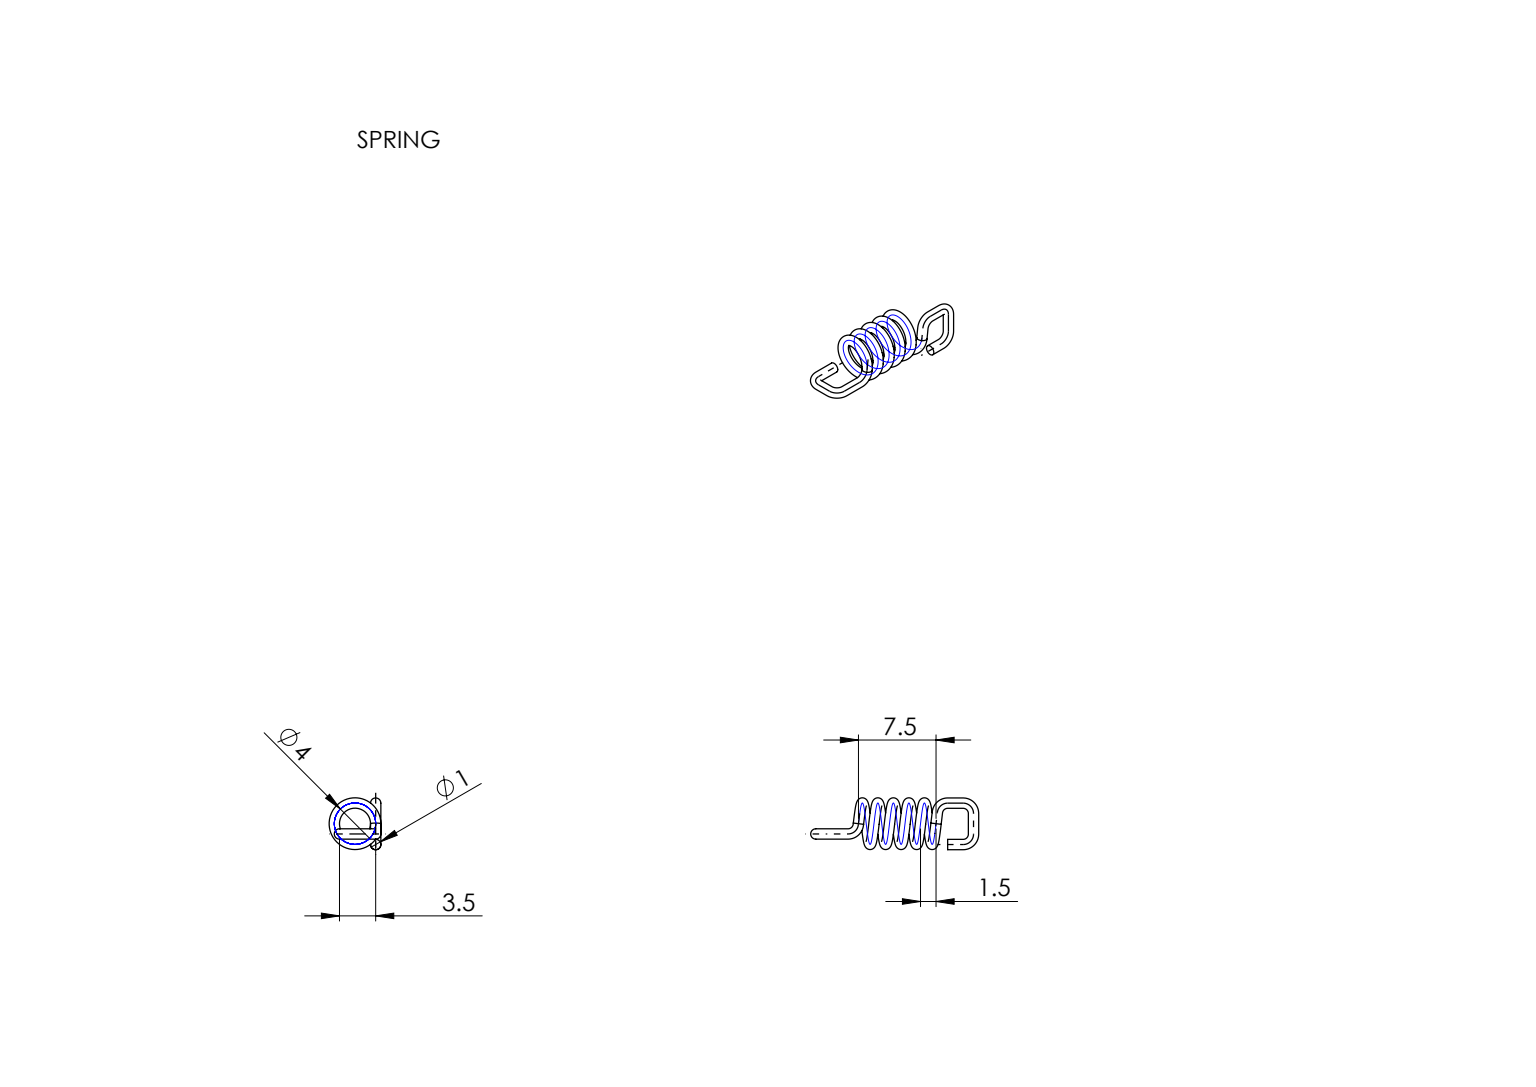
ISO-10303-21;
HEADER;
FILE_DESCRIPTION (('STEP AP214'),
    '1' );
FILE_NAME ('spring.step',
    '2026-09-28T15:49:00',
    ( '' ),
    ( '' ),
    'SwSTEP 2.0',
    'SolidWorks 2026',
    '' );
FILE_SCHEMA (( 'AUTOMOTIVE_DESIGN' ));
ENDSEC;

DATA;
#5=CARTESIAN_POINT ( 'NONE',  ( -34.00000000000000000, -114.0592624029313242, 6.003524454178450043 ) ) ;
#16=CARTESIAN_POINT ( 'NONE',  ( -35.50000000000000000, -112.5389594332240222, 2.818899826424027477 ) ) ;
#20=CARTESIAN_POINT ( 'NONE',  ( -35.50000000000000711, -114.9929510916434339, 11.38636890470581164 ) ) ;
#22=CARTESIAN_POINT ( 'NONE',  ( -34.50000000000000000, -113.9929510916434339, 12.17846912687782712 ) ) ;
#25=CARTESIAN_POINT ( 'NONE',  ( -34.50000000000000000, -113.9929510916434339, 10.68227981832981044 ) ) ;
#26=CARTESIAN_POINT ( 'NONE',  ( -38.99999693208653895, -114.9929510916434339, 12.62875129555797749 ) ) ;
#27=CARTESIAN_POINT ( 'NONE',  ( -35.50000000000000711, -114.9860996047076895, 10.38555023491505835 ) ) ;
#42=CARTESIAN_POINT ( 'NONE',  ( -35.50000000000000000, -113.2441867727860227, 0.9026824934337903672 ) ) ;
#44=CARTESIAN_POINT ( 'NONE',  ( -37.97545270896701908, -113.5265240346955977, 3.847274454178448710 ) ) ;
#51=CARTESIAN_POINT ( 'NONE',  ( -35.50000000000000000, -116.2431927316855109, -2.224114562372550008 ) ) ;
#54=CARTESIAN_POINT ( 'NONE',  ( -39.02454729103295961, -114.7691647218148745, 8.159774454178448266 ) ) ;
#59=CARTESIAN_POINT ( 'NONE',  ( -34.50000000000000000, -113.0140978167136581, -0.6247823525984268489 ) ) ;
#65=CARTESIAN_POINT ( 'NONE',  ( -35.50000000000000000, -113.9929510916434339, 10.61627146648203990 ) ) ;
#70=CARTESIAN_POINT ( 'NONE',  ( -34.50000000000000000, -113.0071371610607684, 2.888584676720006961 ) ) ;
#71=CARTESIAN_POINT ( 'NONE',  ( -39.00000000000000000, -115.9929510916434481, 12.17846912687782179 ) ) ;
#77=CARTESIAN_POINT ( 'NONE',  ( -35.50000000000000711, -114.1414532730574507, 9.517316564499758158 ) ) ;
#95=CARTESIAN_POINT ( 'NONE',  ( -36.64504884055821776, -112.9754527089670688, 6.715225545821551734 ) ) ;
#108=CARTESIAN_POINT ( 'NONE',  ( -35.50000000000000711, -114.0882517521923489, 9.510534276948430232 ) ) ;
#115=CARTESIAN_POINT ( 'NONE',  ( -35.87745010033553683, -115.9929510916434481, 14.11371147303761475 ) ) ;
#124=CARTESIAN_POINT ( 'NONE',  ( -35.62769128460905677, -112.5438815906447729, 6.808975545821550845 ) ) ;
#149=CARTESIAN_POINT ( 'NONE',  ( -34.50000000000000000, -113.4307644833805000, -1.624782352598427959 ) ) ;
#151=CARTESIAN_POINT ( 'NONE',  ( -39.00000000000000711, -114.9929510916434339, 12.60752341388803721 ) ) ;
#152=CARTESIAN_POINT ( 'NONE',  ( -35.50000000000000000, -113.9929510916434339, 10.50625754673586876 ) ) ;
#155=CARTESIAN_POINT ( 'NONE',  ( -36.03125000000004263, -114.9929510916434339, 14.11852480586264846 ) ) ;
#167=CARTESIAN_POINT ( 'NONE',  ( -39.16322519054179452, -116.0794154965774823, 6.566024454178448266 ) ) ;
#174=CARTESIAN_POINT ( 'NONE',  ( -39.07941549657748936, -111.8367748094582055, 6.941024454178450043 ) ) ;
#177=DIRECTION ( 'NONE',  ( -1.000000000000000000, 0.000000000000000000, 0.000000000000000000 ) ) ;
#186=CARTESIAN_POINT ( 'NONE',  ( -35.50000000000000000, -111.8727710936879589, 2.535339294948415922 ) ) ;
#193=CARTESIAN_POINT ( 'NONE',  ( -35.50160444427493189, -114.9929510916434339, 12.65937477241749853 ) ) ;
#194=CARTESIAN_POINT ( 'NONE',  ( -36.03125000000003553, -113.9929510916434339, 14.11852480586265024 ) ) ;
#198=CARTESIAN_POINT ( 'NONE',  ( -34.50000000000000000, -113.9929510916434339, 10.50625754673588474 ) ) ;
#199=CARTESIAN_POINT ( 'NONE',  ( -39.00000000000000711, -114.9929510916434339, 11.21034663311206181 ) ) ;
#200=CARTESIAN_POINT ( 'NONE',  ( -35.50000000000000711, -114.9492820284331742, 10.20776876943783940 ) ) ;
#202=CIRCLE ( 'NONE', #8824, 0.5000000000000004441 ) ;
#213=CARTESIAN_POINT ( 'NONE',  ( -35.50000000000000000, -113.0140978167138712, 0.8127176474015720409 ) ) ;
#215=CARTESIAN_POINT ( 'NONE',  ( -36.11231047232249125, -112.0245472910329880, 5.722274454178448266 ) ) ;
#221=CARTESIAN_POINT ( 'NONE',  ( -35.50000000000000711, -112.8356783780338759, 1.859636627348750348 ) ) ;
#224=CARTESIAN_POINT ( 'NONE',  ( -38.97545270896704039, -113.1123104723225197, 8.347274454178448266 ) ) ;
#228=CARTESIAN_POINT ( 'NONE',  ( -34.50000000000000000, -113.6318576702834804, 1.956056246348823580 ) ) ;
#235=CARTESIAN_POINT ( 'NONE',  ( -35.50000000000000000, -113.9929510916434339, 11.38636890470581164 ) ) ;
#240=CARTESIAN_POINT ( 'NONE',  ( -34.50000000000000000, -111.1014359431343905, 1.472195201997948510 ) ) ;
#242=CARTESIAN_POINT ( 'NONE',  ( -37.51022648969539119, -115.9929510916434481, 14.11852173794918563 ) ) ;
#247=CARTESIAN_POINT ( 'NONE',  ( -37.99999897736217491, -115.9929510916434481, 12.62466071271733092 ) ) ;
#267=CARTESIAN_POINT ( 'NONE',  ( -37.74901162816868805, -113.3347980657955958, 4.933975545821551734 ) ) ;
#276=CARTESIAN_POINT ( 'NONE',  ( -35.50000000000000000, -117.0140978167138854, 0.6252176474015650465 ) ) ;
#287=CARTESIAN_POINT ( 'NONE',  ( -38.81062062679291813, -115.9929510916434481, 13.37409560816442244 ) ) ;
#296=CARTESIAN_POINT ( 'NONE',  ( -37.88768952767750875, -112.0245472910329880, 9.527725545821557063 ) ) ;
#324=CARTESIAN_POINT ( 'NONE',  ( -34.50000000000000000, -115.0795240838853886, -1.623175561345890472 ) ) ;
#325=CARTESIAN_POINT ( 'NONE',  ( -38.99999693208653895, -114.9929510916434339, 12.62875129555797749 ) ) ;
#326=CARTESIAN_POINT ( 'NONE',  ( -35.50000000000000000, -113.9929510916433060, 10.50625754673589540 ) ) ;
#328=CARTESIAN_POINT ( 'NONE',  ( -34.50481333282507279, -114.9929510916434339, 12.74107470552716492 ) ) ;
#337=CARTESIAN_POINT ( 'NONE',  ( -33.97545270896702618, -112.8166217158120475, 5.909774454178450931 ) ) ;
#341=CARTESIAN_POINT ( 'NONE',  ( -35.50000000000000711, -115.6286452741999113, -1.424448457485488095 ) ) ;
#358=CARTESIAN_POINT ( 'NONE',  ( -35.50000000000000000, -112.3070160848889429, 2.749963775944984867 ) ) ;
#361=CARTESIAN_POINT ( 'NONE',  ( -35.83891589277640577, -114.9929510916434339, 13.09299768411358222 ) ) ;
#365=CARTESIAN_POINT ( 'NONE',  ( -34.50000000000000000, -113.9929510916434339, 12.56351784598954424 ) ) ;
#368=CARTESIAN_POINT ( 'NONE',  ( -34.50000000000000000, -113.9929510916434339, 11.21034663311132107 ) ) ;
#371=CARTESIAN_POINT ( 'NONE',  ( -35.50000000000000711, -114.8211182053456838, 9.932864235516914775 ) ) ;
#385=CARTESIAN_POINT ( 'NONE',  ( -35.50000000000000000, -114.5974311500472567, -0.6247823525984269599 ) ) ;
#387=CARTESIAN_POINT ( 'NONE',  ( -39.02454729103295961, -114.7691647218148745, 5.159774454178448266 ) ) ;
#394=CARTESIAN_POINT ( 'NONE',  ( -35.50000000000000711, -112.0140900043112282, 0.8439677466545482121 ) ) ;
#399=CARTESIAN_POINT ( 'NONE',  ( -35.00000000000000000, -114.0592624029313242, 9.003524454178448266 ) ) ;
#401=( NAMED_UNIT ( * ) PLANE_ANGLE_UNIT ( ) SI_UNIT ( $, .RADIAN. ) );
#405=CARTESIAN_POINT ( 'NONE',  ( -34.50000000000000000, -112.7472371723319355, 1.839427296857320648 ) ) ;
#410=CIRCLE ( 'NONE', #8457, 0.5000000000000004441 ) ;
#412=CARTESIAN_POINT ( 'NONE',  ( -35.50000000000000000, -113.9929510916434339, 11.91443571948720148 ) ) ;
#415=CARTESIAN_POINT ( 'NONE',  ( -34.50000000000000000, -115.9821387493194891, -0.8839717462762166633 ) ) ;
#419=CARTESIAN_POINT ( 'NONE',  ( -39.00000206272865455, -115.9929510916434481, 12.61164896875035879 ) ) ;
#446=CARTESIAN_POINT ( 'NONE',  ( -37.05926240293131713, -113.0000000000000000, 3.621475545821551734 ) ) ;
#458=CARTESIAN_POINT ( 'NONE',  ( -35.50000000000000711, -115.6286452741999113, -1.424448457485488095 ) ) ;
#460=CARTESIAN_POINT ( 'NONE',  ( -35.50000000000000711, -114.1264797827112574, 9.515205387299289441 ) ) ;
#464=CARTESIAN_POINT ( 'NONE',  ( -34.50000000000000000, -114.9819937217110635, 10.35556074009299188 ) ) ;
#468=CARTESIAN_POINT ( 'NONE',  ( -36.24999999999983658, -115.9929510916434481, 14.11852480586265024 ) ) ;
#469=CARTESIAN_POINT ( 'NONE',  ( -35.50000000000000711, -112.0140900043366088, -0.5935324770972457697 ) ) ;
#480=CARTESIAN_POINT ( 'NONE',  ( -36.11231047232249125, -115.9754527089670262, 7.277725545821551734 ) ) ;
#507=CARTESIAN_POINT ( 'NONE',  ( -34.50000000000000000, -113.3474311500483935, -0.6247823525984269599 ) ) ;
#510=CARTESIAN_POINT ( 'NONE',  ( -39.00000000000000711, -114.9929510916434339, 11.91443571948719615 ) ) ;
#514=CARTESIAN_POINT ( 'NONE',  ( -34.50000000000000000, -114.9929510916434339, 12.59652202191340642 ) ) ;
#523=CARTESIAN_POINT ( 'NONE',  ( -39.16322519054179452, -116.0794154965774823, 3.566024454178448710 ) ) ;
#526=CARTESIAN_POINT ( 'NONE',  ( -35.50000000000000711, -112.1403507321855528, -1.128496220798856253 ) ) ;
#541=CARTESIAN_POINT ( 'NONE',  ( -35.50000000000000000, -112.9611193698460738, 2.883091707513499635 ) ) ;
#543=CARTESIAN_POINT ( 'NONE',  ( -35.50025087934803736, -114.9929510916434339, 12.63488142334835196 ) ) ;
#547=CARTESIAN_POINT ( 'NONE',  ( -38.98797722933581866, -113.9929510916434339, 12.81430620224974959 ) ) ;
#551=CARTESIAN_POINT ( 'NONE',  ( -34.50300906734826611, -113.9929510916434339, 12.71660600561482468 ) ) ;
#552=CARTESIAN_POINT ( 'NONE',  ( -38.98797722933582577, -114.9929510916434339, 12.81430620224974959 ) ) ;
#553=CARTESIAN_POINT ( 'NONE',  ( -35.50000000000000711, -114.9929510916434339, 10.51175824272318415 ) ) ;
#563=CARTESIAN_POINT ( 'NONE',  ( -35.50000000000000000, -113.0140978167138712, -0.6247823525979733228 ) ) ;
#565=CARTESIAN_POINT ( 'NONE',  ( -35.62769128460905677, -115.4561184093552413, 4.691024454178448266 ) ) ;
#572=CARTESIAN_POINT ( 'NONE',  ( -35.50000000000000711, -112.6605569508015350, 1.812590711673265575 ) ) ;
#575=CARTESIAN_POINT ( 'NONE',  ( -38.37230871539094323, -112.5438815906447729, 5.441024454178449155 ) ) ;
#582=CARTESIAN_POINT ( 'NONE',  ( -34.50000000000000000, -113.0106174888879877, 1.881901162060937827 ) ) ;
#588=CARTESIAN_POINT ( 'NONE',  ( -35.50000000000000000, -113.9929510916434339, 10.50625754673577994 ) ) ;
#592=CARTESIAN_POINT ( 'NONE',  ( -34.50000000000000000, -112.7319952733504635, 2.855726801009121463 ) ) ;
#593=CARTESIAN_POINT ( 'NONE',  ( -37.74437085908086686, -115.9929510916434481, 14.09929883582536903 ) ) ;
#617=CARTESIAN_POINT ( 'NONE',  ( -36.52652403469559061, -114.9754527089670262, 5.777725545821551734 ) ) ;
#629=CARTESIAN_POINT ( 'NONE',  ( -35.50000000000000711, -114.9928438774171582, 10.49113435197128652 ) ) ;
#633=CARTESIAN_POINT ( 'NONE',  ( -34.50000000000000000, -114.9929510916434339, 10.85830208992344303 ) ) ;
#638=CARTESIAN_POINT ( 'NONE',  ( -39.00000000000000000, -115.9929510916434481, 11.73841344789285657 ) ) ;
#639=CARTESIAN_POINT ( 'NONE',  ( -35.50000000000000711, -112.2144317118258527, -1.239329810084414341 ) ) ;
#647=CARTESIAN_POINT ( 'NONE',  ( -36.64504884055821776, -112.9754527089670688, 3.715225545821552178 ) ) ;
#672=CARTESIAN_POINT ( 'NONE',  ( -34.50000000000000000, -115.0140978167138712, -0.6247823525985405357 ) ) ;
#675=CARTESIAN_POINT ( 'NONE',  ( -39.00000000000000711, -114.9929510916434339, 12.39849696637031151 ) ) ;
#679=CARTESIAN_POINT ( 'NONE',  ( -34.50000000000000000, -114.2600084737790809, 8.524153227862690585 ) ) ;
#689=CARTESIAN_POINT ( 'NONE',  ( -38.30190309005061522, -116.9754527089670546, 7.972274454178450043 ) ) ;
#691=CARTESIAN_POINT ( 'NONE',  ( -35.50000000000000711, -112.9486715495423681, -1.623175561345890472 ) ) ;
#704=CARTESIAN_POINT ( 'NONE',  ( -36.23083527818513261, -111.9754527089670404, 5.215225545821551734 ) ) ;
#710=CARTESIAN_POINT ( 'NONE',  ( -35.50000000000000000, -112.4803765279500993, 2.803636946313094569 ) ) ;
#715=CARTESIAN_POINT ( 'NONE',  ( -37.37500000000009237, -114.9929510916434339, 13.11852480586264669 ) ) ;
#717=CARTESIAN_POINT ( 'NONE',  ( -37.54906985245723661, -113.9929510916434339, 14.11777216781844757 ) ) ;
#722=CARTESIAN_POINT ( 'NONE',  ( -36.12500000000014211, -113.9929510916434339, 14.11852480586265024 ) ) ;
#725=CARTESIAN_POINT ( 'NONE',  ( -35.50040135968785648, -114.9929510916434339, 12.63896776382214071 ) ) ;
#730=ORIENTED_EDGE ( 'NONE', *, *, #15666, .T. ) ;
#738=CARTESIAN_POINT ( 'NONE',  ( -35.50000000000000000, -115.0140978167134165, -0.6247823525984399495 ) ) ;
#740=CARTESIAN_POINT ( 'NONE',  ( -38.02454729103296671, -114.3549511594417396, 8.159774454178448266 ) ) ;
#742=CARTESIAN_POINT ( 'NONE',  ( -36.11231047232249125, -112.0245472910329880, 7.222274454178451819 ) ) ;
#748=CARTESIAN_POINT ( 'NONE',  ( -35.50000000000000000, -116.0215255531121983, -2.372276521655488857 ) ) ;
#752=CARTESIAN_POINT ( 'NONE',  ( -36.11231047232249125, -112.0245472910329880, 5.722274454178448266 ) ) ;
#757=CARTESIAN_POINT ( 'NONE',  ( -34.50000000000000000, -112.0414288467712112, 1.115164475686276191 ) ) ;
#766=CARTESIAN_POINT ( 'NONE',  ( -37.18750000000004974, -113.9929510916434339, 13.11852480586264846 ) ) ;
#769=CARTESIAN_POINT ( 'NONE',  ( -34.50000000000000000, -111.0140978167138570, 0.5627176474015715968 ) ) ;
#770=CARTESIAN_POINT ( 'NONE',  ( -39.00000000000000000, -115.9929510916434481, 12.57451923796417681 ) ) ;
#794=CARTESIAN_POINT ( 'NONE',  ( -36.52652403469559061, -114.9754527089670262, 7.277725545821552622 ) ) ;
#801=CARTESIAN_POINT ( 'NONE',  ( -35.50000000000000711, -115.2732872103912030, -1.592823285204062911 ) ) ;
#803=CARTESIAN_POINT ( 'NONE',  ( -35.50000000000000711, -114.9929510916434339, 12.59652202191340642 ) ) ;
#807=CARTESIAN_POINT ( 'NONE',  ( -34.50000000000000000, -114.9929510916434339, 10.55026311463432087 ) ) ;
#811=CARTESIAN_POINT ( 'NONE',  ( -39.00000000000000000, -115.9929510916434481, 12.26648026267477221 ) ) ;
#812=CARTESIAN_POINT ( 'NONE',  ( -35.50000000000000711, -112.0414288467712112, 1.115164475686276191 ) ) ;
#821=CARTESIAN_POINT ( 'NONE',  ( -36.64504884055823908, -115.0245472910329880, 1.784774454178449155 ) ) ;
#832=CARTESIAN_POINT ( 'NONE',  ( -37.05926240293131713, -111.0000000000000284, 5.121475545821551734 ) ) ;
#848=CARTESIAN_POINT ( 'NONE',  ( -34.50000000000000000, -115.0140978167139707, -0.6247823525984387283 ) ) ;
#852=CARTESIAN_POINT ( 'NONE',  ( -39.00000000000000711, -114.9929510916434339, 11.73841344789285657 ) ) ;
#854=CARTESIAN_POINT ( 'NONE',  ( -36.23083527818513261, -116.0245472910329880, 1.784774454178448710 ) ) ;
#855=CARTESIAN_POINT ( 'NONE',  ( -39.00000000000000711, -114.9929510916434339, 11.91443571948719615 ) ) ;
#858=DIRECTION ( 'NONE',  ( 0.000000000000000000, 0.000000000000000000, -1.000000000000000000 ) ) ;
#865=CARTESIAN_POINT ( 'NONE',  ( -35.81662171581203324, -110.9754527089670546, 3.715225545821552178 ) ) ;
#867=CARTESIAN_POINT ( 'NONE',  ( -35.50000000000000711, -112.8511839106603247, -1.611965039240275122 ) ) ;
#885=CARTESIAN_POINT ( 'NONE',  ( -39.02454729103295961, -113.2308352781851397, 6.340225545821550845 ) ) ;
#893=CARTESIAN_POINT ( 'NONE',  ( -35.50000000000000000, -113.2224311500466030, -2.624782352598442614 ) ) ;
#896=CARTESIAN_POINT ( 'NONE',  ( -35.74814306589956914, -114.9929510916434339, 13.05539834812772781 ) ) ;
#897=CARTESIAN_POINT ( 'NONE',  ( -39.00000206272865455, -113.9929510916434339, 12.61164896875035879 ) ) ;
#901=CARTESIAN_POINT ( 'NONE',  ( -35.80421860361284558, -113.9929510916434339, 14.10650203519841916 ) ) ;
#906=CARTESIAN_POINT ( 'NONE',  ( -35.96730626674924025, -114.9929510916434339, 13.11752178341330044 ) ) ;
#913=CARTESIAN_POINT ( 'NONE',  ( -35.74814306589956914, -114.9929510916434339, 13.05539834812772781 ) ) ;
#922=CARTESIAN_POINT ( 'NONE',  ( -35.50000000000000000, -113.0140978167156902, -0.6247823525984268489 ) ) ;
#924=CARTESIAN_POINT ( 'NONE',  ( -35.97545270896702618, -113.6450488405582604, 8.909774454178450043 ) ) ;
#928=CARTESIAN_POINT ( 'NONE',  ( -38.97545270896704039, -113.1123104723225197, 6.847274454178450931 ) ) ;
#931=CARTESIAN_POINT ( 'NONE',  ( -35.50000000000000711, -112.0221129971568104, -0.7553032835231431319 ) ) ;
#942=CARTESIAN_POINT ( 'NONE',  ( -34.50000000000000000, -112.9185811467682754, 1.870920967077121411 ) ) ;
#950=CARTESIAN_POINT ( 'NONE',  ( -35.93473953453761993, -113.9929510916434339, 13.11451721564123396 ) ) ;
#953=CARTESIAN_POINT ( 'NONE',  ( -35.69272627125608466, -113.9929510916434339, 13.01835785830562209 ) ) ;
#955=CARTESIAN_POINT ( 'NONE',  ( -35.50000000000000000, -115.9929510916434481, 10.94631322572069365 ) ) ;
#986=CARTESIAN_POINT ( 'NONE',  ( -37.74901162816868805, -113.3347980657955958, 9.433975545821549957 ) ) ;
#998=CARTESIAN_POINT ( 'NONE',  ( -35.95915003344517658, -114.9929510916434339, 13.11692036158763308 ) ) ;
#1003=CARTESIAN_POINT ( 'NONE',  ( -34.50000000000000000, -114.0998638248492085, 9.511920366020609308 ) ) ;
#1009=CARTESIAN_POINT ( 'NONE',  ( -35.50000000000000000, -115.9929081983957104, 10.49113315946066294 ) ) ;
#1010=CARTESIAN_POINT ( 'NONE',  ( -35.50000000000000711, -113.6318576702834804, 1.956056246348823580 ) ) ;
#1021=CARTESIAN_POINT ( 'NONE',  ( -37.66520193420439711, -114.7490116281687023, 6.058975545821550845 ) ) ;
#1031=CARTESIAN_POINT ( 'NONE',  ( -36.94073759706866156, -111.0000000000000284, 7.128524454178450043 ) ) ;
#1048=CARTESIAN_POINT ( 'NONE',  ( -34.50000000000000000, -115.0140978167138712, -0.4685323525984310122 ) ) ;
#1052=CARTESIAN_POINT ( 'NONE',  ( -34.50000000000000000, -114.3793648455349654, 8.543708532059524074 ) ) ;
#1055=CARTESIAN_POINT ( 'NONE',  ( -38.99879592093640923, -114.9929510916434339, 12.67985367974111455 ) ) ;
#1065=CARTESIAN_POINT ( 'NONE',  ( -39.16322519054178741, -111.9205845034225177, 3.433975545821550845 ) ) ;
#1067=CARTESIAN_POINT ( 'NONE',  ( -35.50000000000000711, -116.0140978167138712, -0.4685323525984310677 ) ) ;
#1079=CARTESIAN_POINT ( 'NONE',  ( -37.76916472181486739, -116.0245472910329880, 5.965225545821551734 ) ) ;
#1083=CARTESIAN_POINT ( 'NONE',  ( -35.50000000000000000, -114.8057644833805853, -2.624782352598442614 ) ) ;
#1088=CARTESIAN_POINT ( 'NONE',  ( -37.59808119975203766, -113.9929510916434339, 14.11551573851449071 ) ) ;
#1093=CARTESIAN_POINT ( 'NONE',  ( -37.46874999999995737, -113.9929510916434339, 14.11852480586265024 ) ) ;
#1095=CARTESIAN_POINT ( 'NONE',  ( -36.03906250000000000, -114.9929510916434339, 13.11852480586264669 ) ) ;
#1102=CARTESIAN_POINT ( 'NONE',  ( -35.50000000000000711, -114.9929510916434339, 11.38636890470581164 ) ) ;
#1105=CARTESIAN_POINT ( 'NONE',  ( -37.88768952767750164, -115.9754527089670262, 1.972274454178448710 ) ) ;
#1110=CARTESIAN_POINT ( 'NONE',  ( -35.50000000000000000, -113.0140978167138996, -0.6247823525984306237 ) ) ;
#1114=CARTESIAN_POINT ( 'NONE',  ( -37.88768952767750164, -115.9754527089670262, 1.972274454178448710 ) ) ;
#1116=CARTESIAN_POINT ( 'NONE',  ( -35.50000000000000711, -115.0795240838853886, -1.623175561345890472 ) ) ;
#1127=CARTESIAN_POINT ( 'NONE',  ( -34.50000000000000000, -116.0140978167138712, -0.4685323525984310677 ) ) ;
#1134=CARTESIAN_POINT ( 'NONE',  ( -37.50613590685470911, -113.9929510916434339, 13.11852378322482515 ) ) ;
#1139=CARTESIAN_POINT ( 'NONE',  ( -35.50000000000000000, -113.9929510916434339, 11.91443571948720148 ) ) ;
#1140=CARTESIAN_POINT ( 'NONE',  ( -35.50000000000000000, -115.9929510916434481, 10.72628538622835670 ) ) ;
#1158=CARTESIAN_POINT ( 'NONE',  ( -34.50000000000000000, -115.2751396785629510, -2.608751991713152307 ) ) ;
#1159=DIRECTION ( 'NONE',  ( -1.000000000000000000, 0.000000000000000000, 0.000000000000000000 ) ) ;
#1162=CARTESIAN_POINT ( 'NONE',  ( -37.99999999999998579, -113.9407375970686758, 3.753524454178448710 ) ) ;
#1168=CARTESIAN_POINT ( 'NONE',  ( -34.50000000000000000, -113.0140978167142833, 0.8752176474019800478 ) ) ;
#1174=CARTESIAN_POINT ( 'NONE',  ( -35.50400759022159036, -114.9929510916434339, 12.68378527132497524 ) ) ;
#1181=CARTESIAN_POINT ( 'NONE',  ( -34.50000000000000000, -114.9929510916434339, 10.94631322572069365 ) ) ;
#1186=CARTESIAN_POINT ( 'NONE',  ( -35.50000000000000000, -115.9874658933321001, 10.35517832894335832 ) ) ;
#1187=CARTESIAN_POINT ( 'NONE',  ( -35.50000000000000711, -112.1222502514821144, 1.343475657184566296 ) ) ;
#1196=CARTESIAN_POINT ( 'NONE',  ( -36.94073759706868287, -115.0000000000000000, 7.371475545821551734 ) ) ;
#1203=CARTESIAN_POINT ( 'NONE',  ( -33.97545270896703329, -115.1833782841879810, 5.590225545821552622 ) ) ;
#1222=CARTESIAN_POINT ( 'NONE',  ( -34.50000000000000000, -113.2224311500466030, -0.6247823525984269599 ) ) ;
#1225=CARTESIAN_POINT ( 'NONE',  ( -34.50000000000000000, -114.1556834383649459, 8.511484393387789282 ) ) ;
#1227=CARTESIAN_POINT ( 'NONE',  ( -38.97545270896704039, -113.1123104723225055, 2.347274454178448710 ) ) ;
#1230=CARTESIAN_POINT ( 'NONE',  ( -34.50000000000000000, -114.1371041221139109, 8.509266650872710613 ) ) ;
#1238=CARTESIAN_POINT ( 'NONE',  ( -34.00000000000000000, -113.9407375970686758, 5.496475545821551734 ) ) ;
#1240=CARTESIAN_POINT ( 'NONE',  ( -35.50000000000000000, -113.3822401464312719, 0.9191614010536472978 ) ) ;
#1248=CARTESIAN_POINT ( 'NONE',  ( -34.97545270896703329, -114.7691647218148745, 2.590225545821551290 ) ) ;
#1253=CARTESIAN_POINT ( 'NONE',  ( -35.50000000000000000, -115.2751396785629510, -2.608751991713152307 ) ) ;
#1257=CARTESIAN_POINT ( 'NONE',  ( -37.99999897736218202, -114.9929510916434339, 12.62466071271732915 ) ) ;
#1259=CARTESIAN_POINT ( 'NONE',  ( -34.50000000000000000, -114.1021862393805577, 9.512197583835053649 ) ) ;
#1262=CARTESIAN_POINT ( 'NONE',  ( -38.99924736195577424, -113.9929510916434339, 12.66759465831984599 ) ) ;
#1264=CARTESIAN_POINT ( 'NONE',  ( -36.24999999999983658, -114.9929510916434339, 13.11852480586264669 ) ) ;
#1270=CARTESIAN_POINT ( 'NONE',  ( -35.50000000000000711, -114.9925223117477202, 10.47601618151863079 ) ) ;
#1278=CARTESIAN_POINT ( 'NONE',  ( -34.50000000000000000, -113.0140978167138712, 0.8752176474016720720 ) ) ;
#1280=CARTESIAN_POINT ( 'NONE',  ( -38.45611840935523418, -115.3723087153909432, 8.066024454178448266 ) ) ;
#1282=CARTESIAN_POINT ( 'NONE',  ( -37.76916472181487450, -111.9754527089670404, 2.534774454178448710 ) ) ;
#1286=CARTESIAN_POINT ( 'NONE',  ( -35.50000000000000711, -113.0557643173828524, -1.624792769101735868 ) ) ;
#1295=CARTESIAN_POINT ( 'NONE',  ( -34.50000000000000000, -112.3995503592287690, -1.424448457485529618 ) ) ;
#1298=ADVANCED_FACE ( 'NONE', ( #6669 ), #9134, .T. ) ;
#1303=CARTESIAN_POINT ( 'NONE',  ( -37.99359134332094357, -113.9929510916434339, 12.69998175888958514 ) ) ;
#1305=CARTESIAN_POINT ( 'NONE',  ( -36.03906250000000000, -113.9929510916434339, 13.11852480586264846 ) ) ;
#1306=CARTESIAN_POINT ( 'NONE',  ( -35.50005019975638021, -115.9929510916434481, 12.62670525340498351 ) ) ;
#1321=CARTESIAN_POINT ( 'NONE',  ( -35.50000000000000711, -113.8159288351371714, 1.978028123174813802 ) ) ;
#1324=CARTESIAN_POINT ( 'NONE',  ( -35.50000000000000711, -114.1152303497977414, 9.513755561829650986 ) ) ;
#1326=ORIENTED_EDGE ( 'NONE', *, *, #32143, .T. ) ;
#1329=CARTESIAN_POINT ( 'NONE',  ( -34.50000000000000000, -113.6807644833805995, -2.624782352598442614 ) ) ;
#1334=CARTESIAN_POINT ( 'NONE',  ( -36.64504884055823908, -115.0245472910329880, 1.784774454178449155 ) ) ;
#1340=CARTESIAN_POINT ( 'NONE',  ( -35.50000000000000000, -113.8474311500459777, -0.6247823525984269599 ) ) ;
#1348=CARTESIAN_POINT ( 'NONE',  ( -35.49999931242378892, -114.9929510916434339, 12.61439929482945566 ) ) ;
#1351=CARTESIAN_POINT ( 'NONE',  ( -34.50120407906360498, -114.9929510916434339, 12.67985367974112343 ) ) ;
#1356=CARTESIAN_POINT ( 'NONE',  ( -35.50000000000000000, -115.9929510916434481, 11.73841344789270202 ) ) ;
#1357=CARTESIAN_POINT ( 'NONE',  ( -35.50000000000000711, -115.1446187476384040, -1.616767172155725740 ) ) ;
#1370=CARTESIAN_POINT ( 'NONE',  ( -36.52652403469559061, -114.9754527089670262, 5.777725545821551734 ) ) ;
#1376=DIRECTION ( 'NONE',  ( 0.000000000000000000, -0.9929510916431035783, 0.1185248058626076212 ) ) ;
#1379=CARTESIAN_POINT ( 'NONE',  ( -38.30190309005061522, -111.0245472910330022, 9.527725545821551734 ) ) ;
#1390=CARTESIAN_POINT ( 'NONE',  ( -35.50000000000000711, -114.0000000000000853, 2.000000000000001776 ) ) ;
#1394=CARTESIAN_POINT ( 'NONE',  ( -34.50000000000000000, -112.4434344552011282, 1.705278471174987986 ) ) ;
#1399=CARTESIAN_POINT ( 'NONE',  ( -37.48437500000004263, -115.9929510916434481, 14.11852480586265024 ) ) ;
#1403=CARTESIAN_POINT ( 'NONE',  ( -39.00000000000000711, -114.9929510916434339, 12.57451923796417503 ) ) ;
#1413=CARTESIAN_POINT ( 'NONE',  ( -40.02454729103296671, -112.8166217158120332, 6.340225545821551734 ) ) ;
#1415=CARTESIAN_POINT ( 'NONE',  ( -35.50000000000000000, -113.0140978167136581, -0.6247823525984268489 ) ) ;
#1427=CARTESIAN_POINT ( 'NONE',  ( -35.54388159064475872, -115.3723087153909432, 7.183975545821551734 ) ) ;
#1432=CARTESIAN_POINT ( 'NONE',  ( -35.50000000000000000, -117.0140978167138854, -0.4685323525984309012 ) ) ;
#1436=CARTESIAN_POINT ( 'NONE',  ( -38.00000000000000711, -114.9929510916434339, 12.57451923796417503 ) ) ;
#1438=CARTESIAN_POINT ( 'NONE',  ( -34.50000000000000000, -114.9929510916434339, 10.94631322572069365 ) ) ;
#1440=CARTESIAN_POINT ( 'NONE',  ( -37.18750000000006395, -114.9929510916434339, 13.11852480586264669 ) ) ;
#1442=CARTESIAN_POINT ( 'NONE',  ( -35.98977351030467986, -113.9929510916434339, 14.11852173794918563 ) ) ;
#1444=CARTESIAN_POINT ( 'NONE',  ( -36.00585935943767169, -114.9929510916434339, 13.11852578240983291 ) ) ;
#1453=CARTESIAN_POINT ( 'NONE',  ( -35.52552712174884419, -114.9929510916434339, 12.77960891308624447 ) ) ;
#1455=CARTESIAN_POINT ( 'NONE',  ( -36.94073759706868287, -112.0000000000000142, 2.628524454178448710 ) ) ;
#1460=CARTESIAN_POINT ( 'NONE',  ( -34.50000000000000000, -113.0140978167138712, -0.4685323525984296800 ) ) ;
#1462=CARTESIAN_POINT ( 'NONE',  ( -38.37230871539094323, -112.5438815906447729, 6.941024454178449155 ) ) ;
#1464=CARTESIAN_POINT ( 'NONE',  ( -38.99999999999999289, -113.9407375970686900, 6.753524454178448266 ) ) ;
#1467=CARTESIAN_POINT ( 'NONE',  ( -35.50000000000000711, -112.9813730236132585, -1.624774171495860786 ) ) ;
#1474=CARTESIAN_POINT ( 'NONE',  ( -34.50000000000000000, -112.0460568841087223, -0.8839717462762063382 ) ) ;
#1484=CARTESIAN_POINT ( 'NONE',  ( -35.69272627125608466, -113.9929510916434339, 13.01835785830562209 ) ) ;
#1486=CARTESIAN_POINT ( 'NONE',  ( -36.01562499999997158, -113.9929510916434339, 13.11852480586264846 ) ) ;
#1487=CARTESIAN_POINT ( 'NONE',  ( -35.50000000000000000, -115.9929510916434481, 10.55026311463432087 ) ) ;
#1499=CARTESIAN_POINT ( 'NONE',  ( -35.50000000000000711, -112.0140978167138712, 0.7502176474015694874 ) ) ;
#1510=CARTESIAN_POINT ( 'NONE',  ( -34.50000000000000000, -115.0631849411758196, -2.624765990393648885 ) ) ;
#1514=CARTESIAN_POINT ( 'NONE',  ( -38.02454729103295961, -113.6450488405582462, 9.340225545821551734 ) ) ;
#1519=CARTESIAN_POINT ( 'NONE',  ( -35.50000000000000000, -114.9932644833805426, -0.6247823525982824089 ) ) ;
#1525=CARTESIAN_POINT ( 'NONE',  ( -35.93473953453761283, -114.9929510916434339, 13.11451721564123574 ) ) ;
#1527=CARTESIAN_POINT ( 'NONE',  ( -34.50000306791346816, -114.9929510916434339, 12.62875129555796150 ) ) ;
#1535=CARTESIAN_POINT ( 'NONE',  ( -35.50000102263781798, -115.9929510916434481, 12.62466071271731494 ) ) ;
#1536=CARTESIAN_POINT ( 'NONE',  ( -35.50000000000000711, -116.0141056290913610, -0.5935324770972248976 ) ) ;
#1548=CARTESIAN_POINT ( 'NONE',  ( -37.97545270896702618, -114.4734759653044023, 7.652725545821552622 ) ) ;
#1559=CARTESIAN_POINT ( 'NONE',  ( -35.54388159064475872, -115.3723087153909432, 2.683975545821551290 ) ) ;
#1580=CARTESIAN_POINT ( 'NONE',  ( -34.50000000000000000, -115.9929510916434481, 12.59102132592610346 ) ) ;
#1585=CARTESIAN_POINT ( 'NONE',  ( -36.94073759706868287, -112.0000000000000142, 2.628524454178448710 ) ) ;
#1587=CARTESIAN_POINT ( 'NONE',  ( -34.50000000000000000, -115.9929510916434481, 12.44250253426871033 ) ) ;
#1597=CARTESIAN_POINT ( 'NONE',  ( -35.81662171581203324, -110.9754527089670546, 6.715225545821551734 ) ) ;
#1600=CARTESIAN_POINT ( 'NONE',  ( -35.50000000000000000, -113.0140978167139991, 0.8752176474014555785 ) ) ;
#1618=CARTESIAN_POINT ( 'NONE',  ( -35.50000000000000000, -114.8474311500471572, -2.624782352598442614 ) ) ;
#1624=CARTESIAN_POINT ( 'NONE',  ( -37.97447287825094975, -114.9929510916434339, 12.77960891308616809 ) ) ;
#1625=CARTESIAN_POINT ( 'NONE',  ( -34.50000000000000000, -114.9929510916434339, 10.61627146648203812 ) ) ;
#1628=CARTESIAN_POINT ( 'NONE',  ( -36.15625000000007816, -114.9929510916434339, 13.11852480586264669 ) ) ;
#1631=CARTESIAN_POINT ( 'NONE',  ( -34.50000000000000000, -114.2598117360253696, 9.542047897280109936 ) ) ;
#1639=CARTESIAN_POINT ( 'NONE',  ( -35.50100302244946704, -114.9929510916434339, 12.65121853911337269 ) ) ;
#1642=CARTESIAN_POINT ( 'NONE',  ( -39.02454729103295961, -114.7691647218148745, 2.159774454178448710 ) ) ;
#1648=CARTESIAN_POINT ( 'NONE',  ( -34.50000000000000000, -113.0140978167138996, -0.6247823525984306237 ) ) ;
#1650=CARTESIAN_POINT ( 'NONE',  ( -36.94073759706868287, -112.0000000000000142, 7.128524454178449155 ) ) ;
#1653=CARTESIAN_POINT ( 'NONE',  ( -34.00000000000000000, -114.0592624029313242, 3.003524454178448710 ) ) ;
#1655=CARTESIAN_POINT ( 'NONE',  ( -35.50000000000000711, -112.2144317118258527, -1.239329810084414341 ) ) ;
#1663=CARTESIAN_POINT ( 'NONE',  ( -34.50000000000000000, -115.8137639216009234, -1.239329810084483841 ) ) ;
#1673=CARTESIAN_POINT ( 'NONE',  ( -34.50000000000000000, -113.9000545103886850, 10.49516883415891577 ) ) ;
#1675=CARTESIAN_POINT ( 'NONE',  ( -35.50000000000000000, -113.9929510916434339, 12.44250253426871033 ) ) ;
#1676=CARTESIAN_POINT ( 'NONE',  ( -37.53269373325071712, -115.9929510916434481, 13.11752178341324360 ) ) ;
#1685=CARTESIAN_POINT ( 'NONE',  ( -35.50000000000000711, -112.6605569508015350, 1.812590711673265575 ) ) ;
#1694=CARTESIAN_POINT ( 'NONE',  ( -34.50000000000000000, -116.0215255531121983, -2.372276521655488857 ) ) ;
#1698=CARTESIAN_POINT ( 'NONE',  ( -37.66520193420439000, -113.2509883718312977, 3.941024454178448710 ) ) ;
#1702=CARTESIAN_POINT ( 'NONE',  ( -35.50000000000000000, -115.0140978167139707, -0.6091573525984161908 ) ) ;
#1706=CARTESIAN_POINT ( 'NONE',  ( -37.93687354226506869, -114.9929510916434339, 12.87038173996323565 ) ) ;
#1709=CARTESIAN_POINT ( 'NONE',  ( -37.54906985245724371, -114.9929510916434339, 14.11777216781844579 ) ) ;
#1716=CARTESIAN_POINT ( 'NONE',  ( -35.98364338251434447, -115.9929510916434481, 13.11827392651456314 ) ) ;
#1717=CARTESIAN_POINT ( 'NONE',  ( -35.50000000000000711, -116.0140978167138712, 0.8752176474015622709 ) ) ;
#1728=CARTESIAN_POINT ( 'NONE',  ( -37.05926240293133134, -115.0000000000000000, 6.378524454178448266 ) ) ;
#1737=CARTESIAN_POINT ( 'NONE',  ( -38.37230871539094323, -115.4561184093552413, 3.058975545821551290 ) ) ;
#1758=CARTESIAN_POINT ( 'NONE',  ( -36.03125000000003553, -115.9929510916434481, 14.11852480586265024 ) ) ;
#1761=CARTESIAN_POINT ( 'NONE',  ( -35.00000000000000000, -114.0592624029313242, 7.503524454178449155 ) ) ;
#1762=CARTESIAN_POINT ( 'NONE',  ( -34.50000000000000000, -115.9929510916434481, 12.17846912687782712 ) ) ;
#1774=CARTESIAN_POINT ( 'NONE',  ( -34.00000000000000000, -113.9407375970686758, 9.996475545821549957 ) ) ;
#1778=CARTESIAN_POINT ( 'NONE',  ( -35.50000000000000000, -113.0140978167138712, -0.4685323525984296800 ) ) ;
#1797=CARTESIAN_POINT ( 'NONE',  ( -35.50000000000000711, -113.0974311500471714, -1.624782352598427959 ) ) ;
#1806=CARTESIAN_POINT ( 'NONE',  ( -34.50000000000000000, -112.1859307030124739, 1.448610958621386224 ) ) ;
#1807=CARTESIAN_POINT ( 'NONE',  ( -34.57658136524562309, -114.9929510916434339, 13.10177712753338497 ) ) ;
#1809=CARTESIAN_POINT ( 'NONE',  ( -37.52044295795950291, -114.9929510916434339, 13.11812344617477244 ) ) ;
#1811=CARTESIAN_POINT ( 'NONE',  ( -34.50000000000000000, -114.4026847875275337, 9.592046023459676718 ) ) ;
#1813=CARTESIAN_POINT ( 'NONE',  ( -38.00000000000000711, -114.9929510916434339, 10.85830208992306822 ) ) ;
#1819=CARTESIAN_POINT ( 'NONE',  ( -37.98402046630260287, -114.9929510916434339, 12.74811950270164118 ) ) ;
#1822=CARTESIAN_POINT ( 'NONE',  ( -39.02454729103295961, -114.7691647218148745, 3.659774454178448710 ) ) ;
#1828=CARTESIAN_POINT ( 'NONE',  ( -34.50000000000000000, -113.0140978167139991, 0.8752176474014555785 ) ) ;
#1836=CARTESIAN_POINT ( 'NONE',  ( -34.00000000000000000, -114.0592624029313242, 1.503524454178448710 ) ) ;
#1848=CARTESIAN_POINT ( 'NONE',  ( -34.50000000000000000, -114.8057644833805853, -2.624782352598442614 ) ) ;
#1854=CARTESIAN_POINT ( 'NONE',  ( -34.50000000000000000, -113.9929510916434339, 10.50625754673588474 ) ) ;
#1859=CARTESIAN_POINT ( 'NONE',  ( -38.00000000000000711, -113.9929510916434339, 12.26648026267477221 ) ) ;
#1860=CARTESIAN_POINT ( 'NONE',  ( -36.01562499999997158, -115.9929510916434481, 13.11852480586264846 ) ) ;
#1872=CARTESIAN_POINT ( 'NONE',  ( -35.50000000000000711, -112.0154707866092707, 0.9357013553229778235 ) ) ;
#1878=CARTESIAN_POINT ( 'NONE',  ( -34.50000000000000000, -111.0173113992184710, -0.7556348869410824953 ) ) ;
#1884=CARTESIAN_POINT ( 'NONE',  ( -35.02454729103298803, -114.8876895276775087, 1.597274454178448710 ) ) ;
#1892=CARTESIAN_POINT ( 'NONE',  ( -35.50000000000000000, -115.0140978167138712, -0.4685323525984309012 ) ) ;
#1896=CARTESIAN_POINT ( 'NONE',  ( -35.50000000000000000, -113.9836614335179377, 10.50514867547815534 ) ) ;
#1898=CARTESIAN_POINT ( 'NONE',  ( -36.31249999999995026, -114.9929510916434339, 14.11852480586264846 ) ) ;
#1904=CARTESIAN_POINT ( 'NONE',  ( -35.50005019975638021, -115.9929510916434481, 12.62670525340498351 ) ) ;
#1905=CARTESIAN_POINT ( 'NONE',  ( -35.50000000000000711, -114.8057644833805568, -1.624782352598427959 ) ) ;
#1916=CARTESIAN_POINT ( 'NONE',  ( -37.99999999999998579, -113.9407375970686758, 5.253524454178449155 ) ) ;
#1925=CARTESIAN_POINT ( 'NONE',  ( -36.94073759706868287, -116.9999999999999858, 7.371475545821551734 ) ) ;
#1943=CARTESIAN_POINT ( 'NONE',  ( -35.95093014754292682, -115.9929510916434481, 14.11777216781842625 ) ) ;
#1945=CARTESIAN_POINT ( 'NONE',  ( -39.02454729103295961, -114.7691647218148745, 8.159774454178448266 ) ) ;
#1946=CARTESIAN_POINT ( 'NONE',  ( -34.50000000000000000, -114.8124184834118324, 8.677834500183694288 ) ) ;
#1955=CARTESIAN_POINT ( 'NONE',  ( -38.37230871539094323, -115.4561184093552413, 4.558975545821550845 ) ) ;
#1957=CARTESIAN_POINT ( 'NONE',  ( -35.50000000000000000, -113.0140978167138712, 0.6252176474015680441 ) ) ;
#1969=CARTESIAN_POINT ( 'NONE',  ( -34.97545270896703329, -114.7691647218148745, 8.590225545821551734 ) ) ;
#1974=CARTESIAN_POINT ( 'NONE',  ( -35.50000000000000711, -112.0577668799241309, 1.173706424699810569 ) ) ;
#1983=CARTESIAN_POINT ( 'NONE',  ( -34.50000000000000000, -114.9929510916434339, 10.52000928670414126 ) ) ;
#1985=CARTESIAN_POINT ( 'NONE',  ( -37.58145695302688694, -114.9929510916434339, 13.11211614918362756 ) ) ;
#1987=CARTESIAN_POINT ( 'NONE',  ( -34.50000000000000000, -114.1302255537607095, 9.515717283514957714 ) ) ;
#1998=CARTESIAN_POINT ( 'NONE',  ( -37.48437500000004263, -114.9929510916434339, 13.11852480586264669 ) ) ;
#2001=CARTESIAN_POINT ( 'NONE',  ( -38.45611840935523418, -115.3723087153909432, 6.566024454178448266 ) ) ;
#2011=CARTESIAN_POINT ( 'NONE',  ( -34.02454729103298092, -115.3019030900506294, 4.597274454178449155 ) ) ;
#2024=CARTESIAN_POINT ( 'NONE',  ( -34.50000000000000000, -111.0140978167138570, 0.5627176474015715968 ) ) ;
#2028=CARTESIAN_POINT ( 'NONE',  ( -35.50000000000000711, -114.0650276068786582, 9.507762098804159123 ) ) ;
#2031=CARTESIAN_POINT ( 'NONE',  ( -34.50000000000000000, -113.9929510916434339, 10.50625754673586876 ) ) ;
#2036=CARTESIAN_POINT ( 'NONE',  ( -34.50000000000000000, -113.9743717753924699, 10.50403980422039396 ) ) ;
#2038=CARTESIAN_POINT ( 'NONE',  ( -37.98402046630260287, -115.9929510916434481, 12.74811950270164296 ) ) ;
#2052=CARTESIAN_POINT ( 'NONE',  ( -35.50000000000000711, -112.0140900043366088, -0.5935324770972457697 ) ) ;
#2054=CARTESIAN_POINT ( 'NONE',  ( -35.50000000000000711, -114.4026847875275337, 9.592046023459676718 ) ) ;
#2059=CARTESIAN_POINT ( 'NONE',  ( -35.50000000000000000, -113.3474311500483935, -2.624782352598442614 ) ) ;
#2063=CARTESIAN_POINT ( 'NONE',  ( -36.25098837183129774, -113.3347980657956242, 5.816024454178450043 ) ) ;
#2070=CARTESIAN_POINT ( 'NONE',  ( -34.50000000000000000, -113.0140978167138712, -0.6247823525988807081 ) ) ;
#2076=CARTESIAN_POINT ( 'NONE',  ( -37.99839555572501837, -114.9929510916434339, 12.65937477241748965 ) ) ;
#2080=CARTESIAN_POINT ( 'NONE',  ( -34.50000000000000000, -112.0269151300720409, -0.7876962586524208776 ) ) ;
#2087=CARTESIAN_POINT ( 'NONE',  ( -35.50000000000000000, -115.9929510916434481, 12.57451923796416260 ) ) ;
#2088=CARTESIAN_POINT ( 'NONE',  ( -35.50000000000000711, -115.9821387493194891, -0.8839717462762166633 ) ) ;
#2100=CARTESIAN_POINT ( 'NONE',  ( -37.66520193420439000, -113.2509883718312977, 6.941024454178450043 ) ) ;
#2112=CARTESIAN_POINT ( 'NONE',  ( -37.05926240293131713, -112.0000000000000142, 5.121475545821551734 ) ) ;
#2136=CARTESIAN_POINT ( 'NONE',  ( -38.45611840935523418, -115.3723087153909432, 5.066024454178449155 ) ) ;
#2137=CARTESIAN_POINT ( 'NONE',  ( -34.50000000000000000, -115.6492853190479337, 9.359470924297957239 ) ) ;
#2148=CARTESIAN_POINT ( 'NONE',  ( -35.62769128460905677, -112.5438815906447729, 5.308975545821551734 ) ) ;
#2164=CARTESIAN_POINT ( 'NONE',  ( -37.05926240293131713, -112.0000000000000142, 9.621475545821551734 ) ) ;
#2170=CARTESIAN_POINT ( 'NONE',  ( -35.50000000000000711, -112.0140978167138712, 0.7502176474015694874 ) ) ;
#2181=CARTESIAN_POINT ( 'NONE',  ( -34.80050084267117683, -114.9929510916434339, 13.54034599209289169 ) ) ;
#2183=CARTESIAN_POINT ( 'NONE',  ( -37.98402046630260287, -114.9929510916434339, 12.74811950270164118 ) ) ;
#2185=EDGE_CURVE ( 'NONE', #12261, #34373, #29027, .T. ) ;
#2186=CARTESIAN_POINT ( 'NONE',  ( -34.50000000000000000, -114.9656200615856818, 10.26631071845107179 ) ) ;
#2195=CARTESIAN_POINT ( 'NONE',  ( -38.00000068757622529, -114.9929510916434339, 12.61439929482944855 ) ) ;
#2197=CARTESIAN_POINT ( 'NONE',  ( -39.99999999999999289, -113.9407375970686758, 2.253524454178448710 ) ) ;
#2205=CARTESIAN_POINT ( 'NONE',  ( -34.92058450342251064, -116.1632251905417945, 4.691024454178447378 ) ) ;
#2217=CARTESIAN_POINT ( 'NONE',  ( -34.50000000000000000, -111.0140978167138570, 0.2502176474015764263 ) ) ;
#2222=CARTESIAN_POINT ( 'NONE',  ( -35.50000000000000711, -114.9925223117477202, 10.47601618151863079 ) ) ;
#2223=CARTESIAN_POINT ( 'NONE',  ( -38.00000000000000711, -113.9929510916434339, 10.85830208992306822 ) ) ;
#2227=CARTESIAN_POINT ( 'NONE',  ( -37.58145695302688694, -113.9929510916434339, 13.11211614918362756 ) ) ;
#2229=CARTESIAN_POINT ( 'NONE',  ( -37.37500000000009237, -115.9929510916434481, 13.11852480586264846 ) ) ;
#2241=CARTESIAN_POINT ( 'NONE',  ( -35.50000000000000711, -112.6043641208289188, 1.789429170677330649 ) ) ;
#2243=CARTESIAN_POINT ( 'NONE',  ( -35.50000000000000711, -114.9929510916434339, 12.44250253426871033 ) ) ;
#2248=CARTESIAN_POINT ( 'NONE',  ( -35.50000000000000000, -114.3474311500471572, -2.624782352598442614 ) ) ;
#2251=CARTESIAN_POINT ( 'NONE',  ( -37.76916472181487450, -111.9754527089670404, 2.534774454178448710 ) ) ;
#2258=CARTESIAN_POINT ( 'NONE',  ( -34.50000000000000000, -112.9977353549762000, -0.6247823525983134951 ) ) ;
#2264=CARTESIAN_POINT ( 'NONE',  ( -38.00000000000000711, -114.9929510916434339, 12.60752341388803721 ) ) ;
#2268=CARTESIAN_POINT ( 'NONE',  ( -34.50000000000000000, -113.4307644833805000, -1.624782352598427959 ) ) ;
#2273=CARTESIAN_POINT ( 'NONE',  ( -35.50000000000000711, -114.0882517521923489, 9.510534276948430232 ) ) ;
#2294=CARTESIAN_POINT ( 'NONE',  ( -35.54388159064475872, -115.3723087153909432, 7.183975545821551734 ) ) ;
#2314=CARTESIAN_POINT ( 'NONE',  ( -37.76916472181487450, -111.9754527089670404, 4.034774454178449155 ) ) ;
#2315=CARTESIAN_POINT ( 'NONE',  ( -34.50000000000000000, -115.9929510916434481, 12.26648026267477398 ) ) ;
#2324=CARTESIAN_POINT ( 'NONE',  ( -34.83677480945821259, -116.0794154965774965, 8.683975545821549957 ) ) ;
#2339=CARTESIAN_POINT ( 'NONE',  ( -36.23083527818513261, -111.9754527089670404, 9.715225545821551734 ) ) ;
#2344=CARTESIAN_POINT ( 'NONE',  ( -35.50000000000000711, -112.0141059978162019, -0.6575071456984691309 ) ) ;
#2350=CARTESIAN_POINT ( 'NONE',  ( -34.50000000000000000, -116.0012805033554883, -0.7876962586524312027 ) ) ;
#2351=CARTESIAN_POINT ( 'NONE',  ( -36.24999999999983658, -114.9929510916434339, 14.11852480586264846 ) ) ;
#2353=CARTESIAN_POINT ( 'NONE',  ( -35.50000000000000000, -113.9929510916434339, 10.53376102667243508 ) ) ;
#2356=CARTESIAN_POINT ( 'NONE',  ( -34.50000000000000000, -114.9929510916434339, 10.52826033068511435 ) ) ;
#2358=CARTESIAN_POINT ( 'NONE',  ( -37.80727372874345349, -114.9929510916434339, 13.01835785830664527 ) ) ;
#2364=CARTESIAN_POINT ( 'NONE',  ( -37.99359134332094357, -114.9929510916434339, 12.69998175888958158 ) ) ;
#2366=CARTESIAN_POINT ( 'NONE',  ( -36.94073759706868287, -112.0000000000000142, 4.128524454178449155 ) ) ;
#2375=CARTESIAN_POINT ( 'NONE',  ( -39.97545270896702618, -112.6980969099493990, 5.347274454178449155 ) ) ;
#2381=EDGE_CURVE ( 'NONE', #19761, #12261, #3715, .T. ) ;
#2388=CARTESIAN_POINT ( 'NONE',  ( -34.50000000000000000, -112.5389594332240222, 2.818899826424027477 ) ) ;
#2392=CARTESIAN_POINT ( 'NONE',  ( -34.50000000000000000, -113.9929510916434339, 10.50625754673587409 ) ) ;
#2396=CARTESIAN_POINT ( 'NONE',  ( -37.46093750000000711, -113.9929510916434339, 13.11852480586264846 ) ) ;
#2397=CARTESIAN_POINT ( 'NONE',  ( -37.99999897736217491, -115.9929510916434481, 12.62466071271733092 ) ) ;
#2409=CARTESIAN_POINT ( 'NONE',  ( -35.50000000000000000, -113.0140978167138712, 0.8752176474015934682 ) ) ;
#2412=CARTESIAN_POINT ( 'NONE',  ( -35.50000000000000711, -114.9929510916434339, 10.52000928670414126 ) ) ;
#2416=CARTESIAN_POINT ( 'NONE',  ( -35.50000000000000000, -111.0140978167138570, -0.3122823525984338988 ) ) ;
#2419=CARTESIAN_POINT ( 'NONE',  ( -38.45611840935523418, -115.3723087153909432, 2.066024454178448710 ) ) ;
#2424=CARTESIAN_POINT ( 'NONE',  ( -34.50000000000000000, -113.0140978167138712, 0.8127176474015720409 ) ) ;
#2430=CARTESIAN_POINT ( 'NONE',  ( -37.53269373325071712, -114.9929510916434339, 13.11752178341324360 ) ) ;
#2433=CARTESIAN_POINT ( 'NONE',  ( -34.50000000000000000, -115.1446187476384040, -1.616767172155725740 ) ) ;
#2439=CARTESIAN_POINT ( 'NONE',  ( -38.00000000000000711, -115.9929510916434481, 11.21034663311206181 ) ) ;
#2461=CARTESIAN_POINT ( 'NONE',  ( -39.02454729103295961, -113.2308352781851539, 4.840225545821551734 ) ) ;
#2481=CARTESIAN_POINT ( 'NONE',  ( -36.23083527818513261, -116.0245472910329880, 3.284774454178449155 ) ) ;
#2483=CARTESIAN_POINT ( 'NONE',  ( -37.37500000000009237, -115.9929510916434481, 14.11852480586265024 ) ) ;
#2494=CARTESIAN_POINT ( 'NONE',  ( -36.11231047232249125, -115.9754527089670262, 4.277725545821551734 ) ) ;
#2515=CARTESIAN_POINT ( 'NONE',  ( -35.50000000000000711, -112.9185811467682754, 1.870920967077121411 ) ) ;
#2521=CARTESIAN_POINT ( 'NONE',  ( -34.50000000000000000, -112.0140978167138712, -0.1247823525984259746 ) ) ;
#2525=CARTESIAN_POINT ( 'NONE',  ( -37.59808119975203766, -114.9929510916434339, 14.11551573851448893 ) ) ;
#2529=CARTESIAN_POINT ( 'NONE',  ( -38.00000000000000711, -114.9929510916434339, 12.56351784598954779 ) ) ;
#2531=CARTESIAN_POINT ( 'NONE',  ( -34.50000000000000000, -114.9929510916434339, 10.85830208992344303 ) ) ;
#2538=CARTESIAN_POINT ( 'NONE',  ( -35.97955704204053262, -114.9929510916434339, 13.11812344617474579 ) ) ;
#2541=CARTESIAN_POINT ( 'NONE',  ( -37.76916472181487450, -111.9754527089670404, 8.534774454178448266 ) ) ;
#2551=CARTESIAN_POINT ( 'NONE',  ( -35.69809690994938478, -111.0245472910330022, 7.222274454178449155 ) ) ;
#2554=CARTESIAN_POINT ( 'NONE',  ( -35.50000000000000711, -116.0140978167138712, -0.3747823525984422255 ) ) ;
#2563=CARTESIAN_POINT ( 'NONE',  ( -34.50000000000000000, -113.1807644833805426, -2.624782352598442614 ) ) ;
#2566=CARTESIAN_POINT ( 'NONE',  ( -35.50000000000000711, -114.9929510916434339, 10.94631322572069365 ) ) ;
#2568=CARTESIAN_POINT ( 'NONE',  ( -35.61121590948313553, -113.9929510916434339, 14.07058620477040733 ) ) ;
#2571=CARTESIAN_POINT ( 'NONE',  ( -37.46874999999995737, -113.9929510916434339, 13.11852480586264846 ) ) ;
#2572=CARTESIAN_POINT ( 'NONE',  ( -35.50000000000000711, -114.9929510916434339, 10.53376102667243508 ) ) ;
#2586=CARTESIAN_POINT ( 'NONE',  ( -35.50000000000000711, -116.0140978167138712, -0.4685323525984310677 ) ) ;
#2588=CARTESIAN_POINT ( 'NONE',  ( -35.50000000000000711, -114.9912366357066986, 10.44580456020104720 ) ) ;
#2592=CARTESIAN_POINT ( 'NONE',  ( -35.50000000000000000, -111.6790780953339066, 2.383953864837686343 ) ) ;
#2595=CARTESIAN_POINT ( 'NONE',  ( -35.62769128460905677, -115.4561184093552413, 3.191024454178449155 ) ) ;
#2599=CARTESIAN_POINT ( 'NONE',  ( -34.50000000000000000, -114.1807644833817648, -0.6247823525984269599 ) ) ;
#2607=CARTESIAN_POINT ( 'NONE',  ( -35.50000000000000000, -113.9929510916430075, 10.50625754673586876 ) ) ;
#2610=CARTESIAN_POINT ( 'NONE',  ( -34.50000000000000000, -112.7549084230351752, -1.592823285203595285 ) ) ;
#2611=CARTESIAN_POINT ( 'NONE',  ( -36.99999999999988631, -115.9929510916434481, 14.11852480586265024 ) ) ;
#2617=CARTESIAN_POINT ( 'NONE',  ( -38.00000000000000711, -115.9929510916434481, 12.53051367006571937 ) ) ;
#2639=CARTESIAN_POINT ( 'NONE',  ( -35.62769128460905677, -112.5438815906447729, 8.308975545821549957 ) ) ;
#2661=CARTESIAN_POINT ( 'NONE',  ( -38.95206139890799335, -115.9929510916434481, 13.00730889637963550 ) ) ;
#2671=CARTESIAN_POINT ( 'NONE',  ( -36.52652403469559061, -114.9754527089670262, 4.277725545821552622 ) ) ;
#2702=CARTESIAN_POINT ( 'NONE',  ( -34.50000000000000000, -115.3362660311619692, -1.573728109101206085 ) ) ;
#2703=CARTESIAN_POINT ( 'NONE',  ( -35.75562914091914024, -114.9929510916434339, 14.09929883582542409 ) ) ;
#2705=CARTESIAN_POINT ( 'NONE',  ( -35.50000000000000000, -113.9929510916438460, 10.50625754673626133 ) ) ;
#2707=CARTESIAN_POINT ( 'NONE',  ( -36.01562499999996447, -114.9929510916434339, 14.11852480586264846 ) ) ;
#2721=CARTESIAN_POINT ( 'NONE',  ( -37.05926240293133134, -116.9999999999999858, 1.878524454178448710 ) ) ;
#2730=CARTESIAN_POINT ( 'NONE',  ( -39.16322519054179452, -116.0794154965774823, 8.066024454178448266 ) ) ;
#2746=CARTESIAN_POINT ( 'NONE',  ( -34.50000000000000000, -116.6134300264884445, -1.853877267570539944 ) ) ;
#2753=CARTESIAN_POINT ( 'NONE',  ( -35.50000000000000711, -114.9929296450195721, 10.49869535309826674 ) ) ;
#2754=CARTESIAN_POINT ( 'NONE',  ( -37.34375000000001421, -113.9929510916434339, 14.11852480586265024 ) ) ;
#2757=CARTESIAN_POINT ( 'NONE',  ( -34.50000000000000000, -113.9929510916430075, 10.50625754673586876 ) ) ;
#2758=CARTESIAN_POINT ( 'NONE',  ( -39.00000000000000711, -114.9929510916434339, 12.59102132592608925 ) ) ;
#2759=CARTESIAN_POINT ( 'NONE',  ( -35.50000000000000711, -114.0882517521923489, 9.510534276948430232 ) ) ;
#2772=CARTESIAN_POINT ( 'NONE',  ( -35.50000000000000000, -113.0140978167136581, 0.8752176474015690433 ) ) ;
#2774=CARTESIAN_POINT ( 'NONE',  ( -38.02454729103296671, -114.3549511594417396, 5.159774454178449155 ) ) ;
#2781=CARTESIAN_POINT ( 'NONE',  ( -35.50000000000000000, -111.2304026862503719, 1.811733666967775713 ) ) ;
#2784=CARTESIAN_POINT ( 'NONE',  ( -35.00000000000000000, -114.0592624029313242, 4.503524454178448266 ) ) ;
#2789=CARTESIAN_POINT ( 'NONE',  ( -34.50000000000000000, -113.4307644833805142, -0.6247823525984269599 ) ) ;
#2796=CARTESIAN_POINT ( 'NONE',  ( -35.50000102263781798, -113.9929510916434339, 12.62466071271731494 ) ) ;
#2800=CARTESIAN_POINT ( 'NONE',  ( -34.50000000000000000, -111.0140978167138570, -0.4997823525984338988 ) ) ;
#2801=CARTESIAN_POINT ( 'NONE',  ( -38.95206139890799335, -115.9929510916434481, 13.00730889637963550 ) ) ;
#2807=CARTESIAN_POINT ( 'NONE',  ( -38.00000000000000711, -115.9929510916434481, 12.17846912687782179 ) ) ;
#2827=CARTESIAN_POINT ( 'NONE',  ( -34.97545270896703329, -114.7691647218148745, 7.090225545821550845 ) ) ;
#2835=CARTESIAN_POINT ( 'NONE',  ( -35.50000000000000711, -114.1068310684433129, 9.512752019463897923 ) ) ;
#2842=CARTESIAN_POINT ( 'NONE',  ( -38.99984940073100148, -115.9929510916434481, 12.64306614848957544 ) ) ;
#2850=CARTESIAN_POINT ( 'NONE',  ( -36.25098837183130485, -114.6652019342044184, 4.183975545821551734 ) ) ;
#2876=CARTESIAN_POINT ( 'NONE',  ( -34.50000000000000000, -112.1403507321855528, -1.128496220798856253 ) ) ;
#2877=CARTESIAN_POINT ( 'NONE',  ( -37.18750000000006395, -114.9929510916434339, 14.11852480586264846 ) ) ;
#2878=CARTESIAN_POINT ( 'NONE',  ( -35.50000000000000000, -113.9186338266397058, 10.49738657667399266 ) ) ;
#2880=CARTESIAN_POINT ( 'NONE',  ( -36.00976557831293690, -114.9929510916434339, 14.11852773550420359 ) ) ;
#2892=CARTESIAN_POINT ( 'NONE',  ( -39.07941549657748936, -111.8367748094582055, 6.941024454178450043 ) ) ;
#2903=CARTESIAN_POINT ( 'NONE',  ( -35.81662171581204746, -117.0245472910329738, 7.784774454178449155 ) ) ;
#2909=EDGE_CURVE ( 'NONE', #14462, #19761, #12277, .T. ) ;
#2915=CARTESIAN_POINT ( 'NONE',  ( -34.50000000000000000, -115.1449503510569059, -2.621568770093253953 ) ) ;
#2920=CARTESIAN_POINT ( 'NONE',  ( -37.50613590685470911, -114.9929510916434339, 13.11852378322482515 ) ) ;
#2921=CARTESIAN_POINT ( 'NONE',  ( -34.49999793727135966, -113.9929510916434339, 12.61164896875036767 ) ) ;
#2924=CARTESIAN_POINT ( 'NONE',  ( -34.50000000000000000, -113.9929510916434339, 10.50625754673577994 ) ) ;
#2925=CARTESIAN_POINT ( 'NONE',  ( -38.99924736195578134, -114.9929510916434339, 12.66759465831984777 ) ) ;
#2927=CARTESIAN_POINT ( 'NONE',  ( -35.50000000000000711, -114.1712995509219724, 9.522174004479579068 ) ) ;
#2940=CARTESIAN_POINT ( 'NONE',  ( -35.50000000000000711, -116.0140978167138712, -0.5622823525984409487 ) ) ;
#2942=CARTESIAN_POINT ( 'NONE',  ( -36.02454729103298092, -114.4734759653044307, 6.097274454178449155 ) ) ;
#2950=CARTESIAN_POINT ( 'NONE',  ( -35.50000000000000000, -115.5324766040685631, -2.560864217809699195 ) ) ;
#2953=CARTESIAN_POINT ( 'NONE',  ( -37.88768952767750164, -115.9754527089670262, 6.472274454178450043 ) ) ;
#2958=CARTESIAN_POINT ( 'NONE',  ( -34.50000000000000000, -115.0140978167140986, -0.6247823525984417259 ) ) ;
#2960=( BOUNDED_SURFACE ( )  B_SPLINE_SURFACE ( 3, 3, ( 
 ( #31743, #31917, #12675, #4396, #15162, #31572, #17700, #14993, #34273, #26718, #12851, #1324, #15344, #26356, #23652, #18414, #9960, #12304, #15521, #26539, #23828, #21106, #2054, #32107, #7436, #4757, #23275, #13028, #24018, #35004, #32284, #16050, #2588, #32455, #7782, #7965, #29772, #5285, #5113, #18768, #16225, #27069, #2412, #13380, #13552, #15876, #10676, #18593, #8138, #24362, #24187, #35180, #35350, #21636, #26901, #10496, #27247, #32642, #18945, #29945, #2243, #24540, #19118, #21461, #35535, #10862, #21821, #5456, #32819, #7603, #30119, #16407, #27426, #29593, #4932, #13209, #34751, #18354, #10072, #12783, #21038, #32399, #20855, #4701, #35119, #23763, #7718, #26110, #7189, #32046, #29179, #31856, #24128, #7381, #15633, #34574, #29354, #4333, #4528, #18701, #1628, #28985, #7011, #26655, #15459, #4158, #15100, #1440, #32223, #9720, #12420, #7550, #23405, #21228, #18168, #34402, #18529, #26474, #9889, #20679, #1809, #31677, #34944, #12607, #1985, #17986, #12962, #23947, #26293, #10266, #15278, #29533, #2183, #23581, #4866, #15809, #26829, #13153, #10443, #21402, #16344, #11144, #11319, #7901, #3049, #16082, #2529, #19226, #5741, #30057, #27008, #19058, #10969, #21570, #22111, #24652, #33107, #35295 ),
 ( #10795, #35464, #2878, #5397, #24476, #13494, #8431, #24304, #21934, #5049, #14008, #21754, #18886, #29881, #27357, #32749, #10613, #5227, #16532, #32929, #30232, #8251, #32567, #2705, #25001, #8075, #13840, #13672, #5570, #326, #24828, #29700, #27186, #16167, #27542, #152, #19415, #27711, #30413, #16699, #22289, #33284, #8600, #15993, #2353, #13323, #9404, #25813, #23083, #26340, #6523, #3846, #29031, #18034, #12289, #31559, #1139, #14975, #31193, #6704, #1675, #17858, #7058, #25982, #31018, #12469, #4380, #31374, #15325, #26152, #20361, #9940, #28498, #20188, #33901, #6884, #17685, #34620, #6350, #23634, #23455, #953, #17316, #34450, #14617, #9767, #28684, #28321, #20728, #12112, #34079, #3667, #4031, #11937, #1486, #14806, #1305, #9230, #23260, #34257, #17498, #9590, #25628, #28855, #12657, #22908, #20558, #4207, #31727, #15147, #13538, #35162, #7590, #2396, #2571, #34797, #29928, #26881, #29400, #10483, #32618, #21270, #18217, #10309, #2227, #12830, #13364, #15858, #24346, #26525, #13195, #20903, #24168, #24524, #21444, #16208, #4745, #18929, #32441, #7765, #7948, #32269, #18577, #18398, #18747, #5269, #27229, #15682, #35513, #29578, #31901, #1859, #21086, #7236, #29223, #10660, #4571, #23813 ),
 ( #15505, #35336, #10119, #32091, #7421, #26700, #2036, #13012, #23997, #34988, #4913, #21617, #29751, #5095, #16036, #27054, #30279, #198, #24873, #5619, #2924, #6135, #21980, #32976, #27755, #13883, #2757, #16389, #5956, #19271, #16580, #24698, #30460, #11182, #8291, #22154, #25408, #8650, #8819, #19102, #33152, #3448, #14228, #3095, #14400, #25045, #8481, #27921, #28105, #25, #19781, #16745, #27588, #368, #22504, #19461, #8120, #5788, #14048, #13719, #3270, #11365, #25228, #27408, #22331, #10842, #33327, #21801, #19617, #17097, #30622, #30794, #16915, #551, #33494, #11538, #32799, #30099, #5437, #11014, #34404, #20145, #15280, #25764, #11703, #6307, #901, #31679, #22672, #26112, #28987, #17274, #1442, #12064, #28638, #33664, #4335, #9722, #4161, #722, #3624, #9001, #7013, #14569, #19966, #12422, #30973, #28279, #17810, #23038, #31151, #15103, #23408, #6482, #1093, #14755, #17455, #28453, #17989, #11883, #22860, #17635, #3798, #25583, #20682, #20322, #33856, #28811, #9183, #34036, #9363, #31516, #31330, #6656, #3984, #14929, #25940, #12248, #1262, #23221, #34214, #9544, #20510, #6838, #5229, #18703, #9891, #7720, #4703, #29884, #29702, #7383, #21040, #26295, #18356, #21230, #4868, #32227 ),
 ( #34576, #10268, #18888, #12609, #29359, #20857, #34753, #24306, #13325, #7553, #26831, #32048, #18531, #26478, #1987, #21572, #13155, #12964, #29181, #29536, #1631, #15811, #1811, #15462, #15635, #26657, #23585, #5051, #2186, #23950, #32569, #34946, #31859, #10445, #4530, #35298, #12785, #10075, #7191, #24130, #35122, #21405, #23765, #2356, #32402, #15996, #27010, #10615, #7903, #18170, #16169, #2531, #32751, #14189, #11321, #27188, #10972, #24830, #8079, #16877, #5399, #13497, #19060, #27360, #16346, #16702, #514, #13844, #5912, #11146, #10797, #13674, #32931, #19418, #328, #5573, #22291, #24654, #14369, #30416, #8253, #3051, #19228, #21937, #25003, #16535, #30234, #27544, #8603, #21756, #22113, #24478, #25191, #2880, #2707, #155, #33109, #8433, #30059, #5743, #14011, #27713, #33287, #19575, #30579, #27881, #11493, #3226, #22463, #33453, #8776, #19743, #30755, #35466, #3579, #30935, #9324, #8956, #12207, #4123, #34356, #20281, #28413, #23181, #23358, #19921, #15063, #12026, #14526, #31291, #17768, #6440, #3410, #31113, #22997, #33623, #34177, #1055, #9501, #11661, #34000, #6090, #6615, #9682, #17586, #1403, #25543, #26073, #28594, #3945, #28770, #17410, #3754, #855, #14890, #12380, #20637, #11837 ),
 ( #25902, #1230, #20459, #31471, #6267, #14709, #17056, #22818, #6797, #9143, #28069, #14358, #25368, #679, #33818, #17232, #22631, #28239, #20105, #25723, #26611, #10222, #1946, #4660, #12921, #2137, #23719, #13284, #4296, #15590, #24263, #17946, #34711, #26247, #4482, #29658, #18661, #23906, #32181, #26432, #34899, #31816, #7337, #26974, #18489, #18313, #34533, #21188, #35249, #7508, #7152, #20813, #20998, #32001, #31636, #35079, #29488, #1762, #2315, #29312, #1587, #15768, #9849, #5000, #18126, #15421, #6973, #10035, #4827, #26787, #29130, #7677, #12744, #13114, #24095, #10403, #21361, #23538, #28947, #15236, #12566, #15956, #32354, #10571, #16301, #30190, #3184, #115, #16837, #30020, #19534, #24791, #33067, #33244, #21897, #32891, #19022, #19367, #8564, #30540, #5356, #468, #10931, #32523, #27143, #21716, #27842, #7855, #11273, #14141, #2483, #22246, #8213, #13803, #18846, #25141, #5870, #24964, #21524, #24433, #29846, #5187, #35420, #16126, #13453, #10750, #32713, #3013, #19191, #27316, #287, #8040, #2661, #5527, #35602, #13624, #24615, #16485, #27503, #2842, #11106, #22074, #8384, #30372, #5701, #16661, #13973, #27672, #11793, #9450, #6565, #811, #26027, #8913, #638, #14313, #22953, #22772 ),
 ( #11451, #3895, #30715, #28547, #25494, #15023, #14851, #28195, #6225, #22417, #3536, #17009, #17541, #19877, #17187, #25319, #31068, #33773, #33579, #9102, #33409, #9278, #20409, #19699, #20062, #4081, #25860, #3709, #8731, #25675, #6396, #1186, #28730, #11615, #31421, #17364, #30890, #1009, #23130, #28366, #6047, #14662, #11985, #3366, #12158, #33951, #34127, #28019, #20233, #22588, #31245, #6751, #17727, #14484, #28901, #1356, #23309, #17905, #35036, #32134, #12332, #31772, #9989, #4251, #2087, #26197, #34309, #15188, #12518, #1535, #1904, #21316, #34668, #26746, #31951, #31597, #34490, #18078, #4614, #21140, #26382, #7464, #9809, #20772, #15548, #29079, #23858, #4428, #7105, #10172, #1716, #15371, #12700, #29441, #6932, #7287, #9638, #10356, #23676, #23495, #20950, #18261, #29266, #26566, #12879, #34847, #18444, #4786, #15729, #13066, #24051, #32310, #7635, #18622, #29620, #4958, #15914, #20599, #26931, #24392, #16083, #30148, #29804, #33027, #24924, #21856, #5485, #32850, #35566, #8169, #8340, #18980, #9010, #35207, #10891, #19974, #13241, #29978, #21487, #35378, #247, #13935, #19150, #27461, #21674, #16440, #27100, #2617, #22201, #13766, #13581, #5143, #2807, #30982, #24751, #2439, #13410, #16256 ),
 ( #6314, #19321, #10527, #30334, #5316, #2273, #5666, #7997, #32676, #24216, #27275, #32479, #22034, #10704, #24575, #77, #16625, #7812, #18804, #27638, #11064, #2976, #11232, #33675, #20691, #34044, #12073, #17283, #9371, #22869, #12433, #25775, #23046, #31160, #1270, #6667, #3808, #31340, #31867, #15111, #15291, #25592, #3996, #9902, #31689, #9553, #20865, #31524, #14938, #34413, #34585, #6489, #26303, #23230, #1102, #6848, #28995, #17644, #14580, #28648, #34223, #9192, #9730, #12256, #7021, #33866, #20520, #28287, #17820, #3631, #28819, #12618, #20330, #1639, #4169, #26120, #4345, #25947, #1453, #14766, #23416, #23593, #913, #17997, #11893, #20153, #17464, #28462, #7393, #2538, #29191, #32580, #35476, #23775, #7914, #18541, #35132, #4538, #10807, #16177, #10624, #21766, #10085, #15470, #13505, #21051, #7198, #18896, #18179, #12795, #24313, #29544, #26666, #21581, #29893, #1998, #32234, #21241, #12973, #34955, #24487, #18365, #29367, #24138, #10276, #34761, #5237, #26842, #26488, #35306, #27199, #7560, #1819, #2364, #4877, #32056, #4712, #15644, #23960, #18713, #15821, #2195, #13163, #10453, #21414, #32410, #7729, #29715, #5059, #16004, #27019, #13335, #30425, #22472, #27723, #27369, #30242, #13854 ) ),
 .UNSPECIFIED., .T., .F., .F. ) 
 B_SPLINE_SURFACE_WITH_KNOTS ( ( 4, 3, 4 ),
 ( 4, 2, 2, 2, 2, 2, 2, 2, 2, 2, 2, 2, 2, 2, 2, 2, 2, 2, 2, 2, 2, 2, 2, 2, 2, 2, 2, 2, 2, 2, 2, 2, 2, 2, 2, 2, 2, 2, 2, 2, 2, 2, 2, 2, 2, 2, 2, 2, 2, 2, 2, 2, 2, 2, 2, 2, 2, 2, 2, 2, 2, 2, 2, 2, 2, 2, 2, 2, 2, 2, 2, 2, 2, 2, 2, 2, 2, 2, 4 ),
 ( 0.000000000000000000, 0.5000000000000000000, 1.000000000000000000 ),
 ( 0.000000000000000000, 0.005381740036788157898, 0.008072610055182236413, 0.009418045064379276105, 0.01009076256897779508, 0.01076348007357631580, 0.01185104180586291078, 0.01293860353814950404, 0.01511372700272269054, 0.01946397393186906355, 0.02816446779016181304, 0.04556545550674730855, 0.08036743093991829956, 0.1151694063730892975, 0.1325703940896748034, 0.1412708879479675494, 0.1456211348771139225, 0.1477962583416871090, 0.1488838200739737161, 0.1499713818062602955, 0.1507624401091536004, 0.1515534984120469053, 0.1531356150178334874, 0.1562998482294066793, 0.1626283146525530909, 0.1752852474988458864, 0.2005991131914315051, 0.2512268445766027147, 0.3018545759617738966, 0.3271684416543594875, 0.3398253745006523108, 0.3461538409237986946, 0.3493180741353718588, 0.3509001907411584686, 0.3524823073469450785, 0.3548354025267266287, 0.3571884977065081790, 0.3618946880660712795, 0.3713070687851974805, 0.3901318302234498825, 0.4277813530999547420, 0.4654308759764596015, 0.4842556374147120035, 0.4936680181338382045, 0.4983742084934013050, 0.5007273036731828553, 0.5030803988529644055, 0.5053274392295320494, 0.5075744796060996933, 0.5120685603592350921, 0.5210567218655057786, 0.5390330448780472627, 0.5749856909031301200, 0.6109383369282129772, 0.6289146599407544613, 0.6379028214470251479, 0.6423969022001605467, 0.6446439425767281906, 0.6468909829532958344, 0.6492440781330773847, 0.6515971733128589349, 0.6563033636724220354, 0.6657157443915482364, 0.6845405058298006384, 0.7221900287063054424, 0.7598395515828102464, 0.7786643130210626484, 0.7880766937401888494, 0.7927828840997519499, 0.7951359792795336112, 0.7974890744593151615, 0.7990711910651018268, 0.8006533076708883812, 0.8038175408824614898, 0.8101460073056079292, 0.8228029401519008079, 0.8481168058444863433, 0.8987445372296576362, 1.000000000000000000 ),
 .UNSPECIFIED. ) 
 GEOMETRIC_REPRESENTATION_ITEM ( )  RATIONAL_B_SPLINE_SURFACE ( (
 ( 1.000000000000000000, 1.000000000000000000, 1.000000000000000000, 1.000000000000000000, 1.000000000000000000, 1.000000000000000000, 1.000000000000000000, 1.000000000000000000, 1.000000000000000000, 1.000000000000000000, 1.000000000000000000, 1.000000000000000000, 1.000000000000000000, 1.000000000000000000, 1.000000000000000000, 1.000000000000000000, 1.000000000000000000, 1.000000000000000000, 1.000000000000000000, 1.000000000000000000, 1.000000000000000000, 1.000000000000000000, 1.000000000000000000, 1.000000000000000000, 1.000000000000000000, 1.000000000000000000, 1.000000000000000000, 1.000000000000000000, 1.000000000000000000, 1.000000000000000000, 1.000000000000000000, 1.000000000000000000, 1.000000000000000000, 1.000000000000000000, 1.000000000000000000, 1.000000000000000000, 1.000000000000000000, 1.000000000000000000, 1.000000000000000000, 1.000000000000000000, 1.000000000000000000, 1.000000000000000000, 1.000000000000000000, 1.000000000000000000, 1.000000000000000000, 1.000000000000000000, 1.000000000000000000, 1.000000000000000000, 1.000000000000000000, 1.000000000000000000, 1.000000000000000000, 1.000000000000000000, 1.000000000000000000, 1.000000000000000000, 1.000000000000000000, 1.000000000000000000, 1.000000000000000000, 1.000000000000000000, 1.000000000000000000, 1.000000000000000000, 1.000000000000000000, 1.000000000000000000, 1.000000000000000000, 1.000000000000000000, 1.000000000000000000, 1.000000000000000000, 1.000000000000000000, 1.000000000000000000, 1.000000000000000000, 1.000000000000000000, 1.000000000000000000, 1.000000000000000000, 1.000000000000000000, 1.000000000000000000, 1.000000000000000000, 1.000000000000000000, 1.000000000000000000, 1.000000000000000000, 1.000000000000000000, 1.000000000000000000, 1.000000000000000000, 1.000000000000000000, 1.000000000000000000, 1.000000000000000000, 1.000000000000000000, 1.000000000000000000, 1.000000000000000000, 1.000000000000000000, 1.000000000000000000, 1.000000000000000000, 1.000000000000000000, 1.000000000000000000, 1.000000000000000000, 1.000000000000000000, 1.000000000000000000, 1.000000000000000000, 1.000000000000000000, 1.000000000000000000, 1.000000000000000000, 1.000000000000000000, 1.000000000000000000, 1.000000000000000000, 1.000000000000000000, 1.000000000000000000, 1.000000000000000000, 1.000000000000000000, 1.000000000000000000, 1.000000000000000000, 1.000000000000000000, 1.000000000000000000, 1.000000000000000000, 1.000000000000000000, 1.000000000000000000, 1.000000000000000000, 1.000000000000000000, 1.000000000000000000, 1.000000000000000000, 1.000000000000000000, 1.000000000000000000, 1.000000000000000000, 1.000000000000000000, 1.000000000000000000, 1.000000000000000000, 1.000000000000000000, 1.000000000000000000, 1.000000000000000000, 1.000000000000000000, 1.000000000000000000, 1.000000000000000000, 1.000000000000000000, 1.000000000000000000, 1.000000000000000000, 1.000000000000000000, 1.000000000000000000, 1.000000000000000000, 1.000000000000000000, 1.000000000000000000, 1.000000000000000000, 1.000000000000000000, 1.000000000000000000, 1.000000000000000000, 1.000000000000000000, 1.000000000000000000, 1.000000000000000000, 1.000000000000000000, 1.000000000000000000, 1.000000000000000000, 1.000000000000000000, 1.000000000000000000, 1.000000000000000000, 1.000000000000000000, 1.000000000000000000, 1.000000000000000000, 1.000000000000000000, 1.000000000000000000, 1.000000000000000000, 1.000000000000000000, 1.000000000000000000),
 ( 0.3333333333333333703, 0.3333333333333333703, 0.3333333333333333703, 0.3333333333333333703, 0.3333333333333333703, 0.3333333333333333703, 0.3333333333333333703, 0.3333333333333333703, 0.3333333333333333703, 0.3333333333333333703, 0.3333333333333333703, 0.3333333333333333703, 0.3333333333333333703, 0.3333333333333333703, 0.3333333333333333703, 0.3333333333333333703, 0.3333333333333333703, 0.3333333333333333703, 0.3333333333333333703, 0.3333333333333333703, 0.3333333333333333703, 0.3333333333333333703, 0.3333333333333333703, 0.3333333333333333703, 0.3333333333333333703, 0.3333333333333333703, 0.3333333333333333703, 0.3333333333333333703, 0.3333333333333333703, 0.3333333333333333703, 0.3333333333333333703, 0.3333333333333333703, 0.3333333333333333703, 0.3333333333333333703, 0.3333333333333333703, 0.3333333333333333703, 0.3333333333333333703, 0.3333333333333333703, 0.3333333333333333703, 0.3333333333333333703, 0.3333333333333333703, 0.3333333333333333703, 0.3333333333333333703, 0.3333333333333333703, 0.3333333333333333703, 0.3333333333333333703, 0.3333333333333333703, 0.3333333333333333703, 0.3333333333333333703, 0.3333333333333333703, 0.3333333333333333703, 0.3333333333333333703, 0.3333333333333333703, 0.3333333333333333703, 0.3333333333333333703, 0.3333333333333333703, 0.3333333333333333703, 0.3333333333333333703, 0.3333333333333333703, 0.3333333333333333703, 0.3333333333333333703, 0.3333333333333333703, 0.3333333333333333703, 0.3333333333333333703, 0.3333333333333333703, 0.3333333333333333703, 0.3333333333333333703, 0.3333333333333333703, 0.3333333333333333703, 0.3333333333333333703, 0.3333333333333333703, 0.3333333333333333703, 0.3333333333333333703, 0.3333333333333333703, 0.3333333333333333703, 0.3333333333333333703, 0.3333333333333333703, 0.3333333333333333703, 0.3333333333333333703, 0.3333333333333333703, 0.3333333333333333703, 0.3333333333333333703, 0.3333333333333333703, 0.3333333333333333703, 0.3333333333333333703, 0.3333333333333333703, 0.3333333333333333703, 0.3333333333333333703, 0.3333333333333333703, 0.3333333333333333703, 0.3333333333333333703, 0.3333333333333333703, 0.3333333333333333703, 0.3333333333333333703, 0.3333333333333333703, 0.3333333333333333703, 0.3333333333333333703, 0.3333333333333333703, 0.3333333333333333703, 0.3333333333333333703, 0.3333333333333333703, 0.3333333333333333703, 0.3333333333333333703, 0.3333333333333333703, 0.3333333333333333703, 0.3333333333333333703, 0.3333333333333333703, 0.3333333333333333703, 0.3333333333333333703, 0.3333333333333333703, 0.3333333333333333703, 0.3333333333333333703, 0.3333333333333333703, 0.3333333333333333703, 0.3333333333333333703, 0.3333333333333333703, 0.3333333333333333703, 0.3333333333333333703, 0.3333333333333333703, 0.3333333333333333703, 0.3333333333333333703, 0.3333333333333333703, 0.3333333333333333703, 0.3333333333333333703, 0.3333333333333333703, 0.3333333333333333703, 0.3333333333333333703, 0.3333333333333333703, 0.3333333333333333703, 0.3333333333333333703, 0.3333333333333333703, 0.3333333333333333703, 0.3333333333333333703, 0.3333333333333333703, 0.3333333333333333703, 0.3333333333333333703, 0.3333333333333333703, 0.3333333333333333703, 0.3333333333333333703, 0.3333333333333333703, 0.3333333333333333703, 0.3333333333333333703, 0.3333333333333333703, 0.3333333333333333703, 0.3333333333333333703, 0.3333333333333333703, 0.3333333333333333703, 0.3333333333333333703, 0.3333333333333333703, 0.3333333333333333703, 0.3333333333333333703, 0.3333333333333333703, 0.3333333333333333703, 0.3333333333333333703, 0.3333333333333333703, 0.3333333333333333703, 0.3333333333333333703, 0.3333333333333333703),
 ( 0.3333333333333333703, 0.3333333333333333703, 0.3333333333333333703, 0.3333333333333333703, 0.3333333333333333703, 0.3333333333333333703, 0.3333333333333333703, 0.3333333333333333703, 0.3333333333333333703, 0.3333333333333333703, 0.3333333333333333703, 0.3333333333333333703, 0.3333333333333333703, 0.3333333333333333703, 0.3333333333333333703, 0.3333333333333333703, 0.3333333333333333703, 0.3333333333333333703, 0.3333333333333333703, 0.3333333333333333703, 0.3333333333333333703, 0.3333333333333333703, 0.3333333333333333703, 0.3333333333333333703, 0.3333333333333333703, 0.3333333333333333703, 0.3333333333333333703, 0.3333333333333333703, 0.3333333333333333703, 0.3333333333333333703, 0.3333333333333333703, 0.3333333333333333703, 0.3333333333333333703, 0.3333333333333333703, 0.3333333333333333703, 0.3333333333333333703, 0.3333333333333333703, 0.3333333333333333703, 0.3333333333333333703, 0.3333333333333333703, 0.3333333333333333703, 0.3333333333333333703, 0.3333333333333333703, 0.3333333333333333703, 0.3333333333333333703, 0.3333333333333333703, 0.3333333333333333703, 0.3333333333333333703, 0.3333333333333333703, 0.3333333333333333703, 0.3333333333333333703, 0.3333333333333333703, 0.3333333333333333703, 0.3333333333333333703, 0.3333333333333333703, 0.3333333333333333703, 0.3333333333333333703, 0.3333333333333333703, 0.3333333333333333703, 0.3333333333333333703, 0.3333333333333333703, 0.3333333333333333703, 0.3333333333333333703, 0.3333333333333333703, 0.3333333333333333703, 0.3333333333333333703, 0.3333333333333333703, 0.3333333333333333703, 0.3333333333333333703, 0.3333333333333333703, 0.3333333333333333703, 0.3333333333333333703, 0.3333333333333333703, 0.3333333333333333703, 0.3333333333333333703, 0.3333333333333333703, 0.3333333333333333703, 0.3333333333333333703, 0.3333333333333333703, 0.3333333333333333703, 0.3333333333333333703, 0.3333333333333333703, 0.3333333333333333703, 0.3333333333333333703, 0.3333333333333333703, 0.3333333333333333703, 0.3333333333333333703, 0.3333333333333333703, 0.3333333333333333703, 0.3333333333333333703, 0.3333333333333333703, 0.3333333333333333703, 0.3333333333333333703, 0.3333333333333333703, 0.3333333333333333703, 0.3333333333333333703, 0.3333333333333333703, 0.3333333333333333703, 0.3333333333333333703, 0.3333333333333333703, 0.3333333333333333703, 0.3333333333333333703, 0.3333333333333333703, 0.3333333333333333703, 0.3333333333333333703, 0.3333333333333333703, 0.3333333333333333703, 0.3333333333333333703, 0.3333333333333333703, 0.3333333333333333703, 0.3333333333333333703, 0.3333333333333333703, 0.3333333333333333703, 0.3333333333333333703, 0.3333333333333333703, 0.3333333333333333703, 0.3333333333333333703, 0.3333333333333333703, 0.3333333333333333703, 0.3333333333333333703, 0.3333333333333333703, 0.3333333333333333703, 0.3333333333333333703, 0.3333333333333333703, 0.3333333333333333703, 0.3333333333333333703, 0.3333333333333333703, 0.3333333333333333703, 0.3333333333333333703, 0.3333333333333333703, 0.3333333333333333703, 0.3333333333333333703, 0.3333333333333333703, 0.3333333333333333703, 0.3333333333333333703, 0.3333333333333333703, 0.3333333333333333703, 0.3333333333333333703, 0.3333333333333333703, 0.3333333333333333703, 0.3333333333333333703, 0.3333333333333333703, 0.3333333333333333703, 0.3333333333333333703, 0.3333333333333333703, 0.3333333333333333703, 0.3333333333333333703, 0.3333333333333333703, 0.3333333333333333703, 0.3333333333333333703, 0.3333333333333333703, 0.3333333333333333703, 0.3333333333333333703, 0.3333333333333333703, 0.3333333333333333703, 0.3333333333333333703, 0.3333333333333333703, 0.3333333333333333703),
 ( 1.000000000000000000, 1.000000000000000000, 1.000000000000000000, 1.000000000000000000, 1.000000000000000000, 1.000000000000000000, 1.000000000000000000, 1.000000000000000000, 1.000000000000000000, 1.000000000000000000, 1.000000000000000000, 1.000000000000000000, 1.000000000000000000, 1.000000000000000000, 1.000000000000000000, 1.000000000000000000, 1.000000000000000000, 1.000000000000000000, 1.000000000000000000, 1.000000000000000000, 1.000000000000000000, 1.000000000000000000, 1.000000000000000000, 1.000000000000000000, 1.000000000000000000, 1.000000000000000000, 1.000000000000000000, 1.000000000000000000, 1.000000000000000000, 1.000000000000000000, 1.000000000000000000, 1.000000000000000000, 1.000000000000000000, 1.000000000000000000, 1.000000000000000000, 1.000000000000000000, 1.000000000000000000, 1.000000000000000000, 1.000000000000000000, 1.000000000000000000, 1.000000000000000000, 1.000000000000000000, 1.000000000000000000, 1.000000000000000000, 1.000000000000000000, 1.000000000000000000, 1.000000000000000000, 1.000000000000000000, 1.000000000000000000, 1.000000000000000000, 1.000000000000000000, 1.000000000000000000, 1.000000000000000000, 1.000000000000000000, 1.000000000000000000, 1.000000000000000000, 1.000000000000000000, 1.000000000000000000, 1.000000000000000000, 1.000000000000000000, 1.000000000000000000, 1.000000000000000000, 1.000000000000000000, 1.000000000000000000, 1.000000000000000000, 1.000000000000000000, 1.000000000000000000, 1.000000000000000000, 1.000000000000000000, 1.000000000000000000, 1.000000000000000000, 1.000000000000000000, 1.000000000000000000, 1.000000000000000000, 1.000000000000000000, 1.000000000000000000, 1.000000000000000000, 1.000000000000000000, 1.000000000000000000, 1.000000000000000000, 1.000000000000000000, 1.000000000000000000, 1.000000000000000000, 1.000000000000000000, 1.000000000000000000, 1.000000000000000000, 1.000000000000000000, 1.000000000000000000, 1.000000000000000000, 1.000000000000000000, 1.000000000000000000, 1.000000000000000000, 1.000000000000000000, 1.000000000000000000, 1.000000000000000000, 1.000000000000000000, 1.000000000000000000, 1.000000000000000000, 1.000000000000000000, 1.000000000000000000, 1.000000000000000000, 1.000000000000000000, 1.000000000000000000, 1.000000000000000000, 1.000000000000000000, 1.000000000000000000, 1.000000000000000000, 1.000000000000000000, 1.000000000000000000, 1.000000000000000000, 1.000000000000000000, 1.000000000000000000, 1.000000000000000000, 1.000000000000000000, 1.000000000000000000, 1.000000000000000000, 1.000000000000000000, 1.000000000000000000, 1.000000000000000000, 1.000000000000000000, 1.000000000000000000, 1.000000000000000000, 1.000000000000000000, 1.000000000000000000, 1.000000000000000000, 1.000000000000000000, 1.000000000000000000, 1.000000000000000000, 1.000000000000000000, 1.000000000000000000, 1.000000000000000000, 1.000000000000000000, 1.000000000000000000, 1.000000000000000000, 1.000000000000000000, 1.000000000000000000, 1.000000000000000000, 1.000000000000000000, 1.000000000000000000, 1.000000000000000000, 1.000000000000000000, 1.000000000000000000, 1.000000000000000000, 1.000000000000000000, 1.000000000000000000, 1.000000000000000000, 1.000000000000000000, 1.000000000000000000, 1.000000000000000000, 1.000000000000000000, 1.000000000000000000, 1.000000000000000000, 1.000000000000000000, 1.000000000000000000, 1.000000000000000000, 1.000000000000000000, 1.000000000000000000, 1.000000000000000000),
 ( 0.3333333333333333703, 0.3333333333333333703, 0.3333333333333333703, 0.3333333333333333703, 0.3333333333333333703, 0.3333333333333333703, 0.3333333333333333703, 0.3333333333333333703, 0.3333333333333333703, 0.3333333333333333703, 0.3333333333333333703, 0.3333333333333333703, 0.3333333333333333703, 0.3333333333333333703, 0.3333333333333333703, 0.3333333333333333703, 0.3333333333333333703, 0.3333333333333333703, 0.3333333333333333703, 0.3333333333333333703, 0.3333333333333333703, 0.3333333333333333703, 0.3333333333333333703, 0.3333333333333333703, 0.3333333333333333703, 0.3333333333333333703, 0.3333333333333333703, 0.3333333333333333703, 0.3333333333333333703, 0.3333333333333333703, 0.3333333333333333703, 0.3333333333333333703, 0.3333333333333333703, 0.3333333333333333703, 0.3333333333333333703, 0.3333333333333333703, 0.3333333333333333703, 0.3333333333333333703, 0.3333333333333333703, 0.3333333333333333703, 0.3333333333333333703, 0.3333333333333333703, 0.3333333333333333703, 0.3333333333333333703, 0.3333333333333333703, 0.3333333333333333703, 0.3333333333333333703, 0.3333333333333333703, 0.3333333333333333703, 0.3333333333333333703, 0.3333333333333333703, 0.3333333333333333703, 0.3333333333333333703, 0.3333333333333333703, 0.3333333333333333703, 0.3333333333333333703, 0.3333333333333333703, 0.3333333333333333703, 0.3333333333333333703, 0.3333333333333333703, 0.3333333333333333703, 0.3333333333333333703, 0.3333333333333333703, 0.3333333333333333703, 0.3333333333333333703, 0.3333333333333333703, 0.3333333333333333703, 0.3333333333333333703, 0.3333333333333333703, 0.3333333333333333703, 0.3333333333333333703, 0.3333333333333333703, 0.3333333333333333703, 0.3333333333333333703, 0.3333333333333333703, 0.3333333333333333703, 0.3333333333333333703, 0.3333333333333333703, 0.3333333333333333703, 0.3333333333333333703, 0.3333333333333333703, 0.3333333333333333703, 0.3333333333333333703, 0.3333333333333333703, 0.3333333333333333703, 0.3333333333333333703, 0.3333333333333333703, 0.3333333333333333703, 0.3333333333333333703, 0.3333333333333333703, 0.3333333333333333703, 0.3333333333333333703, 0.3333333333333333703, 0.3333333333333333703, 0.3333333333333333703, 0.3333333333333333703, 0.3333333333333333703, 0.3333333333333333703, 0.3333333333333333703, 0.3333333333333333703, 0.3333333333333333703, 0.3333333333333333703, 0.3333333333333333703, 0.3333333333333333703, 0.3333333333333333703, 0.3333333333333333703, 0.3333333333333333703, 0.3333333333333333703, 0.3333333333333333703, 0.3333333333333333703, 0.3333333333333333703, 0.3333333333333333703, 0.3333333333333333703, 0.3333333333333333703, 0.3333333333333333703, 0.3333333333333333703, 0.3333333333333333703, 0.3333333333333333703, 0.3333333333333333703, 0.3333333333333333703, 0.3333333333333333703, 0.3333333333333333703, 0.3333333333333333703, 0.3333333333333333703, 0.3333333333333333703, 0.3333333333333333703, 0.3333333333333333703, 0.3333333333333333703, 0.3333333333333333703, 0.3333333333333333703, 0.3333333333333333703, 0.3333333333333333703, 0.3333333333333333703, 0.3333333333333333703, 0.3333333333333333703, 0.3333333333333333703, 0.3333333333333333703, 0.3333333333333333703, 0.3333333333333333703, 0.3333333333333333703, 0.3333333333333333703, 0.3333333333333333703, 0.3333333333333333703, 0.3333333333333333703, 0.3333333333333333703, 0.3333333333333333703, 0.3333333333333333703, 0.3333333333333333703, 0.3333333333333333703, 0.3333333333333333703, 0.3333333333333333703, 0.3333333333333333703, 0.3333333333333333703, 0.3333333333333333703, 0.3333333333333333703, 0.3333333333333333703, 0.3333333333333333703, 0.3333333333333333703),
 ( 0.3333333333333333703, 0.3333333333333333703, 0.3333333333333333703, 0.3333333333333333703, 0.3333333333333333703, 0.3333333333333333703, 0.3333333333333333703, 0.3333333333333333703, 0.3333333333333333703, 0.3333333333333333703, 0.3333333333333333703, 0.3333333333333333703, 0.3333333333333333703, 0.3333333333333333703, 0.3333333333333333703, 0.3333333333333333703, 0.3333333333333333703, 0.3333333333333333703, 0.3333333333333333703, 0.3333333333333333703, 0.3333333333333333703, 0.3333333333333333703, 0.3333333333333333703, 0.3333333333333333703, 0.3333333333333333703, 0.3333333333333333703, 0.3333333333333333703, 0.3333333333333333703, 0.3333333333333333703, 0.3333333333333333703, 0.3333333333333333703, 0.3333333333333333703, 0.3333333333333333703, 0.3333333333333333703, 0.3333333333333333703, 0.3333333333333333703, 0.3333333333333333703, 0.3333333333333333703, 0.3333333333333333703, 0.3333333333333333703, 0.3333333333333333703, 0.3333333333333333703, 0.3333333333333333703, 0.3333333333333333703, 0.3333333333333333703, 0.3333333333333333703, 0.3333333333333333703, 0.3333333333333333703, 0.3333333333333333703, 0.3333333333333333703, 0.3333333333333333703, 0.3333333333333333703, 0.3333333333333333703, 0.3333333333333333703, 0.3333333333333333703, 0.3333333333333333703, 0.3333333333333333703, 0.3333333333333333703, 0.3333333333333333703, 0.3333333333333333703, 0.3333333333333333703, 0.3333333333333333703, 0.3333333333333333703, 0.3333333333333333703, 0.3333333333333333703, 0.3333333333333333703, 0.3333333333333333703, 0.3333333333333333703, 0.3333333333333333703, 0.3333333333333333703, 0.3333333333333333703, 0.3333333333333333703, 0.3333333333333333703, 0.3333333333333333703, 0.3333333333333333703, 0.3333333333333333703, 0.3333333333333333703, 0.3333333333333333703, 0.3333333333333333703, 0.3333333333333333703, 0.3333333333333333703, 0.3333333333333333703, 0.3333333333333333703, 0.3333333333333333703, 0.3333333333333333703, 0.3333333333333333703, 0.3333333333333333703, 0.3333333333333333703, 0.3333333333333333703, 0.3333333333333333703, 0.3333333333333333703, 0.3333333333333333703, 0.3333333333333333703, 0.3333333333333333703, 0.3333333333333333703, 0.3333333333333333703, 0.3333333333333333703, 0.3333333333333333703, 0.3333333333333333703, 0.3333333333333333703, 0.3333333333333333703, 0.3333333333333333703, 0.3333333333333333703, 0.3333333333333333703, 0.3333333333333333703, 0.3333333333333333703, 0.3333333333333333703, 0.3333333333333333703, 0.3333333333333333703, 0.3333333333333333703, 0.3333333333333333703, 0.3333333333333333703, 0.3333333333333333703, 0.3333333333333333703, 0.3333333333333333703, 0.3333333333333333703, 0.3333333333333333703, 0.3333333333333333703, 0.3333333333333333703, 0.3333333333333333703, 0.3333333333333333703, 0.3333333333333333703, 0.3333333333333333703, 0.3333333333333333703, 0.3333333333333333703, 0.3333333333333333703, 0.3333333333333333703, 0.3333333333333333703, 0.3333333333333333703, 0.3333333333333333703, 0.3333333333333333703, 0.3333333333333333703, 0.3333333333333333703, 0.3333333333333333703, 0.3333333333333333703, 0.3333333333333333703, 0.3333333333333333703, 0.3333333333333333703, 0.3333333333333333703, 0.3333333333333333703, 0.3333333333333333703, 0.3333333333333333703, 0.3333333333333333703, 0.3333333333333333703, 0.3333333333333333703, 0.3333333333333333703, 0.3333333333333333703, 0.3333333333333333703, 0.3333333333333333703, 0.3333333333333333703, 0.3333333333333333703, 0.3333333333333333703, 0.3333333333333333703, 0.3333333333333333703, 0.3333333333333333703, 0.3333333333333333703, 0.3333333333333333703, 0.3333333333333333703),
 ( 1.000000000000000000, 1.000000000000000000, 1.000000000000000000, 1.000000000000000000, 1.000000000000000000, 1.000000000000000000, 1.000000000000000000, 1.000000000000000000, 1.000000000000000000, 1.000000000000000000, 1.000000000000000000, 1.000000000000000000, 1.000000000000000000, 1.000000000000000000, 1.000000000000000000, 1.000000000000000000, 1.000000000000000000, 1.000000000000000000, 1.000000000000000000, 1.000000000000000000, 1.000000000000000000, 1.000000000000000000, 1.000000000000000000, 1.000000000000000000, 1.000000000000000000, 1.000000000000000000, 1.000000000000000000, 1.000000000000000000, 1.000000000000000000, 1.000000000000000000, 1.000000000000000000, 1.000000000000000000, 1.000000000000000000, 1.000000000000000000, 1.000000000000000000, 1.000000000000000000, 1.000000000000000000, 1.000000000000000000, 1.000000000000000000, 1.000000000000000000, 1.000000000000000000, 1.000000000000000000, 1.000000000000000000, 1.000000000000000000, 1.000000000000000000, 1.000000000000000000, 1.000000000000000000, 1.000000000000000000, 1.000000000000000000, 1.000000000000000000, 1.000000000000000000, 1.000000000000000000, 1.000000000000000000, 1.000000000000000000, 1.000000000000000000, 1.000000000000000000, 1.000000000000000000, 1.000000000000000000, 1.000000000000000000, 1.000000000000000000, 1.000000000000000000, 1.000000000000000000, 1.000000000000000000, 1.000000000000000000, 1.000000000000000000, 1.000000000000000000, 1.000000000000000000, 1.000000000000000000, 1.000000000000000000, 1.000000000000000000, 1.000000000000000000, 1.000000000000000000, 1.000000000000000000, 1.000000000000000000, 1.000000000000000000, 1.000000000000000000, 1.000000000000000000, 1.000000000000000000, 1.000000000000000000, 1.000000000000000000, 1.000000000000000000, 1.000000000000000000, 1.000000000000000000, 1.000000000000000000, 1.000000000000000000, 1.000000000000000000, 1.000000000000000000, 1.000000000000000000, 1.000000000000000000, 1.000000000000000000, 1.000000000000000000, 1.000000000000000000, 1.000000000000000000, 1.000000000000000000, 1.000000000000000000, 1.000000000000000000, 1.000000000000000000, 1.000000000000000000, 1.000000000000000000, 1.000000000000000000, 1.000000000000000000, 1.000000000000000000, 1.000000000000000000, 1.000000000000000000, 1.000000000000000000, 1.000000000000000000, 1.000000000000000000, 1.000000000000000000, 1.000000000000000000, 1.000000000000000000, 1.000000000000000000, 1.000000000000000000, 1.000000000000000000, 1.000000000000000000, 1.000000000000000000, 1.000000000000000000, 1.000000000000000000, 1.000000000000000000, 1.000000000000000000, 1.000000000000000000, 1.000000000000000000, 1.000000000000000000, 1.000000000000000000, 1.000000000000000000, 1.000000000000000000, 1.000000000000000000, 1.000000000000000000, 1.000000000000000000, 1.000000000000000000, 1.000000000000000000, 1.000000000000000000, 1.000000000000000000, 1.000000000000000000, 1.000000000000000000, 1.000000000000000000, 1.000000000000000000, 1.000000000000000000, 1.000000000000000000, 1.000000000000000000, 1.000000000000000000, 1.000000000000000000, 1.000000000000000000, 1.000000000000000000, 1.000000000000000000, 1.000000000000000000, 1.000000000000000000, 1.000000000000000000, 1.000000000000000000, 1.000000000000000000, 1.000000000000000000, 1.000000000000000000, 1.000000000000000000, 1.000000000000000000, 1.000000000000000000, 1.000000000000000000, 1.000000000000000000, 1.000000000000000000, 1.000000000000000000) ) ) 
 REPRESENTATION_ITEM ( '' )  SURFACE ( )  );
#2962=CARTESIAN_POINT ( 'NONE',  ( -35.50000000000000000, -113.9929510916434339, 10.50625754673586876 ) ) ;
#2968=CARTESIAN_POINT ( 'NONE',  ( -34.50000000000000000, -112.9611193698460738, 2.883091707513499635 ) ) ;
#2970=CARTESIAN_POINT ( 'NONE',  ( -39.00000000000000000, -115.9929510916434481, 12.56351784598954779 ) ) ;
#2976=CARTESIAN_POINT ( 'NONE',  ( -35.50000000000000711, -114.3464919575557843, 9.568884482464163455 ) ) ;
#2994=CARTESIAN_POINT ( 'NONE',  ( -36.94073759706868287, -115.0000000000000000, 7.371475545821551734 ) ) ;
#3004=CARTESIAN_POINT ( 'NONE',  ( -35.50000000000000711, -114.6604609523327838, 9.751889438017201428 ) ) ;
#3013=CARTESIAN_POINT ( 'NONE',  ( -38.25557080230232998, -115.9929510916434481, 13.92914543265419525 ) ) ;
#3022=CARTESIAN_POINT ( 'NONE',  ( -36.94073759706868287, -115.9999999999999858, 7.371475545821551734 ) ) ;
#3044=CARTESIAN_POINT ( 'NONE',  ( -34.50000000000000000, -112.0460568841087223, -0.8839717462762063382 ) ) ;
#3047=CARTESIAN_POINT ( 'NONE',  ( -35.87745010033553683, -114.9929510916434339, 14.11371147303761298 ) ) ;
#3049=CARTESIAN_POINT ( 'NONE',  ( -38.00000000000000711, -114.9929510916434339, 12.59102132592608925 ) ) ;
#3051=CARTESIAN_POINT ( 'NONE',  ( -35.07817881376918479, -114.9929510916434339, 13.81802396319203297 ) ) ;
#3065=CARTESIAN_POINT ( 'NONE',  ( -34.83677480945819838, -111.9205845034225462, 7.316024454178450043 ) ) ;
#3067=CARTESIAN_POINT ( 'NONE',  ( -35.50000000000000711, -112.0140978167138712, -0.3122823525984337878 ) ) ;
#3085=CARTESIAN_POINT ( 'NONE',  ( -35.50000000000000000, -112.8920926830253677, 2.874852253704053062 ) ) ;
#3089=CARTESIAN_POINT ( 'NONE',  ( -35.50000000000000711, -114.9929510916434339, 12.60752341388803544 ) ) ;
#3091=CARTESIAN_POINT ( 'NONE',  ( -34.50120407906360498, -113.9929510916434339, 12.67985367974112343 ) ) ;
#3095=CARTESIAN_POINT ( 'NONE',  ( -34.50000000000000000, -113.9929510916434339, 10.52826033068511435 ) ) ;
#3097=CARTESIAN_POINT ( 'NONE',  ( -35.50000000000000711, -114.9922651054798308, 10.46846006712531008 ) ) ;
#3113=CARTESIAN_POINT ( 'NONE',  ( -35.50000000000000000, -113.0140978167138712, -0.4685323525984296800 ) ) ;
#3115=CARTESIAN_POINT ( 'NONE',  ( -37.76916472181487450, -111.9754527089670404, 4.034774454178449155 ) ) ;
#3118=CARTESIAN_POINT ( 'NONE',  ( -35.50000000000000711, -112.0250551866464548, 1.025914454044489332 ) ) ;
#3121=CARTESIAN_POINT ( 'NONE',  ( -37.76916472181487450, -111.9754527089670404, 7.034774454178450931 ) ) ;
#3127=CARTESIAN_POINT ( 'NONE',  ( -34.50000000000000000, -112.4434344552011282, 1.705278471174987986 ) ) ;
#3132=CARTESIAN_POINT ( 'NONE',  ( -35.50000000000000000, -113.9929510916434339, 10.72628538622835670 ) ) ;
#3138=CARTESIAN_POINT ( 'NONE',  ( -34.50000000000000000, -116.0140978167138712, -0.4685323525984310677 ) ) ;
#3139=CARTESIAN_POINT ( 'NONE',  ( -38.69949915733018742, -115.9929510916434481, 13.54034599209165890 ) ) ;
#3162=CARTESIAN_POINT ( 'NONE',  ( -38.02454729103295961, -113.6450488405582462, 4.840225545821551734 ) ) ;
#3171=CARTESIAN_POINT ( 'NONE',  ( -35.50000000000000711, -115.3362660311619692, -1.573728109101206085 ) ) ;
#3174=CARTESIAN_POINT ( 'NONE',  ( -35.50000000000000711, -114.1302255537607095, 9.515717283514957714 ) ) ;
#3179=CARTESIAN_POINT ( 'NONE',  ( -34.50000000000000000, -114.1861579685891712, 9.524983039397698192 ) ) ;
#3184=CARTESIAN_POINT ( 'NONE',  ( -35.80421860361284558, -115.9929510916434481, 14.10650203519841916 ) ) ;
#3185=CARTESIAN_POINT ( 'NONE',  ( -35.50000000000000711, -112.0140978167138712, -0.5622823525984296245 ) ) ;
#3193=CARTESIAN_POINT ( 'NONE',  ( -35.62769128460905677, -112.5438815906447729, 9.808975545821551734 ) ) ;
#3223=CARTESIAN_POINT ( 'NONE',  ( -34.50000000000000000, -115.9927366631908825, 10.47601115720670073 ) ) ;
#3224=DIRECTION ( 'NONE',  ( 0.000000000000000000, 0.000000000000000000, 1.000000000000000000 ) ) ;
#3226=CARTESIAN_POINT ( 'NONE',  ( -37.18750000000006395, -114.9929510916434339, 14.11852480586264846 ) ) ;
#3236=CARTESIAN_POINT ( 'NONE',  ( -40.02454729103296671, -115.1833782841879525, 5.159774454178449155 ) ) ;
#3239=CARTESIAN_POINT ( 'NONE',  ( -35.50000000000000711, -112.6919296022648638, -1.573728109100751116 ) ) ;
#3258=CARTESIAN_POINT ( 'NONE',  ( -34.50000000000000000, -116.9119893297194324, -1.269118781492768688 ) ) ;
#3262=CARTESIAN_POINT ( 'NONE',  ( -35.91854304697313438, -114.9929510916434339, 13.11211614918345703 ) ) ;
#3266=CARTESIAN_POINT ( 'NONE',  ( -34.50000000000000000, -113.9929510916434339, 12.57451923796416260 ) ) ;
#3270=CARTESIAN_POINT ( 'NONE',  ( -34.50000000000000000, -113.9929510916434339, 12.44250253426871033 ) ) ;
#3273=CARTESIAN_POINT ( 'NONE',  ( -35.50000000000000711, -114.9925223117477202, 10.47601618151863079 ) ) ;
#3286=CARTESIAN_POINT ( 'NONE',  ( -35.50000000000000000, -113.0974311500471714, -0.6247823525984269599 ) ) ;
#3288=CARTESIAN_POINT ( 'NONE',  ( -35.02454729103298803, -114.8876895276775087, 1.597274454178448710 ) ) ;
#3295=CARTESIAN_POINT ( 'NONE',  ( -35.50000000000000000, -117.0140978167138854, 0.8752176474015623819 ) ) ;
#3301=CARTESIAN_POINT ( 'NONE',  ( -38.45611840935523418, -115.3723087153909432, 6.566024454178448266 ) ) ;
#3306=CARTESIAN_POINT ( 'NONE',  ( -34.50000000000000000, -113.1256619669233885, 1.895633585076891947 ) ) ;
#3313=CARTESIAN_POINT ( 'NONE',  ( -35.50000000000000000, -113.9929510916436470, 10.50625754673586876 ) ) ;
#3316=CARTESIAN_POINT ( 'NONE',  ( -34.50000000000000000, -116.0141056290913610, -0.5935324770972248976 ) ) ;
#3319=CARTESIAN_POINT ( 'NONE',  ( -35.50000000000000000, -114.3793648455349654, 8.543708532059524074 ) ) ;
#3346=CARTESIAN_POINT ( 'NONE',  ( -37.05926240293131713, -113.0000000000000000, 5.121475545821551734 ) ) ;
#3357=CARTESIAN_POINT ( 'NONE',  ( -35.50000000000000711, -116.0060826362711595, -0.7553032835231661135 ) ) ;
#3360=CARTESIAN_POINT ( 'NONE',  ( -35.50000000000000711, -114.8847986568751907, 10.03799953695244618 ) ) ;
#3363=CARTESIAN_POINT ( 'NONE',  ( -34.50000000000000000, -114.9929510916434339, 11.91443571948719971 ) ) ;
#3366=CARTESIAN_POINT ( 'NONE',  ( -35.50000000000000000, -115.9929510916434481, 10.52826033068511435 ) ) ;
#3367=CARTESIAN_POINT ( 'NONE',  ( -35.50000000000000711, -112.0651520602111191, -0.9469505670458575608 ) ) ;
#3379=CARTESIAN_POINT ( 'NONE',  ( -37.66520193420439711, -114.7490116281687023, 3.058975545821551734 ) ) ;
#3385=ORIENTED_EDGE ( 'NONE', *, *, #20497, .F. ) ;
#3404=CARTESIAN_POINT ( 'NONE',  ( -34.50000000000000000, -113.0974311500471714, -0.6247823525984269599 ) ) ;
#3407=CARTESIAN_POINT ( 'NONE',  ( -34.50000000000000000, -115.9710363517788068, 10.20486393345008835 ) ) ;
#3410=CARTESIAN_POINT ( 'NONE',  ( -38.95206139890800046, -114.9929510916434339, 13.00730889637963728 ) ) ;
#3421=CARTESIAN_POINT ( 'NONE',  ( -35.81662171581204746, -117.0245472910329738, 4.784774454178448266 ) ) ;
#3423=CARTESIAN_POINT ( 'NONE',  ( -35.50000000000000711, -112.0140978167138712, -0.1247823525984259746 ) ) ;
#3440=CARTESIAN_POINT ( 'NONE',  ( -35.50000000000000000, -111.0140821919084715, 0.8283428459075261596 ) ) ;
#3444=CARTESIAN_POINT ( 'NONE',  ( -36.07812499999994316, -114.9929510916434339, 13.11852480586264669 ) ) ;
#3445=CARTESIAN_POINT ( 'NONE',  ( -39.00000000000000000, -113.9929510916434339, 10.50625754673587053 ) ) ;
#3448=CARTESIAN_POINT ( 'NONE',  ( -34.50000000000000000, -113.9929510916434339, 10.51725893871049067 ) ) ;
#3451=CARTESIAN_POINT ( 'NONE',  ( -37.51635661748575501, -114.9929510916434339, 13.11827392651459157 ) ) ;
#3463=CARTESIAN_POINT ( 'NONE',  ( -35.50000000000000000, -113.0140978167143260, -0.6247823525984285142 ) ) ;
#3465=CARTESIAN_POINT ( 'NONE',  ( -34.97545270896703329, -113.2308352781851539, 5.909774454178449155 ) ) ;
#3471=CARTESIAN_POINT ( 'NONE',  ( -35.50000000000000000, -116.9884631899972476, -0.9506101647064282290 ) ) ;
#3474=CARTESIAN_POINT ( 'NONE',  ( -34.97545270896703329, -113.2308352781851539, 5.909774454178449155 ) ) ;
#3481=CARTESIAN_POINT ( 'NONE',  ( -34.50000000000000000, -112.7765286249690035, 1.847058736912741583 ) ) ;
#3487=CARTESIAN_POINT ( 'NONE',  ( -36.12500000000014211, -113.9929510916434339, 13.11852480586264846 ) ) ;
#3490=CARTESIAN_POINT ( 'NONE',  ( -34.50000000000000000, -116.0140978167138712, -0.5622823525984409487 ) ) ;
#3491=CARTESIAN_POINT ( 'NONE',  ( -39.00000000000000000, -115.9929510916434481, 10.85830208992306822 ) ) ;
#3515=CARTESIAN_POINT ( 'NONE',  ( -36.33479806579560289, -113.2509883718313262, 6.808975545821551734 ) ) ;
#3524=CARTESIAN_POINT ( 'NONE',  ( -35.50000000000000711, -114.1807644833817648, -1.624782352598427959 ) ) ;
#3527=CARTESIAN_POINT ( 'NONE',  ( -35.50000000000000711, -114.9925223117477202, 10.47601618151863079 ) ) ;
#3530=CARTESIAN_POINT ( 'NONE',  ( -34.50000000000000000, -114.9929517792218689, 10.50900788599415314 ) ) ;
#3536=CARTESIAN_POINT ( 'NONE',  ( -35.50000000000000000, -114.2265172349312508, 8.519938377296172760 ) ) ;
#3547=CARTESIAN_POINT ( 'NONE',  ( -35.99999999999999289, -114.0592624029313242, 1.503524454178448710 ) ) ;
#3556=CARTESIAN_POINT ( 'NONE',  ( -34.02454729103298092, -115.3019030900506294, 7.597274454178449155 ) ) ;
#3571=CARTESIAN_POINT ( 'NONE',  ( -34.50000000000000000, -114.8474311500471572, -0.6247823525984269599 ) ) ;
#3574=CARTESIAN_POINT ( 'NONE',  ( -34.50000000000000000, -115.9056129652226872, 9.909279992139808257 ) ) ;
#3579=CARTESIAN_POINT ( 'NONE',  ( -37.46874999999996447, -114.9929510916434339, 14.11852480586264846 ) ) ;
#3589=CARTESIAN_POINT ( 'NONE',  ( -38.18337828418796676, -117.0245472910329738, 7.465225545821552622 ) ) ;
#3591=CARTESIAN_POINT ( 'NONE',  ( -35.50000000000000711, -115.2732872103912030, -1.592823285204062911 ) ) ;
#3604=CARTESIAN_POINT ( 'NONE',  ( -39.02454729103295961, -113.2308352781851397, 3.340225545821551734 ) ) ;
#3611=CARTESIAN_POINT ( 'NONE',  ( -35.50000000000000000, -116.6134300264884445, -1.853877267570539944 ) ) ;
#3616=CARTESIAN_POINT ( 'NONE',  ( -36.06250000000002132, -114.9929510916434339, 13.11852480586264669 ) ) ;
#3618=CARTESIAN_POINT ( 'NONE',  ( -39.00000000000000000, -113.9929510916434339, 12.39849696637031151 ) ) ;
#3624=CARTESIAN_POINT ( 'NONE',  ( -36.15625000000007816, -113.9929510916434339, 14.11852480586265024 ) ) ;
#3626=CARTESIAN_POINT ( 'NONE',  ( -35.50000000000000711, -114.9929510916434339, 12.59102132592610523 ) ) ;
#3631=CARTESIAN_POINT ( 'NONE',  ( -35.50000102263782509, -114.9929510916434339, 12.62466071271731316 ) ) ;
#3640=CARTESIAN_POINT ( 'NONE',  ( -35.50000000000000000, -115.0140978167138712, -0.3122823525984416149 ) ) ;
#3642=CARTESIAN_POINT ( 'NONE',  ( -36.94073759706868287, -112.0000000000000142, 2.628524454178448710 ) ) ;
#3644=CARTESIAN_POINT ( 'NONE',  ( -38.99999999999999289, -113.9407375970686900, 3.753524454178449155 ) ) ;
#3647=CARTESIAN_POINT ( 'NONE',  ( -35.50000000000000000, -114.6807644833805000, -2.624782352598442614 ) ) ;
#3657=CARTESIAN_POINT ( 'NONE',  ( -34.50000000000000000, -112.0140900043366088, -0.5935324770972457697 ) ) ;
#3664=CARTESIAN_POINT ( 'NONE',  ( -37.46874999999995737, -113.9929510916434339, 13.11852480586264846 ) ) ;
#3667=CARTESIAN_POINT ( 'NONE',  ( -35.99181955245763476, -113.9929510916434339, 13.11847460610632510 ) ) ;
#3668=CARTESIAN_POINT ( 'NONE',  ( -35.50000000000000000, -115.9929510916434481, 10.61627146648203990 ) ) ;
#3684=CIRCLE ( 'NONE', #16864, 0.5000000000000004441 ) ;
#3691=CARTESIAN_POINT ( 'NONE',  ( -37.99999999999998579, -114.0592624029313242, 7.746475545821553510 ) ) ;
#3701=CARTESIAN_POINT ( 'NONE',  ( -35.50000000000000711, -114.9929510916434339, 10.72628538622835670 ) ) ;
#3705=CARTESIAN_POINT ( 'NONE',  ( -34.50000000000000000, -114.2305202833893816, 9.534416457224700991 ) ) ;
#3709=CARTESIAN_POINT ( 'NONE',  ( -35.50000000000000000, -115.9056129652226872, 9.909279992139808257 ) ) ;
#3710=CARTESIAN_POINT ( 'NONE',  ( -35.50000000000000711, -112.4434344552011282, 1.705278471174987986 ) ) ;
#3715=CIRCLE ( 'NONE', #5469, 0.5000000000000004441 ) ;
#3720=CARTESIAN_POINT ( 'NONE',  ( -37.05926240293133134, -115.0000000000000000, 1.878524454178448710 ) ) ;
#3729=CARTESIAN_POINT ( 'NONE',  ( -34.00000000000000000, -114.0592624029313242, 9.003524454178446490 ) ) ;
#3747=CARTESIAN_POINT ( 'NONE',  ( -34.50000000000000000, -112.9415908020655195, 1.873661708251232572 ) ) ;
#3751=CARTESIAN_POINT ( 'NONE',  ( -34.50000000000000000, -115.9792481177720731, 10.26484292309424795 ) ) ;
#3754=CARTESIAN_POINT ( 'NONE',  ( -39.00000000000000711, -114.9929510916434339, 12.17846912687782179 ) ) ;
#3763=CARTESIAN_POINT ( 'NONE',  ( -39.99999999999999289, -114.0592624029313242, 4.746475545821549957 ) ) ;
#3766=CARTESIAN_POINT ( 'NONE',  ( -35.50000000000000711, -112.0141059978162019, -0.6575071456984691309 ) ) ;
#3782=CARTESIAN_POINT ( 'NONE',  ( -37.05926240293131713, -112.0000000000000142, 5.121475545821551734 ) ) ;
#3788=CARTESIAN_POINT ( 'NONE',  ( -35.50000000000000000, -116.9980674558286040, -0.8858242144478970514 ) ) ;
#3792=CARTESIAN_POINT ( 'NONE',  ( -37.52044295795950291, -114.9929510916434339, 13.11812344617477244 ) ) ;
#3794=CARTESIAN_POINT ( 'NONE',  ( -37.46093750000000711, -113.9929510916434339, 14.11852480586265024 ) ) ;
#3798=CARTESIAN_POINT ( 'NONE',  ( -37.62254989966453422, -113.9929510916434339, 14.11371147303758278 ) ) ;
#3801=CARTESIAN_POINT ( 'NONE',  ( -35.99386409314529800, -114.9929510916434339, 13.11852378322482515 ) ) ;
#3808=CARTESIAN_POINT ( 'NONE',  ( -35.50000000000000711, -114.9928438774171582, 10.49113435197128652 ) ) ;
#3816=CARTESIAN_POINT ( 'NONE',  ( -35.50000000000000000, -113.8474311500459777, -0.6247823525984269599 ) ) ;
#3819=CARTESIAN_POINT ( 'NONE',  ( -38.37230871539094323, -112.5438815906447729, 5.441024454178449155 ) ) ;
#3821=CARTESIAN_POINT ( 'NONE',  ( -36.23083527818512550, -116.0245472910329880, 1.784774454178448932 ) ) ;
#3824=CARTESIAN_POINT ( 'NONE',  ( -35.50000000000000711, -113.6807644833805995, -1.624782352598427959 ) ) ;
#3836=CARTESIAN_POINT ( 'NONE',  ( -34.50000000000000000, -112.6919296022648638, -1.573728109100751116 ) ) ;
#3843=CARTESIAN_POINT ( 'NONE',  ( -37.50818044754229419, -113.9929510916434339, 13.11847460610629845 ) ) ;
#3844=CARTESIAN_POINT ( 'NONE',  ( -34.50000000000000000, -113.6318576702834804, 1.956056246348823580 ) ) ;
#3846=CARTESIAN_POINT ( 'NONE',  ( -35.50000000000000000, -113.9929510916434339, 10.85830208992344303 ) ) ;
#3847=CARTESIAN_POINT ( 'NONE',  ( -35.50000000000000000, -115.9929524668003182, 10.51038305125561401 ) ) ;
#3871=CARTESIAN_POINT ( 'NONE',  ( -34.50000000000000000, -117.0140978167138854, -0.3747823525984421145 ) ) ;
#3875=CARTESIAN_POINT ( 'NONE',  ( -37.66520193420439000, -113.2509883718312977, 2.441024454178448710 ) ) ;
#3879=CARTESIAN_POINT ( 'NONE',  ( -35.50000000000000000, -115.0140978167138428, -0.6247823525979866455 ) ) ;
#3881=CARTESIAN_POINT ( 'NONE',  ( -35.50000000000000711, -116.0140978167138712, -0.4685323525984310677 ) ) ;
#3885=CARTESIAN_POINT ( 'NONE',  ( -35.51597953369718397, -114.9929510916434339, 12.74811950270164473 ) ) ;
#3891=CARTESIAN_POINT ( 'NONE',  ( -34.50000000000000000, -114.9929510916434339, 11.73841344789270202 ) ) ;
#3895=CARTESIAN_POINT ( 'NONE',  ( -35.50000000000000000, -114.1371041221139109, 8.509266650872710613 ) ) ;
#3896=CARTESIAN_POINT ( 'NONE',  ( -35.50000000000000711, -112.0141053790792114, 0.9054673897245171243 ) ) ;
#3909=CARTESIAN_POINT ( 'NONE',  ( -36.52652403469559061, -114.9754527089670262, 8.777725545821549957 ) ) ;
#3920=CARTESIAN_POINT ( 'NONE',  ( -39.07941549657749647, -116.1632251905417803, 9.058975545821549957 ) ) ;
#3937=CARTESIAN_POINT ( 'NONE',  ( -34.50000000000000000, -114.3474311500471572, -0.6247823525984269599 ) ) ;
#3942=CARTESIAN_POINT ( 'NONE',  ( -34.50000000000000000, -115.1342778146718473, 8.846135899190283425 ) ) ;
#3945=CARTESIAN_POINT ( 'NONE',  ( -39.00000000000000711, -114.9929510916434339, 12.44250253426874941 ) ) ;
#3957=CARTESIAN_POINT ( 'NONE',  ( -36.94073759706868287, -116.9999999999999858, 4.371475545821550845 ) ) ;
#3959=CARTESIAN_POINT ( 'NONE',  ( -35.50000000000000000, -113.0140978167137717, 0.8903425666012282358 ) ) ;
#3972=CARTESIAN_POINT ( 'NONE',  ( -36.94073759706868287, -115.9999999999999858, 5.871475545821550845 ) ) ;
#3976=CARTESIAN_POINT ( 'NONE',  ( -35.50000000000000000, -111.0140978167138570, -0.5622823525984297355 ) ) ;
#3979=CARTESIAN_POINT ( 'NONE',  ( -37.66108410722335265, -114.9929510916434339, 13.09299768411426790 ) ) ;
#3981=CARTESIAN_POINT ( 'NONE',  ( -38.69949915733018742, -113.9929510916434339, 13.54034599209165890 ) ) ;
#3984=CARTESIAN_POINT ( 'NONE',  ( -38.98797722933581866, -113.9929510916434339, 12.81430620224974959 ) ) ;
#3987=CARTESIAN_POINT ( 'NONE',  ( -35.50000000000000711, -114.9929510916434339, 12.44250253426871033 ) ) ;
#3996=CARTESIAN_POINT ( 'NONE',  ( -35.50000000000000711, -114.9929510916434339, 10.52000928670414126 ) ) ;
#3999=CARTESIAN_POINT ( 'NONE',  ( -35.02454729103298803, -114.8876895276775087, 3.097274454178448710 ) ) ;
#4003=CARTESIAN_POINT ( 'NONE',  ( -34.50000000000000000, -113.0601156079281253, 0.8807106166081309917 ) ) ;
#4005=CARTESIAN_POINT ( 'NONE',  ( -38.97545270896704039, -113.1123104723225197, 8.347274454178448266 ) ) ;
#4008=CARTESIAN_POINT ( 'NONE',  ( -35.00000000000000000, -114.0592624029313242, 4.503524454178448266 ) ) ;
#4011=CARTESIAN_POINT ( 'NONE',  ( -35.50000000000000711, -113.8474311500459777, -1.624782352598427959 ) ) ;
#4020=CARTESIAN_POINT ( 'NONE',  ( -34.50000000000000000, -113.2372261171341563, 2.916049522752222511 ) ) ;
#4021=CARTESIAN_POINT ( 'NONE',  ( -35.50000000000000711, -112.8655373925166572, 1.864575885149403423 ) ) ;
#4027=CARTESIAN_POINT ( 'NONE',  ( -36.00585935943765747, -113.9929510916434339, 13.11852578240983291 ) ) ;
#4031=CARTESIAN_POINT ( 'NONE',  ( -35.99386409314529800, -113.9929510916434339, 13.11852378322482515 ) ) ;
#4032=CARTESIAN_POINT ( 'NONE',  ( -35.50000000000000000, -115.9929510916434481, 12.56351784598954424 ) ) ;
#4043=CARTESIAN_POINT ( 'NONE',  ( -35.50000000000000711, -112.9185811467682754, 1.870920967077121411 ) ) ;
#4047=CARTESIAN_POINT ( 'NONE',  ( -35.69809690994938478, -111.0245472910330022, 2.722274454178449155 ) ) ;
#4054=CARTESIAN_POINT ( 'NONE',  ( -34.50000000000000000, -113.1807644833805426, -2.624782352598442614 ) ) ;
#4058=CARTESIAN_POINT ( 'NONE',  ( -38.02454729103296671, -114.3549511594417396, 3.659774454178448710 ) ) ;
#4063=CARTESIAN_POINT ( 'NONE',  ( -34.50000000000000000, -113.0256022645180707, 0.8765908897032291813 ) ) ;
#4067=DIRECTION ( 'NONE',  ( 0.000000000000000000, 0.000000000000000000, 1.000000000000000000 ) ) ;
#4070=CARTESIAN_POINT ( 'NONE',  ( -35.50000000000000711, -114.9929510916434339, 11.73841344789270202 ) ) ;
#4075=CARTESIAN_POINT ( 'NONE',  ( -37.46093750000000711, -114.9929510916434339, 14.11852480586264846 ) ) ;
#4081=CARTESIAN_POINT ( 'NONE',  ( -35.50000000000000000, -115.6492853190479337, 9.359470924297957239 ) ) ;
#4082=CARTESIAN_POINT ( 'NONE',  ( -35.50000000000000711, -112.6919296022648638, -1.573728109100751116 ) ) ;
#4093=CARTESIAN_POINT ( 'NONE',  ( -37.47347596530441649, -113.0245472910329880, 8.027725545821551734 ) ) ;
#4100=CARTESIAN_POINT ( 'NONE',  ( -35.81662171581203324, -110.9754527089670546, 6.715225545821551734 ) ) ;
#4116=CARTESIAN_POINT ( 'NONE',  ( -34.50000000000000000, -115.0140978167137860, -0.6411448143358557950 ) ) ;
#4119=CARTESIAN_POINT ( 'NONE',  ( -37.43749999999998579, -115.9929510916434481, 14.11852480586265024 ) ) ;
#4123=CARTESIAN_POINT ( 'NONE',  ( -37.54906985245724371, -114.9929510916434339, 14.11777216781844579 ) ) ;
#4131=CARTESIAN_POINT ( 'NONE',  ( -39.07941549657749647, -116.1632251905417803, 3.058975545821551734 ) ) ;
#4133=CARTESIAN_POINT ( 'NONE',  ( -35.50000000000000000, -113.0140978167138996, -0.6247823525984302906 ) ) ;
#4142=CARTESIAN_POINT ( 'NONE',  ( -38.45611840935523418, -112.6276912846090568, 4.933975545821551734 ) ) ;
#4149=CARTESIAN_POINT ( 'NONE',  ( -35.50000000000000000, -114.9515981487115823, -2.624803185604625000 ) ) ;
#4156=CARTESIAN_POINT ( 'NONE',  ( -34.50000000000000000, -114.1302255537607095, 9.515717283514957714 ) ) ;
#4158=CARTESIAN_POINT ( 'NONE',  ( -36.87500000000098055, -114.9929510916434339, 13.11852480586264669 ) ) ;
#4161=CARTESIAN_POINT ( 'NONE',  ( -36.07812499999994316, -113.9929510916434339, 14.11852480586265024 ) ) ;
#4163=CARTESIAN_POINT ( 'NONE',  ( -37.46093750000000711, -114.9929510916434339, 13.11852480586264669 ) ) ;
#4169=CARTESIAN_POINT ( 'NONE',  ( -35.50160444427493189, -114.9929510916434339, 12.65937477241749853 ) ) ;
#4177=CARTESIAN_POINT ( 'NONE',  ( -34.50000000000000000, -113.7503824761461004, 0.9631051547057219997 ) ) ;
#4179=CARTESIAN_POINT ( 'NONE',  ( -35.02454729103298803, -114.8876895276775087, 7.597274454178450931 ) ) ;
#4181=CARTESIAN_POINT ( 'NONE',  ( -37.88768952767750164, -115.9754527089670262, 6.472274454178450043 ) ) ;
#4185=CARTESIAN_POINT ( 'NONE',  ( -35.50000000000000711, -113.1807644833805426, -1.624782352598427959 ) ) ;
#4190=SURFACE_STYLE_USAGE ( .BOTH. , #34607 ) ;
#4194=CARTESIAN_POINT ( 'NONE',  ( -34.50000000000000000, -116.0060826362711595, -0.7553032835231661135 ) ) ;
#4195=CARTESIAN_POINT ( 'NONE',  ( -35.50000000000000711, -112.1859307030124739, 1.448610958621386224 ) ) ;
#4204=CARTESIAN_POINT ( 'NONE',  ( -37.46093750000000711, -113.9929510916434339, 13.11852480586264846 ) ) ;
#4206=EDGE_CURVE ( 'NONE', #34373, #35474, #34924, .T. ) ;
#4207=CARTESIAN_POINT ( 'NONE',  ( -37.18750000000004974, -113.9929510916434339, 13.11852480586264846 ) ) ;
#4209=CARTESIAN_POINT ( 'NONE',  ( -35.50100302244945993, -115.9929510916434481, 12.65121853911337446 ) ) ;
#4220=CARTESIAN_POINT ( 'NONE',  ( -35.50000000000000711, -113.6807644833805995, -1.624782352598427959 ) ) ;
#4228=CARTESIAN_POINT ( 'NONE',  ( -34.50000000000000000, -116.9501796819249222, -1.143161139954000260 ) ) ;
#4232=CARTESIAN_POINT ( 'NONE',  ( -37.47347596530441649, -114.9754527089670262, 3.472274454178448710 ) ) ;
#4236=CARTESIAN_POINT ( 'NONE',  ( -35.50000000000000000, -115.0140978167138712, -0.6247823525985405357 ) ) ;
#4243=CARTESIAN_POINT ( 'NONE',  ( -35.50000000000000711, -114.9929510916434339, 12.60752341388803544 ) ) ;
#4247=CARTESIAN_POINT ( 'NONE',  ( -36.62499999999902656, -114.9929510916434339, 14.11852480586264846 ) ) ;
#4251=CARTESIAN_POINT ( 'NONE',  ( -35.50000000000000000, -115.9929510916434481, 12.56351784598954424 ) ) ;
#4252=CARTESIAN_POINT ( 'NONE',  ( -35.50000000000000711, -113.3474311500483935, -1.624782352598427959 ) ) ;
#4262=CARTESIAN_POINT ( 'NONE',  ( -37.05926240293131713, -113.0000000000000000, 8.121475545821549957 ) ) ;
#4274=CARTESIAN_POINT ( 'NONE',  ( -39.07941549657749647, -116.1632251905417803, 7.558975545821551734 ) ) ;
#4292=CARTESIAN_POINT ( 'NONE',  ( -34.50075263804418313, -115.9929510916434481, 12.66759465831979981 ) ) ;
#4296=CARTESIAN_POINT ( 'NONE',  ( -34.50000000000000000, -115.9382890315277308, 10.02636389016632812 ) ) ;
#4304=CARTESIAN_POINT ( 'NONE',  ( -39.97545270896702618, -115.3019030900506152, 6.152725545821551734 ) ) ;
#4306=CARTESIAN_POINT ( 'NONE',  ( -35.50000000000000000, -113.0140978167138712, -0.6247823525988807081 ) ) ;
#4319=CARTESIAN_POINT ( 'NONE',  ( -39.02454729103295961, -113.2308352781851397, 4.840225545821550845 ) ) ;
#4325=CARTESIAN_POINT ( 'NONE',  ( -35.50000000000000000, -115.0631849411758196, -2.624765990393648885 ) ) ;
#4331=CARTESIAN_POINT ( 'NONE',  ( -34.50000000000000000, -114.9929510916434339, 11.91443571948719971 ) ) ;
#4333=CARTESIAN_POINT ( 'NONE',  ( -36.06250000000002132, -114.9929510916434339, 13.11852480586264669 ) ) ;
#4335=CARTESIAN_POINT ( 'NONE',  ( -36.03906250000000000, -113.9929510916434339, 14.11852480586265024 ) ) ;
#4337=CARTESIAN_POINT ( 'NONE',  ( -37.99599240977853754, -114.9929510916434339, 12.68378527132499478 ) ) ;
#4345=CARTESIAN_POINT ( 'NONE',  ( -35.50640865667918433, -114.9929510916434339, 12.69998175888958514 ) ) ;
#4353=CARTESIAN_POINT ( 'NONE',  ( -34.50000000000000000, -113.0140978167137860, -0.6247823525984055326 ) ) ;
#4355=CARTESIAN_POINT ( 'NONE',  ( -37.76916472181487450, -111.9754527089670404, 7.034774454178450931 ) ) ;
#4357=CARTESIAN_POINT ( 'NONE',  ( -37.88768952767750164, -115.9754527089670262, 7.972274454178450043 ) ) ;
#4359=CARTESIAN_POINT ( 'NONE',  ( -35.50000000000000711, -116.0060826362711595, -0.7553032835231661135 ) ) ;
#4368=CARTESIAN_POINT ( 'NONE',  ( -34.50000000000000000, -112.9611193698460738, 2.883091707513499635 ) ) ;
#4369=CARTESIAN_POINT ( 'NONE',  ( -35.50000000000000711, -112.0154707866092707, 0.9357013553229778235 ) ) ;
#4378=CARTESIAN_POINT ( 'NONE',  ( -34.50000000000000000, -113.9929510916433344, 10.50625754673586876 ) ) ;
#4380=CARTESIAN_POINT ( 'NONE',  ( -35.50000000000000000, -113.9929510916434339, 12.59652202191340464 ) ) ;
#4381=CARTESIAN_POINT ( 'NONE',  ( -35.50000000000000000, -115.7766462221073454, 9.569741527169023598 ) ) ;
#4392=CARTESIAN_POINT ( 'NONE',  ( -35.50000000000000711, -114.9724313160460696, -1.624792769101446765 ) ) ;
#4396=CARTESIAN_POINT ( 'NONE',  ( -35.50000000000000711, -114.0650276068786582, 9.507762098804159123 ) ) ;
#4403=CARTESIAN_POINT ( 'NONE',  ( -34.50000000000000000, -116.9119893297194324, -1.269118781492768688 ) ) ;
#4407=CARTESIAN_POINT ( 'NONE',  ( -36.94073759706866156, -113.0000000000000000, 4.128524454178449155 ) ) ;
#4414=CARTESIAN_POINT ( 'NONE',  ( -35.50000000000000000, -115.0140978167138712, -0.1247823525984438492 ) ) ;
#4419=CARTESIAN_POINT ( 'NONE',  ( -35.50000000000000711, -114.9929510916434339, 10.59426868253284226 ) ) ;
#4423=CARTESIAN_POINT ( 'NONE',  ( -36.06250000000002132, -114.9929510916434339, 14.11852480586264846 ) ) ;
#4428=CARTESIAN_POINT ( 'NONE',  ( -35.95915003344518368, -115.9929510916434481, 13.11692036158763308 ) ) ;
#4429=CARTESIAN_POINT ( 'NONE',  ( -35.50000000000000711, -116.0140978167138712, 0.0002176474015577116276 ) ) ;
#4444=CARTESIAN_POINT ( 'NONE',  ( -36.02454729103298092, -114.4734759653044307, 3.097274454178448710 ) ) ;
#4451=CARTESIAN_POINT ( 'NONE',  ( -35.00000000000000000, -114.0000000000000853, 2.000000000000001776 ) ) ;
#4453=CARTESIAN_POINT ( 'NONE',  ( -40.02454729103296671, -112.8166217158120332, 6.340225545821551734 ) ) ;
#4476=CARTESIAN_POINT ( 'NONE',  ( -35.24442919769867899, -115.9929510916434481, 13.92914543265605509 ) ) ;
#4480=CARTESIAN_POINT ( 'NONE',  ( -35.54388159064475872, -112.6276912846090568, 7.316024454178449155 ) ) ;
#4482=CARTESIAN_POINT ( 'NONE',  ( -34.50000000000000000, -115.9920935318519923, 10.44577481630138749 ) ) ;
#4494=CARTESIAN_POINT ( 'NONE',  ( -37.88768952767750875, -112.0245472910329880, 5.027725545821550845 ) ) ;
#4498=CARTESIAN_POINT ( 'NONE',  ( -35.50000000000000000, -113.0140978167138712, -0.6247823525983134951 ) ) ;
#4517=CARTESIAN_POINT ( 'NONE',  ( -35.50000000000000711, -112.0140978167138712, 0.0002176474015661141945 ) ) ;
#4522=CARTESIAN_POINT ( 'NONE',  ( -38.00000000000000711, -114.9929510916434339, 11.91443571948719615 ) ) ;
#4526=CARTESIAN_POINT ( 'NONE',  ( -34.50075263804418313, -114.9929510916434339, 12.66759465831979981 ) ) ;
#4528=CARTESIAN_POINT ( 'NONE',  ( -36.07812499999994316, -114.9929510916434339, 13.11852480586264669 ) ) ;
#4530=CARTESIAN_POINT ( 'NONE',  ( -34.50000000000000000, -114.9925223117477202, 10.47601618151863079 ) ) ;
#4532=CARTESIAN_POINT ( 'NONE',  ( -37.97447287825094975, -114.9929510916434339, 12.77960891308616809 ) ) ;
#4538=CARTESIAN_POINT ( 'NONE',  ( -36.06250000000002132, -114.9929510916434339, 13.11852480586264669 ) ) ;
#4541=CARTESIAN_POINT ( 'NONE',  ( -37.88768952767750164, -115.9754527089670262, 3.472274454178448266 ) ) ;
#4548=CARTESIAN_POINT ( 'NONE',  ( -34.50000000000000000, -113.0140978167138712, -0.4997823525984338988 ) ) ;
#4552=CARTESIAN_POINT ( 'NONE',  ( -35.02454729103298803, -114.8876895276775087, 7.597274454178450931 ) ) ;
#4562=CARTESIAN_POINT ( 'NONE',  ( -34.50000000000000000, -115.5178116849130276, -1.498529437126731034 ) ) ;
#4569=CARTESIAN_POINT ( 'NONE',  ( -34.50000000000000000, -113.9929510916434623, 10.50625754673586876 ) ) ;
#4571=CARTESIAN_POINT ( 'NONE',  ( -38.00000000000000711, -113.9929510916434339, 10.85830208992306822 ) ) ;
#4572=CARTESIAN_POINT ( 'NONE',  ( -36.03125000000003553, -115.9929510916434481, 13.11852480586264846 ) ) ;
#4581=CARTESIAN_POINT ( 'NONE',  ( -35.50000000000000711, -112.0140978167138712, -0.3747823525984256832 ) ) ;
#4589=CARTESIAN_POINT ( 'NONE',  ( -34.50000000000000000, -111.4147656069378058, -1.853877267569947529 ) ) ;
#4593=CARTESIAN_POINT ( 'NONE',  ( -37.05926240293133134, -115.0000000000000000, 3.378524454178448710 ) ) ;
#4599=CARTESIAN_POINT ( 'NONE',  ( -35.50000000000000000, -115.0140978167138712, -0.3122823525984416149 ) ) ;
#4603=CARTESIAN_POINT ( 'NONE',  ( -35.50000000000000000, -113.9465028010160381, 10.50071319044726081 ) ) ;
#4606=CARTESIAN_POINT ( 'NONE',  ( -35.61121590948313553, -114.9929510916434339, 14.07058620477040733 ) ) ;
#4614=CARTESIAN_POINT ( 'NONE',  ( -35.52552712174883709, -115.9929510916434481, 12.77960891308624625 ) ) ;
#4615=CARTESIAN_POINT ( 'NONE',  ( -35.50000000000000711, -112.8511839106603247, -1.611965039240275122 ) ) ;
#4625=CARTESIAN_POINT ( 'NONE',  ( -36.33479806579561000, -114.7490116281687165, 6.191024454178448266 ) ) ;
#4633=CARTESIAN_POINT ( 'NONE',  ( -34.83677480945821259, -116.0794154965774965, 8.683975545821549957 ) ) ;
#4656=CARTESIAN_POINT ( 'NONE',  ( -36.00976557831293690, -115.9929510916434481, 14.11852773550420359 ) ) ;
#4658=CARTESIAN_POINT ( 'NONE',  ( -36.23083527818513261, -116.0245472910329880, 7.784774454178449155 ) ) ;
#4660=CARTESIAN_POINT ( 'NONE',  ( -34.50000000000000000, -115.1342778146718473, 8.846135899190283425 ) ) ;
#4670=CARTESIAN_POINT ( 'NONE',  ( -35.00000000000000000, -113.9407375970686900, 2.496475545821551290 ) ) ;
#4673=CARTESIAN_POINT ( 'NONE',  ( -35.50000000000000000, -113.9344536409997630, 0.9850770315317123327 ) ) ;
#4688=CARTESIAN_POINT ( 'NONE',  ( -35.50000000000000711, -112.0157046079661995, -0.6902086197697556713 ) ) ;
#4698=CARTESIAN_POINT ( 'NONE',  ( -34.50000000000000000, -113.0106174888879877, 1.881901162060937827 ) ) ;
#4699=CARTESIAN_POINT ( 'NONE',  ( -34.50000000000000000, -114.1861579685891712, 9.524983039397698192 ) ) ;
#4701=CARTESIAN_POINT ( 'NONE',  ( -35.83891589277640577, -114.9929510916434339, 13.09299768411358222 ) ) ;
#4703=CARTESIAN_POINT ( 'NONE',  ( -39.00000000000000000, -113.9929510916434339, 12.50851088611646311 ) ) ;
#4706=CARTESIAN_POINT ( 'NONE',  ( -37.54084996655477369, -114.9929510916434339, 13.11692036158760466 ) ) ;
#4712=CARTESIAN_POINT ( 'NONE',  ( -37.99899697755054717, -114.9929510916434339, 12.65121853911336736 ) ) ;
#4714=CARTESIAN_POINT ( 'NONE',  ( -36.94073759706868287, -112.0000000000000142, 7.128524454178449155 ) ) ;
#4722=CARTESIAN_POINT ( 'NONE',  ( -36.11231047232249125, -112.0245472910329880, 8.722274454178448266 ) ) ;
#4735=CARTESIAN_POINT ( 'NONE',  ( -34.50000000000000000, -111.0397324434303101, -0.9506101647064429949 ) ) ;
#4741=CARTESIAN_POINT ( 'NONE',  ( -35.50000000000000711, -114.3464919575557843, 9.568884482464163455 ) ) ;
#4742=CARTESIAN_POINT ( 'NONE',  ( -38.00000000000000711, -113.9929510916434339, 12.60752341388803721 ) ) ;
#4745=CARTESIAN_POINT ( 'NONE',  ( -37.99899697755054717, -113.9929510916434339, 12.65121853911336913 ) ) ;
#4746=CARTESIAN_POINT ( 'NONE',  ( -37.58145695302688694, -115.9929510916434481, 13.11211614918362756 ) ) ;
#4755=CARTESIAN_POINT ( 'NONE',  ( -35.50000000000000711, -112.0140900043112282, 0.8439677466545482121 ) ) ;
#4757=CARTESIAN_POINT ( 'NONE',  ( -35.50000000000000711, -114.8211182053456838, 9.932864235516914775 ) ) ;
#4763=CARTESIAN_POINT ( 'NONE',  ( -35.50000000000000000, -111.0140978167138570, -0.4685323525984296800 ) ) ;
#4767=CARTESIAN_POINT ( 'NONE',  ( -36.64504884055823908, -115.0245472910329880, 7.784774454178449155 ) ) ;
#4773=CARTESIAN_POINT ( 'NONE',  ( -34.50000000000000000, -113.0349311500474982, -0.6247823525985715110 ) ) ;
#4776=CARTESIAN_POINT ( 'NONE',  ( -37.62959469683911351, -114.9929510916434339, 13.10254527216511633 ) ) ;
#4779=CARTESIAN_POINT ( 'NONE',  ( -34.50000000000000000, -112.0141053790792114, 0.9054673897245171243 ) ) ;
#4780=CARTESIAN_POINT ( 'NONE',  ( -35.87745010033553683, -114.9929510916434339, 14.11371147303761298 ) ) ;
#4786=CARTESIAN_POINT ( 'NONE',  ( -37.18750000000004974, -115.9929510916434481, 13.11852480586264846 ) ) ;
#4787=CARTESIAN_POINT ( 'NONE',  ( -35.50000000000000711, -113.6807644833805995, -1.624782352598427959 ) ) ;
#4796=CARTESIAN_POINT ( 'NONE',  ( -37.47347596530441649, -114.9754527089670262, 3.472274454178448710 ) ) ;
#4807=CARTESIAN_POINT ( 'NONE',  ( -36.23083527818512550, -111.9754527089670404, 3.715225545821550845 ) ) ;
#4826=CARTESIAN_POINT ( 'NONE',  ( -35.54388159064475872, -112.6276912846090568, 8.816024454178448266 ) ) ;
#4827=CARTESIAN_POINT ( 'NONE',  ( -34.49999793727135966, -115.9929510916434481, 12.61164896875036767 ) ) ;
#4836=CARTESIAN_POINT ( 'NONE',  ( -37.76916472181486739, -116.0245472910329880, 5.965225545821550845 ) ) ;
#4846=ORIENTED_EDGE ( 'NONE', *, *, #22366, .F. ) ;
#4849=CARTESIAN_POINT ( 'NONE',  ( -38.97545270896704039, -114.8876895276775087, 9.152725545821553510 ) ) ;
#4856=CARTESIAN_POINT ( 'NONE',  ( -35.50000000000000711, -112.0140900043112282, 0.8439677466545482121 ) ) ;
#4863=CARTESIAN_POINT ( 'NONE',  ( -34.50000000000000000, -112.0250551866464548, 1.025914454044489332 ) ) ;
#4864=CARTESIAN_POINT ( 'NONE',  ( -34.50481333282507279, -114.9929510916434339, 12.74107470552716492 ) ) ;
#4866=CARTESIAN_POINT ( 'NONE',  ( -37.99599240977853754, -114.9929510916434339, 12.68378527132499478 ) ) ;
#4868=CARTESIAN_POINT ( 'NONE',  ( -39.00000000000000000, -113.9929510916434339, 10.85830208992306822 ) ) ;
#4869=DIRECTION ( 'NONE',  ( 0.000000000000000000, 0.9929510916431029122, -0.1185248058626136303 ) ) ;
#4871=CARTESIAN_POINT ( 'NONE',  ( -38.00000000000000711, -114.9929510916434339, 11.21034663311206181 ) ) ;
#4877=CARTESIAN_POINT ( 'NONE',  ( -37.99599240977853754, -114.9929510916434339, 12.68378527132499478 ) ) ;
#4879=CARTESIAN_POINT ( 'NONE',  ( -35.00000000000000000, -114.0592624029313242, 9.003524454178448266 ) ) ;
#4890=CARTESIAN_POINT ( 'NONE',  ( -36.94073759706866156, -111.0000000000000284, 2.628524454178448710 ) ) ;
#4904=CARTESIAN_POINT ( 'NONE',  ( -34.50000000000000000, -111.0140978167138570, 0.0002176474015659786963 ) ) ;
#4907=CARTESIAN_POINT ( 'NONE',  ( -35.50000000000000711, -114.2305202833893816, 9.534416457224700991 ) ) ;
#4909=CARTESIAN_POINT ( 'NONE',  ( -34.50000000000000000, -113.9929510916434339, 10.52000928670414126 ) ) ;
#4913=CARTESIAN_POINT ( 'NONE',  ( -34.50000000000000000, -113.9917898843777522, 10.50611893782865813 ) ) ;
#4916=CARTESIAN_POINT ( 'NONE',  ( -37.42187499999996447, -115.9929510916434481, 13.11852480586264846 ) ) ;
#4928=CARTESIAN_POINT ( 'NONE',  ( -35.50000000000000711, -112.0140978167138712, 0.8127176474015721519 ) ) ;
#4932=CARTESIAN_POINT ( 'NONE',  ( -35.50160444427493189, -114.9929510916434339, 12.65937477241749853 ) ) ;
#4937=CARTESIAN_POINT ( 'NONE',  ( -35.50000000000000000, -113.8474311500459777, -2.624782352598442614 ) ) ;
#4940=CARTESIAN_POINT ( 'NONE',  ( -35.99999999999999289, -114.0592624029313242, 7.503524454178450043 ) ) ;
#4945=CARTESIAN_POINT ( 'NONE',  ( -34.50000000000000000, -114.6807644833805000, -0.6247823525984269599 ) ) ;
#4948=CARTESIAN_POINT ( 'NONE',  ( -38.00000000000000711, -114.9929510916434339, 12.39849696637031151 ) ) ;
#4951=CARTESIAN_POINT ( 'NONE',  ( -34.50000000000000000, -112.0140978167138712, -0.5622823525984296245 ) ) ;
#4958=CARTESIAN_POINT ( 'NONE',  ( -37.48437500000004263, -115.9929510916434481, 13.11852480586264846 ) ) ;
#4979=CARTESIAN_POINT ( 'NONE',  ( -37.76916472181486739, -116.0245472910329880, 4.465225545821550845 ) ) ;
#4999=CARTESIAN_POINT ( 'NONE',  ( -38.97545270896704039, -113.1123104723225055, 6.847274454178450043 ) ) ;
#5000=CARTESIAN_POINT ( 'NONE',  ( -34.50000000000000000, -115.9929510916434481, 12.56351784598954424 ) ) ;
#5012=CARTESIAN_POINT ( 'NONE',  ( -36.94073759706868287, -116.9999999999999858, 8.871475545821548181 ) ) ;
#5033=CARTESIAN_POINT ( 'NONE',  ( -35.50000000000000711, -112.0154707866092707, 0.9357013553229778235 ) ) ;
#5041=CARTESIAN_POINT ( 'NONE',  ( -34.50000000000000000, -115.8878449012421754, -1.128496220799388494 ) ) ;
#5043=APPLICATION_CONTEXT ( 'automotive_design' ) ;
#5045=CARTESIAN_POINT ( 'NONE',  ( -34.50000000000000000, -114.3464919575557843, 9.568884482464163455 ) ) ;
#5049=CARTESIAN_POINT ( 'NONE',  ( -35.50000000000000000, -113.9883062625807071, 10.50570311110699961 ) ) ;
#5051=CARTESIAN_POINT ( 'NONE',  ( -34.50000000000000000, -114.9492820284331742, 10.20776876943783940 ) ) ;
#5053=CARTESIAN_POINT ( 'NONE',  ( -37.99839555572501837, -114.9929510916434339, 12.65937477241748965 ) ) ;
#5059=CARTESIAN_POINT ( 'NONE',  ( -38.00000000000000711, -114.9929510916434339, 12.50851088611646311 ) ) ;
#5062=CARTESIAN_POINT ( 'NONE',  ( -35.02454729103298803, -114.8876895276775087, 6.097274454178449155 ) ) ;
#5071=CARTESIAN_POINT ( 'NONE',  ( -40.02454729103296671, -115.1833782841879525, 5.159774454178449155 ) ) ;
#5084=CARTESIAN_POINT ( 'NONE',  ( -34.50000000000000000, -111.0278007905855588, 1.116632271043183078 ) ) ;
#5089=CARTESIAN_POINT ( 'NONE',  ( -34.50000000000000000, -113.9929510916434339, 10.50625754673588474 ) ) ;
#5095=CARTESIAN_POINT ( 'NONE',  ( -34.50000000000000000, -113.9929510916434623, 10.50625754673586876 ) ) ;
#5097=CARTESIAN_POINT ( 'NONE',  ( -37.18750000000004974, -115.9929510916434481, 13.11852480586264846 ) ) ;
#5111=CARTESIAN_POINT ( 'NONE',  ( -35.50000000000000000, -113.0140978167138712, 0.3752176474015639918 ) ) ;
#5113=CARTESIAN_POINT ( 'NONE',  ( -35.50000000000000711, -114.9929501463477663, 10.50247632894551231 ) ) ;
#5117=CARTESIAN_POINT ( 'NONE',  ( -35.50000000000000000, -111.0140821919084715, 0.8283428459075261596 ) ) ;
#5120=CARTESIAN_POINT ( 'NONE',  ( -37.47347596530441649, -114.9754527089670262, 6.472274454178449155 ) ) ;
#5127=CARTESIAN_POINT ( 'NONE',  ( -34.50000000000000000, -113.0140978167138712, 0.7502176474015694874 ) ) ;
#5133=CARTESIAN_POINT ( 'NONE',  ( -37.97447287825094975, -114.9929510916434339, 12.77960891308616809 ) ) ;
#5138=CARTESIAN_POINT ( 'NONE',  ( -34.50000000000000000, -115.0468226098135744, -1.624774171496087716 ) ) ;
#5143=CARTESIAN_POINT ( 'NONE',  ( -38.00000000000000711, -115.9929510916434481, 12.26648026267477221 ) ) ;
#5163=CARTESIAN_POINT ( 'NONE',  ( -35.62769128460905677, -112.5438815906447729, 3.808975545821551290 ) ) ;
#5186=CARTESIAN_POINT ( 'NONE',  ( -38.97545270896704039, -113.1123104723225055, 5.347274454178449155 ) ) ;
#5187=CARTESIAN_POINT ( 'NONE',  ( -37.59808119975203766, -115.9929510916434481, 14.11551573851449071 ) ) ;
#5196=CARTESIAN_POINT ( 'NONE',  ( -34.02454729103297382, -112.6980969099494132, 9.902725545821553510 ) ) ;
#5202=CARTESIAN_POINT ( 'NONE',  ( -34.50000000000000000, -113.9344536409997630, 0.9850770315317123327 ) ) ;
#5218=CARTESIAN_POINT ( 'NONE',  ( -35.50000000000000711, -114.0000000000000853, 2.000000000000001776 ) ) ;
#5224=CARTESIAN_POINT ( 'NONE',  ( -34.50000000000000000, -116.0140978167138712, -0.4997823525984418369 ) ) ;
#5225=CARTESIAN_POINT ( 'NONE',  ( -35.95093014754292682, -114.9929510916434339, 14.11777216781842448 ) ) ;
#5227=CARTESIAN_POINT ( 'NONE',  ( -35.50000000000000000, -113.9929510916434339, 10.50625754673588474 ) ) ;
#5229=CARTESIAN_POINT ( 'NONE',  ( -39.00000000000000000, -113.9929510916434339, 12.59102132592609102 ) ) ;
#5237=CARTESIAN_POINT ( 'NONE',  ( -37.66108410722335265, -114.9929510916434339, 13.09299768411426790 ) ) ;
#5239=CARTESIAN_POINT ( 'NONE',  ( -35.62769128460905677, -115.4561184093552413, 7.691024454178449155 ) ) ;
#5247=CARTESIAN_POINT ( 'NONE',  ( -34.00000000000000000, -113.9407375970686758, 2.496475545821551290 ) ) ;
#5250=CARTESIAN_POINT ( 'NONE',  ( -35.50000000000000711, -116.0140978167138712, 0.8752176474015622709 ) ) ;
#5261=CARTESIAN_POINT ( 'NONE',  ( -34.50000000000000000, -111.4147656069378058, -1.853877267569947529 ) ) ;
#5265=CARTESIAN_POINT ( 'NONE',  ( -35.50000000000000711, -114.9929510916434339, 10.59426868253284226 ) ) ;
#5266=CARTESIAN_POINT ( 'NONE',  ( -36.00976557831293690, -113.9929510916434339, 14.11852773550420359 ) ) ;
#5269=CARTESIAN_POINT ( 'NONE',  ( -38.00000000000000711, -113.9929510916434339, 12.57451923796417681 ) ) ;
#5270=CARTESIAN_POINT ( 'NONE',  ( -37.66108410722335265, -115.9929510916434481, 13.09299768411426612 ) ) ;
#5283=CARTESIAN_POINT ( 'NONE',  ( -35.50000000000000711, -116.0140978167138712, -0.1247823525984439463 ) ) ;
#5285=CARTESIAN_POINT ( 'NONE',  ( -35.50000000000000711, -114.9929296450195721, 10.49869535309826674 ) ) ;
#5290=CARTESIAN_POINT ( 'NONE',  ( -35.50000000000000000, -112.0066700803175763, -2.372276521656937920 ) ) ;
#5294=CARTESIAN_POINT ( 'NONE',  ( -35.97545270896702618, -113.6450488405582604, 8.909774454178450043 ) ) ;
#5299=CARTESIAN_POINT ( 'NONE',  ( -34.50000000000000000, -113.0140978167143260, -0.6247823525984285142 ) ) ;
#5307=CARTESIAN_POINT ( 'NONE',  ( -35.50000000000000000, -113.9929510916434339, 10.55026311463432087 ) ) ;
#5310=CARTESIAN_POINT ( 'NONE',  ( -34.50000000000000000, -112.0140978167138712, 0.2502176474015765373 ) ) ;
#5311=CARTESIAN_POINT ( 'NONE',  ( -34.50120407906360498, -115.9929510916434481, 12.67985367974112343 ) ) ;
#5316=CARTESIAN_POINT ( 'NONE',  ( -35.50000000000000711, -114.0743172650041686, 9.508870970061893857 ) ) ;
#5337=CARTESIAN_POINT ( 'NONE',  ( -36.94073759706868287, -115.9999999999999858, 5.871475545821550845 ) ) ;
#5356=CARTESIAN_POINT ( 'NONE',  ( -36.15625000000007816, -115.9929510916434481, 14.11852480586265024 ) ) ;
#5367=CARTESIAN_POINT ( 'NONE',  ( -36.02454729103297382, -113.5265240346956261, 3.902725545821552178 ) ) ;
#5392=CARTESIAN_POINT ( 'NONE',  ( -34.50000000000000000, -114.5974311500472425, -1.624782352598427959 ) ) ;
#5394=CARTESIAN_POINT ( 'NONE',  ( -36.03125000000004263, -114.9929510916434339, 14.11852480586264846 ) ) ;
#5397=CARTESIAN_POINT ( 'NONE',  ( -35.50000000000000000, -113.9465028010160381, 10.50071319044726081 ) ) ;
#5399=CARTESIAN_POINT ( 'NONE',  ( -34.50000000000000000, -114.9929510916434339, 12.44250253426871033 ) ) ;
#5411=CARTESIAN_POINT ( 'NONE',  ( -34.97545270896703329, -113.2308352781851539, 8.909774454178450043 ) ) ;
#5419=CARTESIAN_POINT ( 'NONE',  ( -39.97545270896702618, -115.3019030900506152, 3.152725545821551734 ) ) ;
#5430=CARTESIAN_POINT ( 'NONE',  ( -34.50000000000000000, -111.1162063037085801, -1.269118781493287607 ) ) ;
#5433=CARTESIAN_POINT ( 'NONE',  ( -35.50000000000000711, -114.9929510916434339, 10.56126450660895699 ) ) ;
#5434=CARTESIAN_POINT ( 'NONE',  ( -34.68937937320795584, -113.9929510916434339, 13.37409560816408671 ) ) ;
#5437=CARTESIAN_POINT ( 'NONE',  ( -34.57658136524561598, -113.9929510916434339, 13.10177712753338675 ) ) ;
#5439=CARTESIAN_POINT ( 'NONE',  ( -35.50000000000000711, -114.2305202833893816, 9.534416457224700991 ) ) ;
#5452=CARTESIAN_POINT ( 'NONE',  ( -35.50000000000000000, -113.0140978167142833, 0.8752176474015604946 ) ) ;
#5454=CARTESIAN_POINT ( 'NONE',  ( -36.02454729103298092, -114.4734759653044307, 4.597274454178449155 ) ) ;
#5456=CARTESIAN_POINT ( 'NONE',  ( -35.50000000000000711, -114.9929510916434339, 12.60752341388803544 ) ) ;
#5460=CARTESIAN_POINT ( 'NONE',  ( -35.50000000000000000, -112.6882700046066645, -2.599147725882136939 ) ) ;
#5463=CARTESIAN_POINT ( 'NONE',  ( -35.62769128460905677, -115.4561184093552413, 7.691024454178449155 ) ) ;
#5467=CARTESIAN_POINT ( 'NONE',  ( -34.50000000000000000, -114.5974311500472567, -0.6247823525984269599 ) ) ;
#5469=AXIS2_PLACEMENT_3D ( 'NONE', #4451, #1376, #17383 ) ;
#5475=CARTESIAN_POINT ( 'NONE',  ( -35.50000000000000000, -113.9929510916433912, 10.50625754673588474 ) ) ;
#5478=CARTESIAN_POINT ( 'NONE',  ( -34.50000000000000000, -111.0140978167138570, -0.3122823525984338988 ) ) ;
#5479=CARTESIAN_POINT ( 'NONE',  ( -35.50000000000000000, -114.2265172349312508, 8.519938377296172760 ) ) ;
#5485=CARTESIAN_POINT ( 'NONE',  ( -37.66108410722335265, -115.9929510916434481, 13.09299768411426612 ) ) ;
#5507=CARTESIAN_POINT ( 'NONE',  ( -36.94073759706868287, -115.9999999999999858, 7.371475545821551734 ) ) ;
#5517=CARTESIAN_POINT ( 'NONE',  ( -35.50000000000000711, -114.9929510916434339, 10.52826033068511435 ) ) ;
#5527=CARTESIAN_POINT ( 'NONE',  ( -38.98077402996267438, -115.9929510916434481, 12.86289566494346204 ) ) ;
#5537=CARTESIAN_POINT ( 'NONE',  ( -39.02454729103295961, -113.2308352781851539, 9.340225545821549957 ) ) ;
#5566=CARTESIAN_POINT ( 'NONE',  ( -34.50000000000000000, -112.0140978167138712, -0.5622823525984296245 ) ) ;
#5567=CARTESIAN_POINT ( 'NONE',  ( -38.99984940073101569, -114.9929510916434339, 12.64306614848957189 ) ) ;
#5570=CARTESIAN_POINT ( 'NONE',  ( -35.50000000000000000, -113.9929510916436470, 10.50625754673581724 ) ) ;
#5573=CARTESIAN_POINT ( 'NONE',  ( -34.51202277066418844, -114.9929510916434339, 12.81430620224972294 ) ) ;
#5584=CARTESIAN_POINT ( 'NONE',  ( -37.05926240293133134, -116.9999999999999858, 7.878524454178450043 ) ) ;
#5594=CARTESIAN_POINT ( 'NONE',  ( -34.83677480945819838, -111.9205845034225462, 7.316024454178450043 ) ) ;
#5607=CARTESIAN_POINT ( 'NONE',  ( -35.50000000000000000, -111.2304026862503719, 1.811733666967775713 ) ) ;
#5613=CARTESIAN_POINT ( 'NONE',  ( -36.12500000000014211, -114.9929510916434339, 13.11852480586264669 ) ) ;
#5614=CARTESIAN_POINT ( 'NONE',  ( -35.87745010033553683, -113.9929510916434339, 14.11371147303761475 ) ) ;
#5619=CARTESIAN_POINT ( 'NONE',  ( -34.50000000000000000, -113.9929510916435618, 10.50625754673588474 ) ) ;
#5621=CARTESIAN_POINT ( 'NONE',  ( -35.50000000000000711, -114.9929510916434339, 10.72628538622835670 ) ) ;
#5634=CARTESIAN_POINT ( 'NONE',  ( -35.50000000000000000, -113.0140978167138712, 0.8752176474016720720 ) ) ;
#5636=CARTESIAN_POINT ( 'NONE',  ( -37.66520193420439000, -113.2509883718312977, 5.441024454178449155 ) ) ;
#5641=CARTESIAN_POINT ( 'NONE',  ( -35.50000000000000000, -117.0140978167138854, -0.3122823525984416149 ) ) ;
#5644=CARTESIAN_POINT ( 'NONE',  ( -35.54388159064475872, -112.6276912846090568, 7.316024454178449155 ) ) ;
#5650=CARTESIAN_POINT ( 'NONE',  ( -34.50000000000000000, -112.8356783780338759, 1.859636627348750348 ) ) ;
#5657=CARTESIAN_POINT ( 'NONE',  ( -35.49999931242378182, -113.9929510916434339, 12.61439929482945743 ) ) ;
#5660=CARTESIAN_POINT ( 'NONE',  ( -34.50000000000000000, -111.0140978167138570, 0.7189676474015717078 ) ) ;
#5661=CARTESIAN_POINT ( 'NONE',  ( -37.54906985245723661, -115.9929510916434481, 14.11777216781844757 ) ) ;
#5666=CARTESIAN_POINT ( 'NONE',  ( -35.50000000000000711, -114.0928965812550757, 9.511088712577292270 ) ) ;
#5686=CARTESIAN_POINT ( 'NONE',  ( -37.35495115944176803, -115.0245472910329880, 4.465225545821550845 ) ) ;
#5693=CARTESIAN_POINT ( 'NONE',  ( -35.50000000000000711, -114.1021862393805577, 9.512197583835053649 ) ) ;
#5701=CARTESIAN_POINT ( 'NONE',  ( -39.00000000000000000, -115.9929510916434481, 12.59102132592609102 ) ) ;
#5709=CARTESIAN_POINT ( 'NONE',  ( -38.45611840935523418, -112.6276912846090568, 7.933975545821552622 ) ) ;
#5739=CARTESIAN_POINT ( 'NONE',  ( -34.50000000000000000, -112.0140978167138712, 0.2502176474015765373 ) ) ;
#5740=CARTESIAN_POINT ( 'NONE',  ( -37.74437085908087397, -114.9929510916434339, 14.09929883582536903 ) ) ;
#5741=CARTESIAN_POINT ( 'NONE',  ( -38.00000000000000711, -114.9929510916434339, 12.50851088611646311 ) ) ;
#5743=CARTESIAN_POINT ( 'NONE',  ( -36.12500000000014211, -114.9929510916434339, 14.11852480586264846 ) ) ;
#5755=CARTESIAN_POINT ( 'NONE',  ( -35.69809690994938478, -111.0245472910330022, 4.222274454178449155 ) ) ;
#5759=CARTESIAN_POINT ( 'NONE',  ( -35.50000000000000711, -112.9813730236132585, -1.624774171495860786 ) ) ;
#5779=CARTESIAN_POINT ( 'NONE',  ( -34.50000000000000000, -115.0631849411758196, -2.624765990393648885 ) ) ;
#5783=CARTESIAN_POINT ( 'NONE',  ( -36.03906250000000000, -114.9929510916434339, 13.11852480586264669 ) ) ;
#5785=CARTESIAN_POINT ( 'NONE',  ( -37.18750000000004974, -113.9929510916434339, 14.11852480586265024 ) ) ;
#5788=CARTESIAN_POINT ( 'NONE',  ( -34.50000000000000000, -113.9929510916434339, 12.17846912687782712 ) ) ;
#5789=CARTESIAN_POINT ( 'NONE',  ( -38.99518666717493431, -114.9929510916434339, 12.74107470552714716 ) ) ;
#5791=CARTESIAN_POINT ( 'NONE',  ( -35.50000000000000711, -114.9656200615856818, 10.26631071845107179 ) ) ;
#5803=CARTESIAN_POINT ( 'NONE',  ( -35.50000000000000711, -115.2732872103912030, -1.592823285204062911 ) ) ;
#5806=CARTESIAN_POINT ( 'NONE',  ( -37.05926240293131713, -115.9999999999999858, 6.378524454178448266 ) ) ;
#5812=CARTESIAN_POINT ( 'NONE',  ( -35.50000000000000711, -113.8159288351371714, 1.978028123174813802 ) ) ;
#5816=CARTESIAN_POINT ( 'NONE',  ( -36.23083527818512550, -116.0245472910329880, 6.284774454178450043 ) ) ;
#5821=CARTESIAN_POINT ( 'NONE',  ( -34.50000000000000000, -112.0250551866464548, 1.025914454044489332 ) ) ;
#5824=CARTESIAN_POINT ( 'NONE',  ( -35.50000000000000000, -113.9929510916434339, 10.50625754673587409 ) ) ;
#5830=CARTESIAN_POINT ( 'NONE',  ( -34.50000000000000000, -112.8115600290184801, 2.865251044451027074 ) ) ;
#5831=CARTESIAN_POINT ( 'NONE',  ( -35.50000000000000000, -114.1928420708668028, 8.515919878418792166 ) ) ;
#5853=CARTESIAN_POINT ( 'NONE',  ( -36.02454729103297382, -113.5265240346956261, 3.902725545821552178 ) ) ;
#5861=CARTESIAN_POINT ( 'NONE',  ( -35.50000000000000711, -116.0140978167138712, -0.5622823525984409487 ) ) ;
#5864=CARTESIAN_POINT ( 'NONE',  ( -35.50000000000000711, -114.9902084924877954, 10.43071793783961176 ) ) ;
#5867=CARTESIAN_POINT ( 'NONE',  ( -34.50000000000000000, -114.5636144531578680, 9.676196722963288366 ) ) ;
#5870=CARTESIAN_POINT ( 'NONE',  ( -37.49023442168701337, -115.9929510916434481, 14.11852773550420359 ) ) ;
#5880=CARTESIAN_POINT ( 'NONE',  ( -36.11231047232249125, -115.9754527089670262, 8.777725545821555286 ) ) ;
#5906=CARTESIAN_POINT ( 'NONE',  ( -34.50000000000000000, -116.0140978167138712, 0.0002176474015577116276 ) ) ;
#5909=CARTESIAN_POINT ( 'NONE',  ( -34.50000000000000000, -115.9929524668003182, 10.51038305125561401 ) ) ;
#5910=CARTESIAN_POINT ( 'NONE',  ( -38.50000000000000711, -114.9929510916434339, 10.50625754673587231 ) ) ;
#5912=CARTESIAN_POINT ( 'NONE',  ( -34.49999793727135255, -114.9929510916434339, 12.61164896875036590 ) ) ;
#5925=CARTESIAN_POINT ( 'NONE',  ( -35.81662171581204746, -117.0245472910329738, 3.284774454178449155 ) ) ;
#5927=CARTESIAN_POINT ( 'NONE',  ( -35.50000000000000711, -112.0140978167138712, -0.3747823525984256832 ) ) ;
#5946=CARTESIAN_POINT ( 'NONE',  ( -35.50000000000000000, -111.3577635893106361, 2.022004269840791402 ) ) ;
#5951=CARTESIAN_POINT ( 'NONE',  ( -35.50400759022159036, -114.9929510916434339, 12.68378527132497524 ) ) ;
#5953=CARTESIAN_POINT ( 'NONE',  ( -34.50000000000000000, -113.9929510916434339, 12.50851088611648265 ) ) ;
#5956=CARTESIAN_POINT ( 'NONE',  ( -34.50000000000000000, -113.9929510916436470, 10.50625754673581724 ) ) ;
#5958=CARTESIAN_POINT ( 'NONE',  ( -35.50000000000000711, -114.0743172650041686, 9.508870970061893857 ) ) ;
#5974=CARTESIAN_POINT ( 'NONE',  ( -35.50000000000000000, -114.9932644833805426, -0.6247823525982824089 ) ) ;
#5976=CARTESIAN_POINT ( 'NONE',  ( -34.97545270896703329, -113.2308352781851539, 2.909774454178448710 ) ) ;
#5983=CARTESIAN_POINT ( 'NONE',  ( -35.50000000000000000, -114.8057644833805853, -2.624782352598442614 ) ) ;
#5991=CARTESIAN_POINT ( 'NONE',  ( -34.50000000000000000, -112.0141053790792114, 0.9054673897245171243 ) ) ;
#5997=CARTESIAN_POINT ( 'NONE',  ( -35.50640865667917723, -113.9929510916434339, 12.69998175888958691 ) ) ;
#6003=CARTESIAN_POINT ( 'NONE',  ( -34.50000000000000000, -113.8814751941374652, 2.992951091643117678 ) ) ;
#6004=CARTESIAN_POINT ( 'NONE',  ( -35.50000000000000000, -114.2675000158779710, 8.525177020294046670 ) ) ;
#6028=CARTESIAN_POINT ( 'NONE',  ( -35.97545270896705460, -114.3549511594417680, 4.090225545821551734 ) ) ;
#6034=CARTESIAN_POINT ( 'NONE',  ( -35.50000000000000711, -116.0140978167138712, 0.8752176474015622709 ) ) ;
#6039=CARTESIAN_POINT ( 'NONE',  ( -35.50000000000000711, -114.9860996047076895, 10.38555023491505835 ) ) ;
#6042=CARTESIAN_POINT ( 'NONE',  ( -34.50000000000000000, -114.9929510916434339, 10.53376102667243508 ) ) ;
#6047=CARTESIAN_POINT ( 'NONE',  ( -35.50000000000000000, -115.9929510916434481, 10.51175824272318415 ) ) ;
#6048=CARTESIAN_POINT ( 'NONE',  ( -35.50000000000000711, -112.0140978167138712, 0.2502176474015765373 ) ) ;
#6051=PLANE ( 'NONE',  #33149 ) ;
#6058=CARTESIAN_POINT ( 'NONE',  ( -38.02454729103295961, -113.6450488405582462, 3.340225545821551290 ) ) ;
#6084=CARTESIAN_POINT ( 'NONE',  ( -34.50000000000000000, -115.0140978167138712, 0.6252176474015650465 ) ) ;
#6087=CARTESIAN_POINT ( 'NONE',  ( -34.50000000000000000, -114.1371041221139109, 8.509266650872710613 ) ) ;
#6090=CARTESIAN_POINT ( 'NONE',  ( -39.00000206272865455, -114.9929510916434339, 12.61164896875035701 ) ) ;
#6099=CARTESIAN_POINT ( 'NONE',  ( -34.83677480945819838, -111.9205845034225462, 4.316024454178448266 ) ) ;
#6102=CARTESIAN_POINT ( 'NONE',  ( -35.50000000000000711, -112.0140978167138712, 0.2502176474015765373 ) ) ;
#6119=CARTESIAN_POINT ( 'NONE',  ( -35.50000000000000000, -111.0141129414446652, 0.9205922128478062350 ) ) ;
#6126=CARTESIAN_POINT ( 'NONE',  ( -35.97955704204053262, -114.9929510916434339, 13.11812344617474579 ) ) ;
#6127=MECHANICAL_DESIGN_GEOMETRIC_PRESENTATION_REPRESENTATION('',(#20502),#12480);
#6130=CARTESIAN_POINT ( 'NONE',  ( -38.99924736195577424, -113.9929510916434339, 12.66759465831984599 ) ) ;
#6135=CARTESIAN_POINT ( 'NONE',  ( -34.50000000000000000, -113.9929510916434339, 10.50625754673609258 ) ) ;
#6136=CARTESIAN_POINT ( 'NONE',  ( -39.00000000000000711, -114.9929510916434339, 11.73841344789285657 ) ) ;
#6138=CARTESIAN_POINT ( 'NONE',  ( -35.50000000000000711, -114.9819937217110635, 10.35556074009299188 ) ) ;
#6149=CARTESIAN_POINT ( 'NONE',  ( -35.50000000000000000, -115.0140978167139707, -0.6091573525984161908 ) ) ;
#6151=CARTESIAN_POINT ( 'NONE',  ( -38.97545270896704039, -113.1123104723225197, 5.347274454178449155 ) ) ;
#6157=CARTESIAN_POINT ( 'NONE',  ( -35.50000000000000000, -116.7615919857705080, -1.632210089000343700 ) ) ;
#6161=CARTESIAN_POINT ( 'NONE',  ( -35.02454729103298803, -114.8876895276775087, 7.597274454178450931 ) ) ;
#6166=CARTESIAN_POINT ( 'NONE',  ( -34.50000000000000000, -112.0140978167138712, -0.3747823525984256832 ) ) ;
#6176=CARTESIAN_POINT ( 'NONE',  ( -37.99959864031216483, -113.9929510916434339, 12.63896776382213538 ) ) ;
#6180=CARTESIAN_POINT ( 'NONE',  ( -34.50000000000000000, -111.0168437565048691, 0.9961850632443862708 ) ) ;
#6184=CARTESIAN_POINT ( 'NONE',  ( -38.81062062679291813, -115.9929510916434481, 13.37409560816442244 ) ) ;
#6205=CARTESIAN_POINT ( 'NONE',  ( -37.74901162816868805, -113.3347980657955958, 6.433975545821551734 ) ) ;
#6216=CARTESIAN_POINT ( 'NONE',  ( -35.50000000000000711, -115.9630435732166518, -0.9469505670456015434 ) ) ;
#6218=CARTESIAN_POINT ( 'NONE',  ( -35.50000000000000711, -114.1712995509219724, 9.522174004479579068 ) ) ;
#6222=CARTESIAN_POINT ( 'NONE',  ( -34.50000000000000000, -114.0882517521923489, 9.510534276948430232 ) ) ;
#6225=CARTESIAN_POINT ( 'NONE',  ( -35.50000000000000000, -114.2207110452431635, 8.519246492191951958 ) ) ;
#6226=CARTESIAN_POINT ( 'NONE',  ( -35.50000000000000711, -113.2637153405686519, 1.912112492696748989 ) ) ;
#6236=CARTESIAN_POINT ( 'NONE',  ( -37.05926240293131713, -113.0000000000000000, 5.121475545821551734 ) ) ;
#6247=CARTESIAN_POINT ( 'NONE',  ( -39.97545270896702618, -112.6980969099493990, 8.347274454178448266 ) ) ;
#6261=CARTESIAN_POINT ( 'NONE',  ( -34.50000000000000000, -113.6318576702834804, 1.956056246348823580 ) ) ;
#6264=CARTESIAN_POINT ( 'NONE',  ( -39.00000000000000711, -114.9929510916434339, 12.44250253426874941 ) ) ;
#6267=CARTESIAN_POINT ( 'NONE',  ( -34.50000000000000000, -114.1928420708668028, 8.515919878418792166 ) ) ;
#6276=CARTESIAN_POINT ( 'NONE',  ( -39.99999999999999289, -113.9407375970686758, 8.253524454178448266 ) ) ;
#6278=CARTESIAN_POINT ( 'NONE',  ( -35.50000000000000711, -115.1770117227680998, -1.611965039240062181 ) ) ;
#6292=CARTESIAN_POINT ( 'NONE',  ( -38.97545270896704039, -114.8876895276775087, 3.152725545821551290 ) ) ;
#6297=CARTESIAN_POINT ( 'NONE',  ( -35.50000000000000000, -111.0140978167138570, 0.3752176474015639918 ) ) ;
#6300=CARTESIAN_POINT ( 'NONE',  ( -35.50000000000000711, -114.9929510916434339, 11.73841344789270202 ) ) ;
#6302=CARTESIAN_POINT ( 'NONE',  ( -37.51022648969539119, -113.9929510916434339, 14.11852173794918563 ) ) ;
#6307=CARTESIAN_POINT ( 'NONE',  ( -35.75562914091914024, -113.9929510916434339, 14.09929883582542409 ) ) ;
#6310=CARTESIAN_POINT ( 'NONE',  ( -35.50000000000000711, -114.9929510916434339, 12.50851088611648088 ) ) ;
#6314=CARTESIAN_POINT ( 'NONE',  ( -35.50000000000000711, -114.0000000000003411, 9.500000000000035527 ) ) ;
#6322=CARTESIAN_POINT ( 'NONE',  ( -35.50000000000000000, -113.0140978167137860, -0.6247823525984055326 ) ) ;
#6324=CARTESIAN_POINT ( 'NONE',  ( -37.66520193420439000, -113.2509883718312977, 8.441024454178448266 ) ) ;
#6327=CARTESIAN_POINT ( 'NONE',  ( -35.62769128460905677, -115.4561184093552413, 4.691024454178448266 ) ) ;
#6330=CARTESIAN_POINT ( 'NONE',  ( -35.50000000000000000, -117.0140978167138854, 0.6252176474015650465 ) ) ;
#6340=CARTESIAN_POINT ( 'NONE',  ( -34.50000000000000000, -115.0140978167138712, 0.6252176474015650465 ) ) ;
#6346=CARTESIAN_POINT ( 'NONE',  ( -35.91854304697312728, -113.9929510916434339, 13.11211614918345703 ) ) ;
#6350=CARTESIAN_POINT ( 'NONE',  ( -35.52552712174883709, -113.9929510916434339, 12.77960891308624625 ) ) ;
#6351=CARTESIAN_POINT ( 'NONE',  ( -35.50000000000000000, -115.9929510916434481, 10.68227981832981044 ) ) ;
#6364=CARTESIAN_POINT ( 'NONE',  ( -35.50000000000000711, -114.0000000000000853, 2.000000000000001776 ) ) ;
#6377=CARTESIAN_POINT ( 'NONE',  ( -37.66520193420439711, -114.7490116281687023, 6.058975545821550845 ) ) ;
#6388=CARTESIAN_POINT ( 'NONE',  ( -35.50000000000000711, -114.9929510916434339, 12.56351784598954424 ) ) ;
#6392=CARTESIAN_POINT ( 'NONE',  ( -34.50000000000000000, -114.1068310684433129, 9.512752019463897923 ) ) ;
#6396=CARTESIAN_POINT ( 'NONE',  ( -35.50000000000000000, -115.9792481177720731, 10.26484292309424795 ) ) ;
#6408=CARTESIAN_POINT ( 'NONE',  ( -37.99999999999998579, -114.0592624029313242, 9.246475545821549957 ) ) ;
#6417=CARTESIAN_POINT ( 'NONE',  ( -39.07941549657748936, -111.8367748094582055, 8.441024454178448266 ) ) ;
#6433=CARTESIAN_POINT ( 'NONE',  ( -34.50000000000000000, -115.0140978167138712, -0.6247823525984408377 ) ) ;
#6436=CARTESIAN_POINT ( 'NONE',  ( -34.50000000000000000, -115.9929510916434481, 10.56126450660895699 ) ) ;
#6440=CARTESIAN_POINT ( 'NONE',  ( -38.92341863475394348, -114.9929510916434339, 13.10177712753322155 ) ) ;
#6442=CARTESIAN_POINT ( 'NONE',  ( -35.00000000000000000, -116.0140978167138712, 0.8752176474015622709 ) ) ;
#6450=CARTESIAN_POINT ( 'NONE',  ( -37.05926240293131713, -111.0000000000000284, 3.621475545821551734 ) ) ;
#6453=CARTESIAN_POINT ( 'NONE',  ( -35.50000000000000711, -114.3474311500471430, -1.624782352598427959 ) ) ;
#6466=CARTESIAN_POINT ( 'NONE',  ( -35.02454729103298092, -113.1123104723225055, 3.902725545821551290 ) ) ;
#6471=CARTESIAN_POINT ( 'NONE',  ( -35.50000000000000000, -111.0140978167138570, -0.3122823525984338988 ) ) ;
#6478=CARTESIAN_POINT ( 'NONE',  ( -39.00000000000000000, -113.9929510916434339, 12.50851088611646311 ) ) ;
#6482=CARTESIAN_POINT ( 'NONE',  ( -37.46093750000000711, -113.9929510916434339, 14.11852480586265024 ) ) ;
#6484=CARTESIAN_POINT ( 'NONE',  ( -35.74814306589956914, -114.9929510916434339, 13.05539834812772781 ) ) ;
#6489=CARTESIAN_POINT ( 'NONE',  ( -35.50000000000000711, -114.9929510916434339, 10.85830208992344303 ) ) ;
#6497=CARTESIAN_POINT ( 'NONE',  ( -35.50000000000000000, -114.8474311500471572, -0.6247823525984269599 ) ) ;
#6499=CARTESIAN_POINT ( 'NONE',  ( -38.99999999999999289, -113.9407375970686900, 3.753524454178449155 ) ) ;
#6501=CARTESIAN_POINT ( 'NONE',  ( -36.94073759706868287, -112.0000000000000142, 2.628524454178448710 ) ) ;
#6503=CARTESIAN_POINT ( 'NONE',  ( -35.50000000000000711, -116.0141056290913610, -0.5935324770972248976 ) ) ;
#6512=CARTESIAN_POINT ( 'NONE',  ( -34.50000000000000000, -116.0141056290913610, -0.5935324770972248976 ) ) ;
#6513=CARTESIAN_POINT ( 'NONE',  ( -35.50000000000000711, -112.0414288467712112, 1.115164475686276191 ) ) ;
#6521=CARTESIAN_POINT ( 'NONE',  ( -37.89983305244309264, -113.9929510916434339, 12.92579853460519423 ) ) ;
#6523=CARTESIAN_POINT ( 'NONE',  ( -35.50000000000000000, -113.9929510916434339, 10.72628538622835670 ) ) ;
#6524=CARTESIAN_POINT ( 'NONE',  ( -35.50025087934803736, -115.9929510916434481, 12.63488142334835196 ) ) ;
#6543=CARTESIAN_POINT ( 'NONE',  ( -34.50000000000000000, -111.2666036476567655, -1.632210088999287212 ) ) ;
#6547=CARTESIAN_POINT ( 'NONE',  ( -35.99999999999999289, -113.9407375970686758, 8.496475545821549957 ) ) ;
#6551=CARTESIAN_POINT ( 'NONE',  ( -34.50000000000000000, -113.0140978167136581, 0.8752176474015604946 ) ) ;
#6556=CARTESIAN_POINT ( 'NONE',  ( -36.03906250000000000, -114.9929510916434339, 13.11852480586264669 ) ) ;
#6560=CARTESIAN_POINT ( 'NONE',  ( -34.50000000000000000, -114.9929510916434339, 11.38636890470581164 ) ) ;
#6565=CARTESIAN_POINT ( 'NONE',  ( -39.00000000000000000, -115.9929510916434481, 12.39849696637031151 ) ) ;
#6566=CARTESIAN_POINT ( 'NONE',  ( -35.50000000000000711, -112.7472371723319355, 1.839427296857320648 ) ) ;
#6578=CARTESIAN_POINT ( 'NONE',  ( -36.94073759706868287, -115.0000000000000000, 8.871475545821548181 ) ) ;
#6587=CARTESIAN_POINT ( 'NONE',  ( -37.05926240293131713, -112.0000000000000142, 3.621475545821551290 ) ) ;
#6607=CARTESIAN_POINT ( 'NONE',  ( -34.50000000000000000, -113.6807644833805995, -0.6247823525984269599 ) ) ;
#6611=CARTESIAN_POINT ( 'NONE',  ( -34.50000000000000000, -114.2183886307118428, 8.518969274377507617 ) ) ;
#6615=CARTESIAN_POINT ( 'NONE',  ( -39.00000000000000711, -114.9929510916434339, 12.60752341388803721 ) ) ;
#6624=CARTESIAN_POINT ( 'NONE',  ( -39.99999999999999289, -114.0592624029313242, 3.246475545821551734 ) ) ;
#6626=CARTESIAN_POINT ( 'NONE',  ( -35.50000000000000000, -113.7503824761461004, 0.9631051547057219997 ) ) ;
#6640=CARTESIAN_POINT ( 'NONE',  ( -38.37230871539094323, -115.4561184093552413, 3.058975545821551290 ) ) ;
#6647=CARTESIAN_POINT ( 'NONE',  ( -35.50000000000000000, -112.9650106922503170, -2.624765990393421955 ) ) ;
#6652=CARTESIAN_POINT ( 'NONE',  ( -38.00000000000000711, -114.9929510916434339, 12.44250253426874941 ) ) ;
#6653=CARTESIAN_POINT ( 'NONE',  ( -34.50000000000000000, -114.0928965812550757, 9.511088712577292270 ) ) ;
#6656=CARTESIAN_POINT ( 'NONE',  ( -38.98077402996267438, -113.9929510916434339, 12.86289566494346204 ) ) ;
#6660=CARTESIAN_POINT ( 'NONE',  ( -36.99999999999989342, -114.9929510916434339, 13.11852480586264669 ) ) ;
#6667=CARTESIAN_POINT ( 'NONE',  ( -35.50000000000000711, -114.9927795562974069, 10.48735431211914815 ) ) ;
#6669=FACE_OUTER_BOUND ( 'NONE', #9469, .T. ) ;
#6674=CARTESIAN_POINT ( 'NONE',  ( -35.50000000000000000, -114.6807644833805000, -0.6247823525984269599 ) ) ;
#6678=CARTESIAN_POINT ( 'NONE',  ( -34.97545270896703329, -113.2308352781851539, 4.409774454178448266 ) ) ;
#6683=CARTESIAN_POINT ( 'NONE',  ( -35.50000000000000711, -112.0140978167138712, -0.4997823525984337878 ) ) ;
#6692=CARTESIAN_POINT ( 'NONE',  ( -34.50000000000000000, -116.0140978167138712, -0.1247823525984439463 ) ) ;
#6694=CARTESIAN_POINT ( 'NONE',  ( -35.50000000000000711, -113.2637153405686519, 1.912112492696748989 ) ) ;
#6702=CARTESIAN_POINT ( 'NONE',  ( -35.56312645773537895, -113.9929510916434339, 12.87038173996308998 ) ) ;
#6704=CARTESIAN_POINT ( 'NONE',  ( -35.50000000000000000, -113.9929510916434339, 12.39849696637031684 ) ) ;
#6705=CARTESIAN_POINT ( 'NONE',  ( -35.50000000000000000, -115.9929510916434481, 11.38636890470581164 ) ) ;
#6728=CARTESIAN_POINT ( 'NONE',  ( -34.50000000000000000, -114.9515981487115823, -2.624803185604625000 ) ) ;
#6732=CARTESIAN_POINT ( 'NONE',  ( -37.47347596530441649, -114.9754527089670262, 1.972274454178448932 ) ) ;
#6737=CARTESIAN_POINT ( 'NONE',  ( -35.50000000000000000, -113.0349311500474982, -0.6247823525985715110 ) ) ;
#6743=CARTESIAN_POINT ( 'NONE',  ( -35.50000000000000711, -114.9929510916434339, 11.21034663311131929 ) ) ;
#6747=CARTESIAN_POINT ( 'NONE',  ( -37.46874999999996447, -114.9929510916434339, 14.11852480586264846 ) ) ;
#6751=CARTESIAN_POINT ( 'NONE',  ( -35.50000000000000000, -115.9929510916434481, 10.85830208992344303 ) ) ;
#6752=CARTESIAN_POINT ( 'NONE',  ( -35.50000000000000711, -112.0140978167138712, -0.4685323525984295134 ) ) ;
#6763=CARTESIAN_POINT ( 'NONE',  ( -36.02454729103297382, -113.5265240346956261, 6.902725545821551734 ) ) ;
#6775=CARTESIAN_POINT ( 'NONE',  ( -34.92058450342249643, -111.8367748094582197, 5.308975545821551734 ) ) ;
#6790=CARTESIAN_POINT ( 'NONE',  ( -34.50000000000000000, -112.6043641208289188, 1.789429170677330649 ) ) ;
#6794=CARTESIAN_POINT ( 'NONE',  ( -36.03906250000000000, -115.9929510916434481, 14.11852480586265024 ) ) ;
#6797=CARTESIAN_POINT ( 'NONE',  ( -34.50000000000000000, -114.2207110452431635, 8.519246492191951958 ) ) ;
#6806=CARTESIAN_POINT ( 'NONE',  ( -34.83677480945821259, -116.0794154965774965, 4.183975545821551734 ) ) ;
#6808=CARTESIAN_POINT ( 'NONE',  ( -35.50000000000000000, -112.9990795116828650, 0.8734249692896993711 ) ) ;
#6822=CARTESIAN_POINT ( 'NONE',  ( -39.02454729103295961, -113.2308352781851397, 7.840225545821551734 ) ) ;
#6829=CARTESIAN_POINT ( 'NONE',  ( -35.50000000000000000, -112.4957190293567066, -2.560864217808777266 ) ) ;
#6834=CARTESIAN_POINT ( 'NONE',  ( -37.43749999999998579, -113.9929510916434339, 14.11852480586265024 ) ) ;
#6838=CARTESIAN_POINT ( 'NONE',  ( -39.00000000000000000, -113.9929510916434339, 12.59652202191340820 ) ) ;
#6841=CARTESIAN_POINT ( 'NONE',  ( -35.51597953369718397, -114.9929510916434339, 12.74811950270164473 ) ) ;
#6844=CARTESIAN_POINT ( 'NONE',  ( -35.00000000000000000, -113.9407375970690310, 9.996475545821589037 ) ) ;
#6848=CARTESIAN_POINT ( 'NONE',  ( -35.50000000000000711, -114.9929510916434339, 11.73841344789270202 ) ) ;
#6850=CARTESIAN_POINT ( 'NONE',  ( -38.37230871539094323, -112.5438815906447729, 2.441024454178448710 ) ) ;
#6855=CARTESIAN_POINT ( 'NONE',  ( -34.50000000000000000, -113.0140978167138712, 0.8752176474015934682 ) ) ;
#6857=CARTESIAN_POINT ( 'NONE',  ( -38.97545270896704039, -113.1123104723225197, 6.847274454178450931 ) ) ;
#6861=CARTESIAN_POINT ( 'NONE',  ( -35.62769128460905677, -115.4561184093552413, 3.191024454178449155 ) ) ;
#6864=CARTESIAN_POINT ( 'NONE',  ( -35.50000000000000711, -112.3995503592287690, -1.424448457485529618 ) ) ;
#6874=CARTESIAN_POINT ( 'NONE',  ( -34.50000000000000000, -116.0012805033554883, -0.7876962586524312027 ) ) ;
#6882=CARTESIAN_POINT ( 'NONE',  ( -35.95915003344518368, -113.9929510916434339, 13.11692036158763308 ) ) ;
#6884=CARTESIAN_POINT ( 'NONE',  ( -35.50400759022158326, -113.9929510916434339, 12.68378527132497524 ) ) ;
#6886=CARTESIAN_POINT ( 'NONE',  ( -35.50000000000000000, -115.3279708130221479, 8.997521329298534098 ) ) ;
#6896=CARTESIAN_POINT ( 'NONE',  ( -35.50000000000000711, -113.2224311500466030, -1.624782352598427959 ) ) ;
#6908=CARTESIAN_POINT ( 'NONE',  ( -34.50000000000000000, -115.1449503510569059, -2.621568770093253953 ) ) ;
#6912=CARTESIAN_POINT ( 'NONE',  ( -35.97545270896705460, -114.3549511594417680, 8.590225545821549957 ) ) ;
#6916=CARTESIAN_POINT ( 'NONE',  ( -35.50000000000000000, -115.0140978167138428, -0.6247823525986679893 ) ) ;
#6922=CARTESIAN_POINT ( 'NONE',  ( -35.50000000000000711, -114.9929510916434339, 12.50851088611648088 ) ) ;
#6926=CARTESIAN_POINT ( 'NONE',  ( -37.51022648969539119, -114.9929510916434339, 14.11852173794918386 ) ) ;
#6932=CARTESIAN_POINT ( 'NONE',  ( -36.01562499999997158, -115.9929510916434481, 13.11852480586264846 ) ) ;
#6933=CARTESIAN_POINT ( 'NONE',  ( -35.50000000000000711, -116.0012805033554883, -0.7876962586524312027 ) ) ;
#6943=CARTESIAN_POINT ( 'NONE',  ( -37.74901162816868805, -113.3347980657955958, 4.933975545821551734 ) ) ;
#6951=CARTESIAN_POINT ( 'NONE',  ( -34.92058450342249643, -111.8367748094582197, 9.808975545821553510 ) ) ;
#6969=CARTESIAN_POINT ( 'NONE',  ( -34.80050084267116972, -115.9929510916434481, 13.54034599209289347 ) ) ;
#6971=CARTESIAN_POINT ( 'NONE',  ( -35.02454729103298092, -114.8876895276775087, 1.597274454178448932 ) ) ;
#6973=CARTESIAN_POINT ( 'NONE',  ( -34.50000000000000000, -115.9929510916434481, 12.59652202191340464 ) ) ;
#6983=CARTESIAN_POINT ( 'NONE',  ( -39.97545270896702618, -115.3019030900506152, 4.652725545821551734 ) ) ;
#6985=CARTESIAN_POINT ( 'NONE',  ( -35.50000000000000000, -113.1061333991432321, 0.8862035858144284850 ) ) ;
#6993=CARTESIAN_POINT ( 'NONE',  ( -37.05926240293131713, -112.0000000000000142, 8.121475545821549957 ) ) ;
#7001=CARTESIAN_POINT ( 'NONE',  ( -35.50000000000000000, -117.0140814545088688, -0.6738694770610542673 ) ) ;
#7005=CARTESIAN_POINT ( 'NONE',  ( -37.75185693410092824, -114.9929510916434339, 13.05539834812634581 ) ) ;
#7008=CARTESIAN_POINT ( 'NONE',  ( -34.50000000000000000, -114.8211182053456838, 9.932864235516914775 ) ) ;
#7011=CARTESIAN_POINT ( 'NONE',  ( -36.31249999999995026, -114.9929510916434339, 13.11852480586264669 ) ) ;
#7013=CARTESIAN_POINT ( 'NONE',  ( -36.31249999999994316, -113.9929510916434339, 14.11852480586265024 ) ) ;
#7015=CARTESIAN_POINT ( 'NONE',  ( -37.93687354226506869, -114.9929510916434339, 12.87038173996323565 ) ) ;
#7021=CARTESIAN_POINT ( 'NONE',  ( -35.50000000000000711, -114.9929510916434339, 12.57451923796416082 ) ) ;
#7030=CARTESIAN_POINT ( 'NONE',  ( -34.50000000000000000, -113.0140978167138712, 0.8752176474015154195 ) ) ;
#7032=CARTESIAN_POINT ( 'NONE',  ( -39.02454729103295961, -114.7691647218148745, 8.159774454178448266 ) ) ;
#7034=CARTESIAN_POINT ( 'NONE',  ( -39.02454729103295961, -114.7691647218148745, 5.159774454178448266 ) ) ;
#7037=CARTESIAN_POINT ( 'NONE',  ( -35.50000000000000711, -115.9821387493194891, -0.8839717462762166633 ) ) ;
#7045=CARTESIAN_POINT ( 'NONE',  ( -34.50000000000000000, -113.0974311500471714, -1.624782352598427959 ) ) ;
#7046=CARTESIAN_POINT ( 'NONE',  ( -35.50000000000000711, -112.9185811467682754, 1.870920967077121411 ) ) ;
#7054=CARTESIAN_POINT ( 'NONE',  ( -34.50000000000000000, -113.9929510916434339, 10.50625754673586876 ) ) ;
#7058=CARTESIAN_POINT ( 'NONE',  ( -35.50000000000000000, -113.9929510916434339, 12.53051367006571581 ) ) ;
#7059=CARTESIAN_POINT ( 'NONE',  ( -35.50000000000000000, -115.1342778146718473, 8.846135899190283425 ) ) ;
#7073=CARTESIAN_POINT ( 'NONE',  ( -35.50000000000000711, -112.2144317118258527, -1.239329810084414341 ) ) ;
#7080=CARTESIAN_POINT ( 'NONE',  ( -35.50000000000000000, -113.6974040292745656, 2.970979214817929481 ) ) ;
#7084=CARTESIAN_POINT ( 'NONE',  ( -38.02454729103296671, -114.3549511594417396, 5.159774454178449155 ) ) ;
#7089=CARTESIAN_POINT ( 'NONE',  ( -35.50000000000000000, -113.6807644833805995, -0.6247823525984269599 ) ) ;
#7095=CARTESIAN_POINT ( 'NONE',  ( -36.99999999999989342, -114.9929510916434339, 13.11852480586264669 ) ) ;
#7101=CARTESIAN_POINT ( 'NONE',  ( -34.68937937320795584, -114.9929510916434339, 13.37409560816408671 ) ) ;
#7105=CARTESIAN_POINT ( 'NONE',  ( -35.96730626674924025, -115.9929510916434481, 13.11752178341330222 ) ) ;
#7106=CARTESIAN_POINT ( 'NONE',  ( -35.50000000000000711, -113.2224311500466030, -1.624782352598427959 ) ) ;
#7118=CARTESIAN_POINT ( 'NONE',  ( -35.97545270896702618, -113.6450488405582604, 5.909774454178450931 ) ) ;
#7129=CARTESIAN_POINT ( 'NONE',  ( -35.69809690994941320, -116.9754527089670546, 7.277725545821552622 ) ) ;
#7148=CARTESIAN_POINT ( 'NONE',  ( -36.50000000000010658, -115.9929510916434481, 14.11852480586265024 ) ) ;
#7151=CARTESIAN_POINT ( 'NONE',  ( -36.11231047232249836, -112.0245472910329880, 7.222274454178450043 ) ) ;
#7152=CARTESIAN_POINT ( 'NONE',  ( -34.50000000000000000, -115.9929510916434481, 10.72628538622835670 ) ) ;
#7161=CARTESIAN_POINT ( 'NONE',  ( -34.92058450342249643, -111.8367748094582197, 5.308975545821551734 ) ) ;
#7163=CARTESIAN_POINT ( 'NONE',  ( -35.50000000000000000, -113.1981689815712997, 0.8971895242272823756 ) ) ;
#7180=CARTESIAN_POINT ( 'NONE',  ( -35.50000000000000711, -112.9813730236132585, -1.624774171495860786 ) ) ;
#7184=CARTESIAN_POINT ( 'NONE',  ( -37.99839555572501837, -114.9929510916434339, 12.65937477241748965 ) ) ;
#7187=CARTESIAN_POINT ( 'NONE',  ( -34.50000000000000000, -114.9902084924877954, 10.43071793783961176 ) ) ;
#7189=CARTESIAN_POINT ( 'NONE',  ( -35.96730626674924025, -114.9929510916434339, 13.11752178341330044 ) ) ;
#7191=CARTESIAN_POINT ( 'NONE',  ( -34.50000000000000000, -114.9929501463477663, 10.50247632894551231 ) ) ;
#7193=CARTESIAN_POINT ( 'NONE',  ( -37.66108410722335265, -114.9929510916434339, 13.09299768411426790 ) ) ;
#7198=CARTESIAN_POINT ( 'NONE',  ( -36.99999999999989342, -114.9929510916434339, 13.11852480586264669 ) ) ;
#7200=CARTESIAN_POINT ( 'NONE',  ( -37.76916472181487450, -111.9754527089670404, 2.534774454178448710 ) ) ;
#7207=CARTESIAN_POINT ( 'NONE',  ( -34.50000000000000000, -113.0140978167136581, 0.8752176474015690433 ) ) ;
#7209=CARTESIAN_POINT ( 'NONE',  ( -38.45611840935523418, -115.3723087153909432, 6.566024454178448266 ) ) ;
#7211=CARTESIAN_POINT ( 'NONE',  ( -34.83677480945819838, -111.9205845034225462, 5.816024454178450043 ) ) ;
#7215=CARTESIAN_POINT ( 'NONE',  ( -35.50000000000000711, -112.0157046079661995, -0.6902086197697556713 ) ) ;
#7224=CARTESIAN_POINT ( 'NONE',  ( -34.50000000000000000, -113.3474311500483935, -1.624782352598427959 ) ) ;
#7234=CARTESIAN_POINT ( 'NONE',  ( -34.50000000000000000, -113.9836614335179377, 10.50514867547815534 ) ) ;
#7236=CARTESIAN_POINT ( 'NONE',  ( -38.00000000000000711, -113.9929510916434339, 11.91443571948719615 ) ) ;
#7237=CARTESIAN_POINT ( 'NONE',  ( -38.00000000000000711, -115.9929510916434481, 12.44250253426875119 ) ) ;
#7249=CARTESIAN_POINT ( 'NONE',  ( -35.50000000000000711, -112.8835768857893527, -1.616767172155725740 ) ) ;
#7259=CARTESIAN_POINT ( 'NONE',  ( -34.50000000000000000, -116.2431927316855109, -2.224114562372550008 ) ) ;
#7264=CARTESIAN_POINT ( 'NONE',  ( -37.74901162816869515, -114.6652019342044042, 2.066024454178448710 ) ) ;
#7271=CARTESIAN_POINT ( 'NONE',  ( -34.50000000000000000, -113.0601156079281253, 0.8807106166081309917 ) ) ;
#7278=CARTESIAN_POINT ( 'NONE',  ( -35.50000000000000000, -113.9813390189866027, 10.50487145766371100 ) ) ;
#7281=CARTESIAN_POINT ( 'NONE',  ( -35.95093014754292682, -114.9929510916434339, 14.11777216781842448 ) ) ;
#7287=CARTESIAN_POINT ( 'NONE',  ( -36.03125000000003553, -115.9929510916434481, 13.11852480586264846 ) ) ;
#7300=CARTESIAN_POINT ( 'NONE',  ( -36.94073759706866156, -113.0000000000000000, 2.628524454178448710 ) ) ;
#7311=CARTESIAN_POINT ( 'NONE',  ( -39.02454729103295961, -113.2308352781851539, 3.340225545821550845 ) ) ;
#7334=CARTESIAN_POINT ( 'NONE',  ( -34.50000000000000000, -115.9929510916434481, 12.39849696637031684 ) ) ;
#7336=CARTESIAN_POINT ( 'NONE',  ( -35.00000000000000000, -114.0592624029313242, 4.503524454178448266 ) ) ;
#7337=CARTESIAN_POINT ( 'NONE',  ( -34.50000000000000000, -115.9929510916434481, 10.52000928670414126 ) ) ;
#7351=CARTESIAN_POINT ( 'NONE',  ( -35.81662171581203324, -110.9754527089670546, 9.715225545821551734 ) ) ;
#7354=CARTESIAN_POINT ( 'NONE',  ( -35.50000000000000000, -113.0140978167138712, 0.8752176474016720720 ) ) ;
#7371=CARTESIAN_POINT ( 'NONE',  ( -35.50000000000000711, -112.7472371723319355, 1.839427296857320648 ) ) ;
#7379=CARTESIAN_POINT ( 'NONE',  ( -34.50000000000000000, -114.9819937217110635, 10.35556074009299188 ) ) ;
#7381=CARTESIAN_POINT ( 'NONE',  ( -36.00585935943767169, -114.9929510916434339, 13.11852578240983291 ) ) ;
#7383=CARTESIAN_POINT ( 'NONE',  ( -39.00000000000000000, -113.9929510916434339, 12.26648026267477221 ) ) ;
#7393=CARTESIAN_POINT ( 'NONE',  ( -35.96730626674924025, -114.9929510916434339, 13.11752178341330044 ) ) ;
#7396=CARTESIAN_POINT ( 'NONE',  ( -34.97545270896703329, -113.2308352781851539, 4.409774454178448266 ) ) ;
#7401=CARTESIAN_POINT ( 'NONE',  ( -38.37230871539094323, -112.5438815906447729, 8.441024454178448266 ) ) ;
#7403=CARTESIAN_POINT ( 'NONE',  ( -40.02454729103296671, -115.1833782841879525, 3.659774454178448710 ) ) ;
#7412=CARTESIAN_POINT ( 'NONE',  ( -34.50000000000000000, -111.0173113992184710, -0.7556348869410824953 ) ) ;
#7418=CARTESIAN_POINT ( 'NONE',  ( -38.00000000000000711, -113.9929510916434339, 12.59102132592609102 ) ) ;
#7421=CARTESIAN_POINT ( 'NONE',  ( -34.50000000000000000, -113.9557924591415627, 10.50182206170499555 ) ) ;
#7422=CARTESIAN_POINT ( 'NONE',  ( -37.24999999999992184, -115.9929510916434481, 13.11852480586264846 ) ) ;
#7432=CARTESIAN_POINT ( 'NONE',  ( -35.50000000000000711, -112.9813730236132585, -1.624774171495860786 ) ) ;
#7436=CARTESIAN_POINT ( 'NONE',  ( -35.50000000000000711, -114.6604609523327838, 9.751889438017201428 ) ) ;
#7441=CARTESIAN_POINT ( 'NONE',  ( -35.50000000000000000, -112.3070160848889429, 2.749963775944984867 ) ) ;
#7445=CARTESIAN_POINT ( 'NONE',  ( -38.99999999999999289, -113.9407375970686900, 3.753524454178449155 ) ) ;
#7450=CARTESIAN_POINT ( 'NONE',  ( -34.50000000000000000, -113.0140978167136581, -0.6247823525984261828 ) ) ;
#7453=CARTESIAN_POINT ( 'NONE',  ( -35.50000000000000000, -113.9186338266397058, 10.49738657667399266 ) ) ;
#7455=CARTESIAN_POINT ( 'NONE',  ( -34.50000000000000000, -112.0209493036498287, 0.9959249592223760050 ) ) ;
#7456=CARTESIAN_POINT ( 'NONE',  ( -34.50481333282507279, -114.9929510916434339, 12.74107470552716492 ) ) ;
#7464=CARTESIAN_POINT ( 'NONE',  ( -35.69272627125608466, -115.9929510916434481, 13.01835785830562209 ) ) ;
#7465=CARTESIAN_POINT ( 'NONE',  ( -35.50000000000000711, -114.1807644833817648, -1.624782352598427959 ) ) ;
#7476=CARTESIAN_POINT ( 'NONE',  ( -36.52652403469556930, -113.0245472910329880, 7.222274454178449155 ) ) ;
#7485=CARTESIAN_POINT ( 'NONE',  ( -39.02454729103295961, -113.2308352781851539, 6.340225545821550845 ) ) ;
#7505=CARTESIAN_POINT ( 'NONE',  ( -35.00000000000000000, -114.0000000000003411, 9.500000000000035527 ) ) ;
#7506=CARTESIAN_POINT ( 'NONE',  ( -36.11231047232249836, -112.0245472910329880, 8.722274454178448266 ) ) ;
#7508=CARTESIAN_POINT ( 'NONE',  ( -34.50000000000000000, -115.9929510916434481, 10.68227981832981044 ) ) ;
#7518=CARTESIAN_POINT ( 'NONE',  ( -37.05926240293131713, -112.0000000000000142, 3.621475545821551290 ) ) ;
#7539=CARTESIAN_POINT ( 'NONE',  ( -35.50000000000000711, -112.0140978167138712, -0.5622823525984296245 ) ) ;
#7547=CARTESIAN_POINT ( 'NONE',  ( -34.50000000000000000, -114.9929510916434339, 12.59102132592610523 ) ) ;
#7550=CARTESIAN_POINT ( 'NONE',  ( -37.42187499999997158, -114.9929510916434339, 13.11852480586264669 ) ) ;
#7553=CARTESIAN_POINT ( 'NONE',  ( -34.50000000000000000, -114.1068310684433129, 9.512752019463897923 ) ) ;
#7555=CARTESIAN_POINT ( 'NONE',  ( -38.00000000000000711, -114.9929510916434339, 12.59102132592608925 ) ) ;
#7560=CARTESIAN_POINT ( 'NONE',  ( -37.97447287825094975, -114.9929510916434339, 12.77960891308616809 ) ) ;
#7562=CARTESIAN_POINT ( 'NONE',  ( -38.37230871539094323, -112.5438815906447729, 8.441024454178448266 ) ) ;
#7568=( GEOMETRIC_REPRESENTATION_CONTEXT ( 3 ) GLOBAL_UNCERTAINTY_ASSIGNED_CONTEXT ( ( #28039 ) ) GLOBAL_UNIT_ASSIGNED_CONTEXT ( ( #17842, #34065, #31886 ) ) REPRESENTATION_CONTEXT ( 'NONE', 'WORKASPACE' ) );
#7571=CARTESIAN_POINT ( 'NONE',  ( -33.97545270896702618, -112.8166217158120475, 2.909774454178449155 ) ) ;
#7581=CARTESIAN_POINT ( 'NONE',  ( -34.50000000000000000, -111.0140978167138570, -0.4685323525984296800 ) ) ;
#7585=CARTESIAN_POINT ( 'NONE',  ( -35.50000000000000711, -114.1489256397697289, 9.518467544735724317 ) ) ;
#7586=CARTESIAN_POINT ( 'NONE',  ( -34.50000000000000000, -113.9929510916434339, 10.50625754673587409 ) ) ;
#7590=CARTESIAN_POINT ( 'NONE',  ( -37.43749999999998579, -113.9929510916434339, 13.11852480586264846 ) ) ;
#7591=CARTESIAN_POINT ( 'NONE',  ( -37.99959864031216483, -115.9929510916434481, 12.63896776382213538 ) ) ;
#7601=CARTESIAN_POINT ( 'NONE',  ( -35.50000000000000711, -112.3995503592287690, -1.424448457485529618 ) ) ;
#7603=CARTESIAN_POINT ( 'NONE',  ( -35.50000102263782509, -114.9929510916434339, 12.62466071271731316 ) ) ;
#7607=CARTESIAN_POINT ( 'NONE',  ( -35.50000000000000000, -111.0140978167138570, 0.8127176474015720409 ) ) ;
#7611=CARTESIAN_POINT ( 'NONE',  ( -35.00000000000000000, -114.0592624029313242, 1.503524454178448710 ) ) ;
#7617=CARTESIAN_POINT ( 'NONE',  ( -34.50000000000000000, -113.0974311500471714, -0.6247823525984269599 ) ) ;
#7623=CARTESIAN_POINT ( 'NONE',  ( -37.99899697755054717, -114.9929510916434339, 12.65121853911336736 ) ) ;
#7628=CARTESIAN_POINT ( 'NONE',  ( -34.50000000000000000, -113.1807644833805426, -1.624782352598427959 ) ) ;
#7635=CARTESIAN_POINT ( 'NONE',  ( -37.43749999999998579, -115.9929510916434481, 13.11852480586264846 ) ) ;
#7655=CARTESIAN_POINT ( 'NONE',  ( -38.37230871539094323, -115.4561184093552413, 6.058975545821551734 ) ) ;
#7676=CARTESIAN_POINT ( 'NONE',  ( -36.23083527818513261, -116.0245472910329880, 4.784774454178448266 ) ) ;
#7677=CARTESIAN_POINT ( 'NONE',  ( -34.50075263804418313, -115.9929510916434481, 12.66759465831979981 ) ) ;
#7686=CARTESIAN_POINT ( 'NONE',  ( -37.76916472181486739, -116.0245472910329880, 2.965225545821551290 ) ) ;
#7706=CARTESIAN_POINT ( 'NONE',  ( -35.50000000000000711, -112.9415908020655195, 1.873661708251232572 ) ) ;
#7716=CARTESIAN_POINT ( 'NONE',  ( -34.50000000000000000, -114.9927795562974069, 10.48735431211914815 ) ) ;
#7718=CARTESIAN_POINT ( 'NONE',  ( -35.93473953453761283, -114.9929510916434339, 13.11451721564123574 ) ) ;
#7720=CARTESIAN_POINT ( 'NONE',  ( -39.00000000000000000, -113.9929510916434339, 12.53051367006571937 ) ) ;
#7729=CARTESIAN_POINT ( 'NONE',  ( -38.00000000000000711, -114.9929510916434339, 12.56351784598954779 ) ) ;
#7731=CARTESIAN_POINT ( 'NONE',  ( -39.97545270896702618, -112.6980969099493990, 2.347274454178448710 ) ) ;
#7743=CARTESIAN_POINT ( 'NONE',  ( -35.81662171581204746, -117.0245472910329738, 3.284774454178449155 ) ) ;
#7755=CARTESIAN_POINT ( 'NONE',  ( -34.50000000000000000, -111.6790780953339066, 2.383953864837686343 ) ) ;
#7758=CARTESIAN_POINT ( 'NONE',  ( -35.50000000000000711, -114.1861579685891712, 9.524983039397698192 ) ) ;
#7761=CARTESIAN_POINT ( 'NONE',  ( -38.00000000000000711, -113.9929510916434339, 12.56351784598954779 ) ) ;
#7765=CARTESIAN_POINT ( 'NONE',  ( -37.99994980024369085, -113.9929510916434339, 12.62670525340494621 ) ) ;
#7767=CARTESIAN_POINT ( 'NONE',  ( -37.99359134332094357, -115.9929510916434481, 12.69998175888958514 ) ) ;
#7779=CARTESIAN_POINT ( 'NONE',  ( -35.50000000000000000, -113.0140978167138712, 0.2502176474015764263 ) ) ;
#7782=CARTESIAN_POINT ( 'NONE',  ( -35.50000000000000711, -114.9925223117477202, 10.47601618151863079 ) ) ;
#7787=CARTESIAN_POINT ( 'NONE',  ( -35.50000000000000000, -111.7850029017436810, -2.224114562373086912 ) ) ;
#7790=ADVANCED_FACE ( 'NONE', ( #34705 ), #29125, .F. ) ;
#7791=CARTESIAN_POINT ( 'NONE',  ( -35.99999999999999289, -114.0592624029313242, 6.003524454178450043 ) ) ;
#7798=CARTESIAN_POINT ( 'NONE',  ( -34.50000000000000000, -113.1807644833805426, -0.6247823525984269599 ) ) ;
#7804=CARTESIAN_POINT ( 'NONE',  ( -37.99999897736218202, -114.9929510916434339, 12.62466071271732915 ) ) ;
#7807=CARTESIAN_POINT ( 'NONE',  ( -34.50000000000000000, -114.9724313160460696, -1.624792769101446765 ) ) ;
#7812=CARTESIAN_POINT ( 'NONE',  ( -35.50000000000000711, -114.1712995509219724, 9.522174004479579068 ) ) ;
#7836=CARTESIAN_POINT ( 'NONE',  ( -36.23083527818512550, -111.9754527089670404, 5.215225545821551734 ) ) ;
#7854=CARTESIAN_POINT ( 'NONE',  ( -35.02454729103298092, -114.8876895276775087, 4.597274454178448266 ) ) ;
#7855=CARTESIAN_POINT ( 'NONE',  ( -37.18750000000004974, -115.9929510916434481, 14.11852480586265024 ) ) ;
#7867=CARTESIAN_POINT ( 'NONE',  ( -35.00000000000000000, -113.9407375970686900, 3.996475545821551290 ) ) ;
#7872=CARTESIAN_POINT ( 'NONE',  ( -34.50000000000000000, -113.0140978167156902, -0.6247823525984268489 ) ) ;
#7883=CARTESIAN_POINT ( 'NONE',  ( -36.11231047232249836, -115.9754527089670262, 8.777725545821553510 ) ) ;
#7889=CARTESIAN_POINT ( 'NONE',  ( -35.50000000000000711, -112.8835768857893527, -1.616767172155725740 ) ) ;
#7897=CARTESIAN_POINT ( 'NONE',  ( -34.50000000000000000, -112.8835768857893527, -1.616767172155725740 ) ) ;
#7899=CARTESIAN_POINT ( 'NONE',  ( -38.25557080230232998, -114.9929510916434339, 13.92914543265419525 ) ) ;
#7901=CARTESIAN_POINT ( 'NONE',  ( -38.00000000000000711, -114.9929510916434339, 12.59652202191340820 ) ) ;
#7903=CARTESIAN_POINT ( 'NONE',  ( -34.50000000000000000, -114.9929510916434339, 10.61627146648203812 ) ) ;
#7914=CARTESIAN_POINT ( 'NONE',  ( -36.01562499999996447, -114.9929510916434339, 13.11852480586264669 ) ) ;
#7916=CARTESIAN_POINT ( 'NONE',  ( -38.37230871539094323, -112.5438815906447729, 5.441024454178449155 ) ) ;
#7926=CARTESIAN_POINT ( 'NONE',  ( -38.37230871539094323, -112.5438815906447729, 8.441024454178448266 ) ) ;
#7939=CARTESIAN_POINT ( 'NONE',  ( -34.50000000000000000, -111.0141141789186605, -0.6738694770610589302 ) ) ;
#7942=CARTESIAN_POINT ( 'NONE',  ( -35.50000000000000711, -114.9929510916434339, 10.52826033068511435 ) ) ;
#7944=CARTESIAN_POINT ( 'NONE',  ( -34.50000306791346816, -113.9929510916434339, 12.62875129555796150 ) ) ;
#7948=CARTESIAN_POINT ( 'NONE',  ( -37.99999897736217491, -113.9929510916434339, 12.62466071271733092 ) ) ;
#7949=CARTESIAN_POINT ( 'NONE',  ( -36.12500000000014211, -115.9929510916434481, 13.11852480586264846 ) ) ;
#7963=CARTESIAN_POINT ( 'NONE',  ( -35.50000000000000711, -116.0140978167138712, -0.4997823525984418369 ) ) ;
#7965=CARTESIAN_POINT ( 'NONE',  ( -35.50000000000000711, -114.9927795562974069, 10.48735431211914815 ) ) ;
#7970=CARTESIAN_POINT ( 'NONE',  ( -35.50000000000000000, -111.0173113992184710, -0.7556348869410824953 ) ) ;
#7973=CARTESIAN_POINT ( 'NONE',  ( -36.52652403469556930, -113.0245472910329880, 8.722274454178450043 ) ) ;
#7981=CARTESIAN_POINT ( 'NONE',  ( -34.50000000000000000, -113.0140978167137717, -0.6411448143358797758 ) ) ;
#7987=CARTESIAN_POINT ( 'NONE',  ( -37.98402046630260287, -114.9929510916434339, 12.74811950270164118 ) ) ;
#7991=CARTESIAN_POINT ( 'NONE',  ( -34.50000000000000000, -112.9486715495423681, -1.623175561345890472 ) ) ;
#7992=CARTESIAN_POINT ( 'NONE',  ( -34.51922597003733273, -115.9929510916434481, 12.86289566494349224 ) ) ;
#7997=CARTESIAN_POINT ( 'NONE',  ( -35.50000000000000711, -114.0998638248492085, 9.511920366020609308 ) ) ;
#8017=CARTESIAN_POINT ( 'NONE',  ( -36.11231047232249125, -115.9754527089670262, 7.277725545821551734 ) ) ;
#8040=CARTESIAN_POINT ( 'NONE',  ( -38.92341863475394348, -115.9929510916434481, 13.10177712753322155 ) ) ;
#8048=CARTESIAN_POINT ( 'NONE',  ( -34.97545270896703329, -114.7691647218148745, 2.590225545821551734 ) ) ;
#8072=CARTESIAN_POINT ( 'NONE',  ( -34.50000000000000000, -112.0140978167138712, -0.3747823525984256832 ) ) ;
#8073=CARTESIAN_POINT ( 'NONE',  ( -37.52454134262690388, -114.9929510916434339, 14.11837420659362152 ) ) ;
#8075=CARTESIAN_POINT ( 'NONE',  ( -35.50000000000000000, -113.9929510916434339, 10.50625754673588474 ) ) ;
#8079=CARTESIAN_POINT ( 'NONE',  ( -34.50000000000000000, -114.9929510916434339, 12.26648026267477221 ) ) ;
#8089=CARTESIAN_POINT ( 'NONE',  ( -34.02454729103298092, -115.3019030900506294, 1.597274454178448932 ) ) ;
#8097=CARTESIAN_POINT ( 'NONE',  ( -33.97545270896702618, -112.8166217158120475, 7.409774454178449155 ) ) ;
#8109=CARTESIAN_POINT ( 'NONE',  ( -34.50000000000000000, -111.0140978167138570, -0.1247823525984260717 ) ) ;
#8111=EDGE_CURVE ( 'NONE', #12890, #18651, #9959, .T. ) ;
#8114=CARTESIAN_POINT ( 'NONE',  ( -35.50000000000000711, -114.9929517792218689, 10.50900788599415314 ) ) ;
#8115=CARTESIAN_POINT ( 'NONE',  ( -34.50000000000000000, -113.9929510916434339, 10.85830208992344303 ) ) ;
#8120=CARTESIAN_POINT ( 'NONE',  ( -34.50000000000000000, -113.9929510916434339, 11.91443571948720148 ) ) ;
#8122=CARTESIAN_POINT ( 'NONE',  ( -38.00000000000000711, -115.9929510916434481, 12.39849696637031151 ) ) ;
#8134=ORIENTED_EDGE ( 'NONE', *, *, #32143, .F. ) ;
#8135=CARTESIAN_POINT ( 'NONE',  ( -35.50000000000000000, -113.3822401464312719, 0.9191614010536472978 ) ) ;
#8137=CARTESIAN_POINT ( 'NONE',  ( -35.97545270896702618, -113.6450488405582604, 4.409774454178449155 ) ) ;
#8138=CARTESIAN_POINT ( 'NONE',  ( -35.50000000000000711, -114.9929510916434339, 10.61627146648203812 ) ) ;
#8139=FACE_OUTER_BOUND ( 'NONE', #13605, .T. ) ;
#8142=CARTESIAN_POINT ( 'NONE',  ( -35.50000000000000000, -111.0141129414446652, 0.9205922128478062350 ) ) ;
#8145=CARTESIAN_POINT ( 'NONE',  ( -38.45611840935523418, -115.3723087153909432, 3.566024454178448710 ) ) ;
#8149=CARTESIAN_POINT ( 'NONE',  ( -34.50000000000000000, -115.0140978167138712, -0.6247823525983134951 ) ) ;
#8158=CARTESIAN_POINT ( 'NONE',  ( -35.50000000000000000, -113.9929510916435618, 10.50625754673588474 ) ) ;
#8162=CARTESIAN_POINT ( 'NONE',  ( -34.50000000000000000, -114.1807644833817648, -1.624782352598427959 ) ) ;
#8164=CARTESIAN_POINT ( 'NONE',  ( -37.52454134262689678, -115.9929510916434481, 14.11837420659362152 ) ) ;
#8169=CARTESIAN_POINT ( 'NONE',  ( -37.89983305244309264, -115.9929510916434481, 12.92579853460519423 ) ) ;
#8192=CARTESIAN_POINT ( 'NONE',  ( -38.45611840935523418, -112.6276912846090568, 6.433975545821550845 ) ) ;
#8205=CARTESIAN_POINT ( 'NONE',  ( -35.50000000000000711, -114.9929510916434339, 10.51725893871048889 ) ) ;
#8213=CARTESIAN_POINT ( 'NONE',  ( -37.43749999999998579, -115.9929510916434481, 14.11852480586265024 ) ) ;
#8222=CARTESIAN_POINT ( 'NONE',  ( -37.88768952767750875, -112.0245472910329880, 8.027725545821549957 ) ) ;
#8241=ORIENTED_EDGE ( 'NONE', *, *, #29513, .F. ) ;
#8248=CARTESIAN_POINT ( 'NONE',  ( -34.50000000000000000, -112.0141059978162019, -0.6575071456984691309 ) ) ;
#8249=CARTESIAN_POINT ( 'NONE',  ( -38.98077402996267438, -114.9929510916434339, 12.86289566494346204 ) ) ;
#8251=CARTESIAN_POINT ( 'NONE',  ( -35.50000000000000000, -113.9929510916434339, 10.50625754673609258 ) ) ;
#8253=CARTESIAN_POINT ( 'NONE',  ( -34.80050084267117683, -114.9929510916434339, 13.54034599209289169 ) ) ;
#8264=CARTESIAN_POINT ( 'NONE',  ( -36.94073759706866156, -111.0000000000000284, 4.128524454178449155 ) ) ;
#8273=CARTESIAN_POINT ( 'NONE',  ( -35.69809690994941320, -116.9754527089670546, 4.277725545821552622 ) ) ;
#8284=CARTESIAN_POINT ( 'NONE',  ( -34.50000000000000000, -115.6584342456100671, -2.522673865603758614 ) ) ;
#8287=CARTESIAN_POINT ( 'NONE',  ( -36.01562499999996447, -114.9929510916434339, 13.11852480586264669 ) ) ;
#8288=CARTESIAN_POINT ( 'NONE',  ( -34.50075263804418313, -113.9929510916434339, 12.66759465831979981 ) ) ;
#8291=CARTESIAN_POINT ( 'NONE',  ( -34.50000000000000000, -113.9929510916434339, 10.50625754673587409 ) ) ;
#8293=CARTESIAN_POINT ( 'NONE',  ( -35.50000000000000711, -114.9929510916434339, 10.51725893871048889 ) ) ;
#8306=CARTESIAN_POINT ( 'NONE',  ( -35.50000000000000000, -113.0140978167138712, 0.0002176474015660057743 ) ) ;
#8308=CARTESIAN_POINT ( 'NONE',  ( -37.97545270896701908, -113.5265240346955977, 2.347274454178448710 ) ) ;
#8312=CARTESIAN_POINT ( 'NONE',  ( -35.50000000000000711, -112.0577668799241309, 1.173706424699810569 ) ) ;
#8315=CARTESIAN_POINT ( 'NONE',  ( -36.23083527818512550, -116.0245472910329880, 4.784774454178448266 ) ) ;
#8317=( LENGTH_UNIT ( ) NAMED_UNIT ( * ) SI_UNIT ( .MILLI., .METRE. ) );
#8322=CARTESIAN_POINT ( 'NONE',  ( -34.50000000000000000, -115.0140978167138712, -0.6247823525984403936 ) ) ;
#8330=CARTESIAN_POINT ( 'NONE',  ( -35.50000000000000000, -113.9929510916434339, 12.59652202191340464 ) ) ;
#8333=CARTESIAN_POINT ( 'NONE',  ( -34.50000000000000000, -111.0140978167138570, -0.4685323525984296800 ) ) ;
#8335=CARTESIAN_POINT ( 'NONE',  ( -38.99984940073100148, -115.9929510916434481, 12.64306614848957544 ) ) ;
#8340=CARTESIAN_POINT ( 'NONE',  ( -37.93687354226506869, -115.9929510916434481, 12.87038173996323565 ) ) ;
#8361=CARTESIAN_POINT ( 'NONE',  ( -35.99999999999999289, -113.9407375970686758, 2.496475545821551290 ) ) ;
#8362=EDGE_CURVE ( 'NONE', #35474, #31629, #12526, .T. ) ;
#8372=CARTESIAN_POINT ( 'NONE',  ( -35.50000000000000711, -114.1091535596544873, 9.513028657562415447 ) ) ;
#8384=CARTESIAN_POINT ( 'NONE',  ( -39.00000000000000000, -115.9929510916434481, 12.60752341388803721 ) ) ;
#8397=CARTESIAN_POINT ( 'NONE',  ( -39.02454729103295961, -113.2308352781851539, 6.340225545821550845 ) ) ;
#8406=DIRECTION ( 'NONE',  ( -1.000000000000000000, 0.000000000000000000, 0.000000000000000000 ) ) ;
#8426=CARTESIAN_POINT ( 'NONE',  ( -34.50000000000000000, -115.1446187476384040, -1.616767172155725740 ) ) ;
#8428=CARTESIAN_POINT ( 'NONE',  ( -36.07812499999994316, -114.9929510916434339, 14.11852480586264846 ) ) ;
#8431=CARTESIAN_POINT ( 'NONE',  ( -35.50000000000000000, -113.9743717753924699, 10.50403980422039396 ) ) ;
#8433=CARTESIAN_POINT ( 'NONE',  ( -36.06250000000002132, -114.9929510916434339, 14.11852480586264846 ) ) ;
#8446=CARTESIAN_POINT ( 'NONE',  ( -33.97545270896702618, -112.8166217158120475, 2.909774454178449155 ) ) ;
#8450=CARTESIAN_POINT ( 'NONE',  ( -35.50000000000000711, -115.8137639216009234, -1.239329810084483841 ) ) ;
#8457=AXIS2_PLACEMENT_3D ( 'NONE', #13974, #13804, #16302 ) ;
#8469=CARTESIAN_POINT ( 'NONE',  ( -34.50000000000000000, -117.0140978167138854, 0.6252176474015650465 ) ) ;
#8475=CARTESIAN_POINT ( 'NONE',  ( -35.50000000000000711, -114.9929510916434339, 12.59102132592610523 ) ) ;
#8478=CARTESIAN_POINT ( 'NONE',  ( -34.50000000000000000, -113.9929510916434339, 10.94631322572069365 ) ) ;
#8481=CARTESIAN_POINT ( 'NONE',  ( -34.50000000000000000, -113.9929510916434339, 10.56126450660895699 ) ) ;
#8483=CARTESIAN_POINT ( 'NONE',  ( -35.50000000000000711, -114.1068310684433129, 9.512752019463897923 ) ) ;
#8499=CARTESIAN_POINT ( 'NONE',  ( -35.50000000000000711, -115.6286452741999113, -1.424448457485488095 ) ) ;
#8501=CARTESIAN_POINT ( 'NONE',  ( -37.05926240293131713, -115.9999999999999858, 1.878524454178448710 ) ) ;
#8506=CARTESIAN_POINT ( 'NONE',  ( -35.50000000000000000, -116.9501796819249222, -1.143161139954000260 ) ) ;
#8509=CARTESIAN_POINT ( 'NONE',  ( -35.54388159064475872, -112.6276912846090568, 8.816024454178448266 ) ) ;
#8511=ORIENTED_EDGE ( 'NONE', *, *, #12960, .F. ) ;
#8513=CARTESIAN_POINT ( 'NONE',  ( -34.50000000000000000, -112.0154707866092707, 0.9357013553229778235 ) ) ;
#8518=CARTESIAN_POINT ( 'NONE',  ( -35.50000000000000000, -113.9929510916434339, 10.52000928670414126 ) ) ;
#8522=CARTESIAN_POINT ( 'NONE',  ( -34.50000000000000000, -112.3070160848889429, 2.749963775944984867 ) ) ;
#8523=CARTESIAN_POINT ( 'NONE',  ( -35.50000000000000000, -114.1556834383649459, 8.511484393387789282 ) ) ;
#8546=CARTESIAN_POINT ( 'NONE',  ( -37.97545270896702618, -114.4734759653044023, 6.152725545821551734 ) ) ;
#8551=CARTESIAN_POINT ( 'NONE',  ( -35.50000000000000711, -115.1770117227680998, -1.611965039240062181 ) ) ;
#8554=CARTESIAN_POINT ( 'NONE',  ( -35.50000000000000711, -114.5636144531578680, 9.676196722963288366 ) ) ;
#8564=CARTESIAN_POINT ( 'NONE',  ( -36.07812499999994316, -115.9929510916434481, 14.11852480586265024 ) ) ;
#8573=CARTESIAN_POINT ( 'NONE',  ( -38.37230871539094323, -115.4561184093552413, 9.058975545821551734 ) ) ;
#8599=CARTESIAN_POINT ( 'NONE',  ( -35.61121590948313553, -114.9929510916434339, 14.07058620477040733 ) ) ;
#8600=CARTESIAN_POINT ( 'NONE',  ( -35.50000000000000000, -113.9929510916434339, 10.52000928670414126 ) ) ;
#8603=CARTESIAN_POINT ( 'NONE',  ( -35.90191880024783444, -114.9929510916434339, 14.11551573851448893 ) ) ;
#8616=CARTESIAN_POINT ( 'NONE',  ( -34.00000000000000000, -114.0592624029313242, 7.503524454178450043 ) ) ;
#8619=CARTESIAN_POINT ( 'NONE',  ( -35.50000000000000711, -114.5974311500472425, -1.624782352598427959 ) ) ;
#8639=CARTESIAN_POINT ( 'NONE',  ( -35.50000000000000000, -113.8814751941374652, 2.992951091643117678 ) ) ;
#8646=CARTESIAN_POINT ( 'NONE',  ( -35.50000000000000711, -114.9929510916434339, 12.39849696637031506 ) ) ;
#8647=CARTESIAN_POINT ( 'NONE',  ( -34.50000000000000000, -113.9929510916434339, 11.38636890470581164 ) ) ;
#8648=CARTESIAN_POINT ( 'NONE',  ( -39.00000000000000711, -114.9929510916434339, 10.50625754673587231 ) ) ;
#8650=CARTESIAN_POINT ( 'NONE',  ( -34.50000000000000000, -113.9929510916434339, 10.50625754673586876 ) ) ;
#8652=CARTESIAN_POINT ( 'NONE',  ( -35.50000000000000711, -114.9929510916434339, 11.38636890470581164 ) ) ;
#8663=CARTESIAN_POINT ( 'NONE',  ( -35.50000000000000000, -113.0349311500474982, -0.6247823525985715110 ) ) ;
#8665=CARTESIAN_POINT ( 'NONE',  ( -36.94073759706868287, -112.0000000000000142, 5.628524454178449155 ) ) ;
#8674=CARTESIAN_POINT ( 'NONE',  ( -35.50000000000000711, -112.0140978167138712, 0.7189676474015718188 ) ) ;
#8677=CARTESIAN_POINT ( 'NONE',  ( -35.00000000000000000, -114.0592624029313242, 6.003524454178450043 ) ) ;
#8681=CARTESIAN_POINT ( 'NONE',  ( -34.50000000000000000, -112.0140978167138712, 0.2502176474015765373 ) ) ;
#8684=B_SPLINE_CURVE_WITH_KNOTS ( 'NONE', 3,
 ( #9227, #29529, #3844, #11934, #31191, #14804, #25811, #4698, #24125, #26471, #18526, #23758, #22904, #12108, #31853, #32041, #12957, #15454, #34938, #1806, #18349, #10263, #12780, #4863, #35116, #15806, #10439, #21398, #32395, #28319, #14615, #20183, #16164, #16529, #5739, #16697, #2521, #33281, #8072, #29696, #24299, #5566, #10965, #8248, #17215, #10610, #16339, #3044, #27182, #2876, #21751, #32927, #24999, #13838, #18698, #13490, #7897, #21932, #24650, #19224, #30228, #27540, #24825, #27354, #149, #11316, #35460, #11140, #14005, #5392, #35289, #22109, #18881, #33105, #19055, #10791, #324, #8426, #19411, #24473, #2702, #30411, #27709, #22285, #5041, #15990, #27004, #2350, #13670, #13320, #21567, #32563, #29878, #5224, #32744, #30054, #20276, #8950, #5906, #33619, #14520, #11833 ),
 .UNSPECIFIED., .F., .F.,
 ( 4, 2, 2, 2, 2, 2, 2, 2, 2, 2, 2, 2, 2, 2, 2, 2, 2, 2, 2, 2, 2, 2, 2, 2, 2, 2, 2, 2, 2, 2, 2, 2, 2, 2, 2, 2, 2, 2, 2, 2, 2, 2, 2, 2, 2, 2, 2, 2, 2, 2, 4 ),
 ( 0.000000000000000000, 0.05194669433742771930, 0.07792004150614158242, 0.09090671509049851051, 0.09740005188267697456, 0.1038933886748554386, 0.1123700156520060500, 0.1208466426291566476, 0.1377998965834578704, 0.1717064044920602883, 0.2056129124006627062, 0.2225661663549639291, 0.2310427933321145266, 0.2395194203092651519, 0.2482763131408625423, 0.2570332059724599327, 0.2745469916356546580, 0.3095745629620442196, 0.3446021342884337813, 0.3621159199516285621, 0.3708728127832259247, 0.3796297056148233429, 0.3887999023441631730, 0.3979700990735030031, 0.4163104925321826633, 0.4529912794495420392, 0.4896720663669014151, 0.5080124598255810753, 0.5171826565549209054, 0.5263528532842607355, 0.5380287103930572190, 0.5497045675018538136, 0.5730562817194468916, 0.6197597101546329368, 0.6664631385898189819, 0.6898148528074120600, 0.7014907099162086546, 0.7131665670250051381, 0.7223367637543449682, 0.7315069604836847983, 0.7498473539423643475, 0.7865281408597235568, 0.8232089277770826552, 0.8415493212357623154, 0.8507195179651021455, 0.8598897146944418646, 0.8686466075260392827, 0.8774035003576365899, 0.8949172860208314262, 0.9299448573472208768, 1.000000000000000000 ),
 .UNSPECIFIED. ) ;
#8687=CARTESIAN_POINT ( 'NONE',  ( -35.50025087934803736, -113.9929510916434339, 12.63488142334835196 ) ) ;
#8692=CARTESIAN_POINT ( 'NONE',  ( -34.50000000000000000, -112.8690837874180062, 2.872105769100646189 ) ) ;
#8693=CARTESIAN_POINT ( 'NONE',  ( -35.50000000000000000, -114.1185248058629611, 8.507048908356933836 ) ) ;
#8714=CARTESIAN_POINT ( 'NONE',  ( -38.02454729103295961, -113.6450488405582462, 3.340225545821551290 ) ) ;
#8722=CARTESIAN_POINT ( 'NONE',  ( -35.50000000000000711, -116.0140978167138712, 0.0002176474015577116276 ) ) ;
#8724=CARTESIAN_POINT ( 'NONE',  ( -35.50000000000000711, -114.3464919575557843, 9.568884482464163455 ) ) ;
#8726=CARTESIAN_POINT ( 'NONE',  ( -35.50000000000000711, -116.0140978167138712, 0.8752176474015622709 ) ) ;
#8727=CARTESIAN_POINT ( 'NONE',  ( -34.50000000000000000, -114.9929296450195721, 10.49869535309826674 ) ) ;
#8731=CARTESIAN_POINT ( 'NONE',  ( -35.50000000000000000, -115.9382890315277308, 10.02636389016632812 ) ) ;
#8733=CARTESIAN_POINT ( 'NONE',  ( -35.50000000000000711, -112.0140978167138712, 0.5627176474015717078 ) ) ;
#8740=CARTESIAN_POINT ( 'NONE',  ( -36.25098837183130485, -114.6652019342044184, 2.683975545821551734 ) ) ;
#8768=CARTESIAN_POINT ( 'NONE',  ( -34.50000000000000000, -115.0140978167138712, 0.0002176474015577929428 ) ) ;
#8772=CARTESIAN_POINT ( 'NONE',  ( -34.50000000000000000, -114.2899554544714960, 8.528375582263644006 ) ) ;
#8776=CARTESIAN_POINT ( 'NONE',  ( -37.37500000000009237, -114.9929510916434339, 14.11852480586264846 ) ) ;
#8787=CARTESIAN_POINT ( 'NONE',  ( -34.83677480945819838, -111.9205845034225462, 2.816024454178448710 ) ) ;
#8789=CARTESIAN_POINT ( 'NONE',  ( -35.50000000000000711, -112.0460568841087223, -0.8839717462762063382 ) ) ;
#8810=CARTESIAN_POINT ( 'NONE',  ( -35.50000000000000000, -111.0278007905855588, 1.116632271043183078 ) ) ;
#8815=CARTESIAN_POINT ( 'NONE',  ( -35.87040530316090070, -114.9929510916434339, 13.10254527216545917 ) ) ;
#8816=CARTESIAN_POINT ( 'NONE',  ( -38.81062062679291813, -113.9929510916434339, 13.37409560816442244 ) ) ;
#8819=CARTESIAN_POINT ( 'NONE',  ( -34.50000000000000000, -113.9929510916434623, 10.50436693183592141 ) ) ;
#8820=CARTESIAN_POINT ( 'NONE',  ( -38.25557080230232998, -114.9929510916434339, 13.92914543265419525 ) ) ;
#8822=CARTESIAN_POINT ( 'NONE',  ( -35.50000000000000711, -114.6604609523327838, 9.751889438017201428 ) ) ;
#8824=AXIS2_PLACEMENT_3D ( 'NONE', #5910, #3224, #9680 ) ;
#8837=CARTESIAN_POINT ( 'NONE',  ( -35.50000000000000000, -115.0140978167140986, -0.6247823525984417259 ) ) ;
#8839=CARTESIAN_POINT ( 'NONE',  ( -37.05926240293131713, -115.9999999999999858, 4.878524454178449155 ) ) ;
#8847=CARTESIAN_POINT ( 'NONE',  ( -35.50000000000000711, -112.0414288467712112, 1.115164475686276191 ) ) ;
#8850=CARTESIAN_POINT ( 'NONE',  ( -38.37230871539094323, -112.5438815906447729, 8.441024454178448266 ) ) ;
#8857=CARTESIAN_POINT ( 'NONE',  ( -34.50000000000000000, -115.0140978167138712, -0.4997823525984417259 ) ) ;
#8863=CARTESIAN_POINT ( 'NONE',  ( -35.50000000000000000, -113.9929510916434339, 10.50763272073269405 ) ) ;
#8867=CARTESIAN_POINT ( 'NONE',  ( -34.50000000000000000, -116.0140978167138712, -0.3122823525984417259 ) ) ;
#8869=CARTESIAN_POINT ( 'NONE',  ( -35.50000000000000000, -114.2207110452431635, 8.519246492191951958 ) ) ;
#8894=CARTESIAN_POINT ( 'NONE',  ( -35.99999999999999289, -113.9407375970686758, 3.996475545821551734 ) ) ;
#8901=CARTESIAN_POINT ( 'NONE',  ( -35.50000000000000711, -116.0141056290913610, -0.5935324770972248976 ) ) ;
#8904=CARTESIAN_POINT ( 'NONE',  ( -35.50000000000000711, -114.0650276068786582, 9.507762098804159123 ) ) ;
#8907=CARTESIAN_POINT ( 'NONE',  ( -34.50000000000000000, -114.0650276068786582, 9.507762098804159123 ) ) ;
#8913=CARTESIAN_POINT ( 'NONE',  ( -39.00000000000000000, -115.9929510916434481, 11.91443571948719615 ) ) ;
#8914=CARTESIAN_POINT ( 'NONE',  ( -35.50000000000000711, -112.6605569508015350, 1.812590711673265575 ) ) ;
#8924=CARTESIAN_POINT ( 'NONE',  ( -36.33479806579560289, -113.2509883718313262, 9.808975545821553510 ) ) ;
#8934=CARTESIAN_POINT ( 'NONE',  ( -37.05926240293133134, -116.9999999999999858, 7.878524454178450043 ) ) ;
#8948=CARTESIAN_POINT ( 'NONE',  ( -34.50000000000000000, -114.1807644833817648, -0.6247823525984269599 ) ) ;
#8950=CARTESIAN_POINT ( 'NONE',  ( -34.50000000000000000, -116.0140978167138712, -0.1247823525984439463 ) ) ;
#8953=CARTESIAN_POINT ( 'NONE',  ( -34.50000000000000000, -115.9915791193162420, 10.43066258751475139 ) ) ;
#8956=CARTESIAN_POINT ( 'NONE',  ( -37.51022648969539119, -114.9929510916434339, 14.11852173794918386 ) ) ;
#8958=DIRECTION ( 'NONE',  ( -1.000000000000000000, 0.000000000000000000, 0.000000000000000000 ) ) ;
#8966=CARTESIAN_POINT ( 'NONE',  ( -38.30190309005061522, -116.9754527089670546, 6.472274454178449155 ) ) ;
#8970=CARTESIAN_POINT ( 'NONE',  ( -35.50000000000000711, -114.9724313160460696, -1.624792769101446765 ) ) ;
#8982=CARTESIAN_POINT ( 'NONE',  ( -36.11231047232249836, -115.9754527089670262, 4.277725545821551734 ) ) ;
#8988=CARTESIAN_POINT ( 'NONE',  ( -35.50000000000000000, -111.0140978167138570, 0.7189676474015717078 ) ) ;
#8992=CARTESIAN_POINT ( 'NONE',  ( -37.48437500000004263, -114.9929510916434339, 13.11852480586264669 ) ) ;
#8996=CARTESIAN_POINT ( 'NONE',  ( -34.50000000000000000, -114.0000000000003411, 9.500000000000035527 ) ) ;
#9001=CARTESIAN_POINT ( 'NONE',  ( -36.24999999999983658, -113.9929510916434339, 14.11852480586265024 ) ) ;
#9004=CARTESIAN_POINT ( 'NONE',  ( -35.60016694755736921, -114.9929510916434339, 12.92579853460621209 ) ) ;
#9010=CARTESIAN_POINT ( 'NONE',  ( -37.98402046630260287, -115.9929510916434481, 12.74811950270164296 ) ) ;
#9021=CARTESIAN_POINT ( 'NONE',  ( -35.50000000000000000, -113.0140978167138712, -0.4997823525984338988 ) ) ;
#9023=CARTESIAN_POINT ( 'NONE',  ( -37.88768952767750164, -115.9754527089670262, 1.972274454178448710 ) ) ;
#9025=CARTESIAN_POINT ( 'NONE',  ( -35.00000000000000000, -114.0592624029313242, 1.503524454178448710 ) ) ;
#9031=CARTESIAN_POINT ( 'NONE',  ( -35.50000000000000711, -113.0796441757086939, 1.890140615870383956 ) ) ;
#9035=CARTESIAN_POINT ( 'NONE',  ( -34.97545270896703329, -113.2308352781851539, 7.409774454178451819 ) ) ;
#9041=CARTESIAN_POINT ( 'NONE',  ( -34.50000000000000000, -115.0140978167138712, -0.5622823525984408377 ) ) ;
#9050=CARTESIAN_POINT ( 'NONE',  ( -37.75185693410092824, -113.9929510916434339, 13.05539834812634759 ) ) ;
#9055=CARTESIAN_POINT ( 'NONE',  ( -34.50000000000000000, -116.0140978167138712, 0.0002176474015577116276 ) ) ;
#9057=CARTESIAN_POINT ( 'NONE',  ( -35.50000000000000000, -115.9929510916434481, 10.51175824272318415 ) ) ;
#9079=CARTESIAN_POINT ( 'NONE',  ( -37.99999999999998579, -114.0592624029313242, 4.746475545821549957 ) ) ;
#9082=AXIS2_PLACEMENT_3D ( 'NONE', #30438, #24851, #177 ) ;
#9089=CARTESIAN_POINT ( 'NONE',  ( -35.50000000000000711, -114.9724313160460696, -1.624792769101446765 ) ) ;
#9092=CARTESIAN_POINT ( 'NONE',  ( -35.50000000000000711, -114.9929510916434339, 12.44250253426871033 ) ) ;
#9097=CARTESIAN_POINT ( 'NONE',  ( -34.50000000000000000, -114.9929501463477663, 10.50247632894551231 ) ) ;
#9102=CARTESIAN_POINT ( 'NONE',  ( -35.50000000000000000, -114.4680894751352156, 8.562575367713533225 ) ) ;
#9103=CARTESIAN_POINT ( 'NONE',  ( -35.50000000000000711, -112.0577668799241309, 1.173706424699810569 ) ) ;
#9113=CARTESIAN_POINT ( 'NONE',  ( -38.02454729103295961, -113.6450488405582462, 7.840225545821554398 ) ) ;
#9121=CARTESIAN_POINT ( 'NONE',  ( -38.30190309005061522, -111.0245472910330022, 5.027725545821551734 ) ) ;
#9124=EDGE_CURVE ( 'NONE', #24733, #12890, #410, .T. ) ;
#9127=PRODUCT_CONTEXT ( 'NONE', #5043, 'mechanical' ) ;
#9134=( BOUNDED_SURFACE ( )  B_SPLINE_SURFACE ( 3, 2, ( 
 ( #28651, #31869, #15293, #26306, #20868, #1105, #26122, #1642, #23232, #9373, #6850, #7200, #1455, #12435, #12621, #34047, #15113, #3999, #17823, #34587, #14941, #4541, #15473, #1822, #25949, #12799, #33869, #9195, #2366, #29897, #34764, #7396, #23778, #13337, #35134, #32582, #10087, #35478, #13166, #32058, #27201, #19070, #7916, #29718, #21243, #32237, #21053, #30070, #18368, #5062, #24317, #21417, #35308, #18899, #2001, #13507, #10809, #29369, #12976, #18715, #4714, #15648, #26668, #16357, #16006, #23962, #5239, #21769, #27023, #34957, #18545, #10626, #21583, #10279, #7562, #2541, #16179, #24489, #10456, #5411, #4879 ),
 ( #32765, #8089, #27371, #29546, #2721, #32412, #15824, #26845, #2197, #7731, #24141, #14200, #25202, #4047, #8787, #8446, #21947, #22122, #28078, #5925, #33296, #33462, #523, #16714, #25014, #32943, #11155, #24841, #8264, #5755, #6099, #30943, #16547, #19240, #22474, #3421, #14021, #11336, #22640, #3236, #11672, #33122, #10983, #19586, #14370, #27554, #28249, #337, #19429, #19753, #22302, #33634, #30427, #8966, #167, #25377, #27725, #30765, #2892, #13685, #13856, #30245, #3065, #27891, #8616, #30590, #11504, #19934, #5584, #689, #16887, #17069, #6276, #17244, #24665, #12389, #31124, #23367, #23547, #31298, #25735 ),
 ( #20291, #34368, #31648, #20647, #25911, #15248, #4131, #11848, #6624, #26257, #1065, #22831, #6450, #865, #17421, #28605, #15070, #28422, #6806, #17594, #3957, #14900, #12215, #6983, #3763, #17955, #23192, #31826, #14719, #12034, #7161, #26082, #1238, #23008, #28958, #34185, #9509, #12576, #20468, #4304, #31482, #1413, #17777, #28781, #9690, #1597, #34009, #9333, #14537, #34543, #9861, #20823, #18135, #3589, #25551, #33827, #9151, #20115, #18322, #21727, #10582, #29321, #21533, #26982, #13463, #34722, #2324, #24274, #5012, #21371, #18669, #24103, #15778, #29668, #26797, #15966, #35260, #7351, #18855, #5196, #1774 ),
 ( #4670, #8048, #15599, #10042, #26622, #7686, #10233, #35089, #13296, #24443, #15428, #29854, #7518, #32531, #16135, #12753, #7867, #27154, #21007, #2494, #35429, #21199, #1955, #10760, #32721, #29142, #32192, #4494, #26441, #23731, #2148, #32011, #12931, #23915, #18498, #34909, #29497, #4836, #13124, #10414, #32364, #8397, #19543, #10940, #22258, #11114, #124, #22082, #27683, #11459, #21907, #480, #3022, #11624, #32900, #19201, #22598, #30548, #5709, #8222, #22426, #19378, #30384, #28030, #13981, #33418, #33079, #5880, #16670, #24974, #8573, #16846, #30201, #5537, #30029, #296, #11286, #27851, #3193, #14150, #33255 ),
 ( #16496, #33591, #8740, #27511, #19710, #25154, #3379, #24624, #30725, #6058, #17020, #14325, #25331, #647, #19030, #5367, #16314, #27325, #2850, #2671, #13634, #35611, #13812, #24800, #17918, #34141, #6943, #17375, #6236, #14862, #9649, #22783, #33963, #28913, #17552, #1370, #11998, #20420, #1021, #31256, #9463, #31434, #20070, #11804, #19888, #22963, #9292, #6763, #28740, #17739, #25872, #31081, #1196, #15202, #33786, #1548, #26037, #9113, #12346, #4093, #4262, #14493, #15034, #23321, #34320, #12170, #20608, #3909, #6578, #20247, #31608, #26211, #6408, #17198, #12531, #23507, #28559, #23144, #8924, #30901, #28207 ),
 ( #3547, #28376, #25505, #821, #3720, #14673, #25687, #32993, #31963, #8308, #20963, #13738, #7300, #19117, #23689, #13902, #12712, #4444, #18277, #13077, #15559, #4796, #32816, #19288, #20783, #44, #12891, #27425, #24716, #18091, #30117, #8137, #26396, #5454, #30298, #26578, #29279, #11034, #16406, #2774, #1916, #21996, #5636, #16595, #21153, #27607, #35533, #7118, #23873, #2942, #4625, #29095, #1728, #31784, #34679, #34861, #10859, #10001, #2100, #10184, #32148, #7476, #18455, #34500, #29453, #9820, #15739, #15384, #26757, #24062, #21819, #740, #11553, #16764, #6324, #25245, #17116, #24890, #19986, #924, #30813 ),
 ( #25605, #3288, #17293, #14591, #8501, #9023, #33686, #27775, #30991, #9201, #16933, #11386, #3642, #28298, #11905, #5976, #22882, #33875, #20163, #22521, #31170, #25425, #33170, #27938, #6499, #22347, #19476, #3115, #22171, #14065, #14246, #11722, #25061, #28122, #565, #33512, #8839, #19801, #17474, #387, #28472, #6151, #3819, #33341, #8665, #215, #22693, #3465, #19634, #11199, #14416, #30474, #5806, #30641, #7209, #17829, #26314, #6857, #1462, #4355, #1650, #25955, #17656, #25787, #28829, #4179, #15301, #34595, #12628, #31698, #1280, #7032, #21060, #4005, #7401, #31878, #14949, #18191, #23604, #34771, #20339 ) ),
 .UNSPECIFIED., .T., .F., .F. ) 
 B_SPLINE_SURFACE_WITH_KNOTS ( ( 4, 3, 4 ),
 ( 3, 2, 2, 2, 2, 2, 2, 2, 2, 2, 2, 2, 2, 2, 2, 2, 2, 2, 2, 2, 2, 2, 2, 2, 2, 2, 2, 2, 2, 2, 2, 2, 2, 2, 2, 2, 2, 2, 2, 2, 3 ),
 ( 0.000000000000000000, 0.5000000000000000000, 1.000000000000000000 ),
 ( 0.000000000000000000, 0.02500000000000000139, 0.05000000000000000278, 0.07499999999999999722, 0.1000000000000000056, 0.1250000000000000000, 0.1499999999999999944, 0.1749999999999999889, 0.2000000000000000111, 0.2250000000000000056, 0.2500000000000000000, 0.2750000000000000222, 0.2999999999999999889, 0.3250000000000000111, 0.3499999999999999778, 0.3750000000000000000, 0.4000000000000000222, 0.4249999999999999889, 0.4500000000000000111, 0.4749999999999999778, 0.5000000000000000000, 0.5250000000000000222, 0.5500000000000000444, 0.5749999999999999556, 0.5999999999999999778, 0.6250000000000000000, 0.6500000000000000222, 0.6750000000000000444, 0.6999999999999999556, 0.7249999999999999778, 0.7500000000000000000, 0.7750000000000000222, 0.8000000000000000444, 0.8249999999999999556, 0.8499999999999999778, 0.8750000000000000000, 0.9000000000000000222, 0.9250000000000000444, 0.9499999999999999556, 0.9749999999999999778, 1.000000000000000000 ),
 .UNSPECIFIED. ) 
 GEOMETRIC_REPRESENTATION_ITEM ( )  RATIONAL_B_SPLINE_SURFACE ( (
 ( 1.000000000000000000, 0.9238795325112867385, 1.000000000000000000, 0.9238795325112867385, 1.000000000000000000, 0.9238795325112867385, 1.000000000000000000, 0.9238795325112867385, 1.000000000000000000, 0.9238795325112867385, 1.000000000000000000, 0.9238795325112867385, 1.000000000000000000, 0.9238795325112867385, 1.000000000000000000, 0.9238795325112867385, 1.000000000000000000, 0.9238795325112867385, 1.000000000000000000, 0.9238795325112867385, 1.000000000000000000, 0.9238795325112867385, 1.000000000000000000, 0.9238795325112867385, 1.000000000000000000, 0.9238795325112867385, 1.000000000000000000, 0.9238795325112867385, 1.000000000000000000, 0.9238795325112867385, 1.000000000000000000, 0.9238795325112867385, 1.000000000000000000, 0.9238795325112867385, 1.000000000000000000, 0.9238795325112867385, 1.000000000000000000, 0.9238795325112867385, 1.000000000000000000, 0.9238795325112867385, 1.000000000000000000, 0.9238795325112867385, 1.000000000000000000, 0.9238795325112867385, 1.000000000000000000, 0.9238795325112867385, 1.000000000000000000, 0.9238795325112867385, 1.000000000000000000, 0.9238795325112867385, 1.000000000000000000, 0.9238795325112867385, 1.000000000000000000, 0.9238795325112867385, 1.000000000000000000, 0.9238795325112867385, 1.000000000000000000, 0.9238795325112867385, 1.000000000000000000, 0.9238795325112867385, 1.000000000000000000, 0.9238795325112867385, 1.000000000000000000, 0.9238795325112867385, 1.000000000000000000, 0.9238795325112867385, 1.000000000000000000, 0.9238795325112867385, 1.000000000000000000, 0.9238795325112867385, 1.000000000000000000, 0.9238795325112867385, 1.000000000000000000, 0.9238795325112867385, 1.000000000000000000, 0.9238795325112867385, 1.000000000000000000, 0.9238795325112867385, 1.000000000000000000, 0.9238795325112867385, 1.000000000000000000),
 ( 0.3333333333333333703, 0.3079598441704289313, 0.3333333333333333703, 0.3079598441704289313, 0.3333333333333333703, 0.3079598441704289313, 0.3333333333333333703, 0.3079598441704289313, 0.3333333333333333703, 0.3079598441704289313, 0.3333333333333333703, 0.3079598441704289313, 0.3333333333333333703, 0.3079598441704289313, 0.3333333333333333703, 0.3079598441704289313, 0.3333333333333333703, 0.3079598441704289313, 0.3333333333333333703, 0.3079598441704289313, 0.3333333333333333703, 0.3079598441704289313, 0.3333333333333333703, 0.3079598441704289313, 0.3333333333333333703, 0.3079598441704289313, 0.3333333333333333703, 0.3079598441704289313, 0.3333333333333333703, 0.3079598441704289313, 0.3333333333333333703, 0.3079598441704289313, 0.3333333333333333703, 0.3079598441704289313, 0.3333333333333333703, 0.3079598441704289313, 0.3333333333333333703, 0.3079598441704289313, 0.3333333333333333703, 0.3079598441704289313, 0.3333333333333333703, 0.3079598441704289313, 0.3333333333333333703, 0.3079598441704289313, 0.3333333333333333703, 0.3079598441704289313, 0.3333333333333333703, 0.3079598441704289313, 0.3333333333333333703, 0.3079598441704289313, 0.3333333333333333703, 0.3079598441704289313, 0.3333333333333333703, 0.3079598441704289313, 0.3333333333333333703, 0.3079598441704289313, 0.3333333333333333703, 0.3079598441704289313, 0.3333333333333333703, 0.3079598441704289313, 0.3333333333333333703, 0.3079598441704289313, 0.3333333333333333703, 0.3079598441704289313, 0.3333333333333333703, 0.3079598441704289313, 0.3333333333333333703, 0.3079598441704289313, 0.3333333333333333703, 0.3079598441704289313, 0.3333333333333333703, 0.3079598441704289313, 0.3333333333333333703, 0.3079598441704289313, 0.3333333333333333703, 0.3079598441704289313, 0.3333333333333333703, 0.3079598441704289313, 0.3333333333333333703, 0.3079598441704289313, 0.3333333333333333703),
 ( 0.3333333333333333703, 0.3079598441704289313, 0.3333333333333333703, 0.3079598441704289313, 0.3333333333333333703, 0.3079598441704289313, 0.3333333333333333703, 0.3079598441704289313, 0.3333333333333333703, 0.3079598441704289313, 0.3333333333333333703, 0.3079598441704289313, 0.3333333333333333703, 0.3079598441704289313, 0.3333333333333333703, 0.3079598441704289313, 0.3333333333333333703, 0.3079598441704289313, 0.3333333333333333703, 0.3079598441704289313, 0.3333333333333333703, 0.3079598441704289313, 0.3333333333333333703, 0.3079598441704289313, 0.3333333333333333703, 0.3079598441704289313, 0.3333333333333333703, 0.3079598441704289313, 0.3333333333333333703, 0.3079598441704289313, 0.3333333333333333703, 0.3079598441704289313, 0.3333333333333333703, 0.3079598441704289313, 0.3333333333333333703, 0.3079598441704289313, 0.3333333333333333703, 0.3079598441704289313, 0.3333333333333333703, 0.3079598441704289313, 0.3333333333333333703, 0.3079598441704289313, 0.3333333333333333703, 0.3079598441704289313, 0.3333333333333333703, 0.3079598441704289313, 0.3333333333333333703, 0.3079598441704289313, 0.3333333333333333703, 0.3079598441704289313, 0.3333333333333333703, 0.3079598441704289313, 0.3333333333333333703, 0.3079598441704289313, 0.3333333333333333703, 0.3079598441704289313, 0.3333333333333333703, 0.3079598441704289313, 0.3333333333333333703, 0.3079598441704289313, 0.3333333333333333703, 0.3079598441704289313, 0.3333333333333333703, 0.3079598441704289313, 0.3333333333333333703, 0.3079598441704289313, 0.3333333333333333703, 0.3079598441704289313, 0.3333333333333333703, 0.3079598441704289313, 0.3333333333333333703, 0.3079598441704289313, 0.3333333333333333703, 0.3079598441704289313, 0.3333333333333333703, 0.3079598441704289313, 0.3333333333333333703, 0.3079598441704289313, 0.3333333333333333703, 0.3079598441704289313, 0.3333333333333333703),
 ( 1.000000000000000000, 0.9238795325112867385, 1.000000000000000000, 0.9238795325112867385, 1.000000000000000000, 0.9238795325112867385, 1.000000000000000000, 0.9238795325112867385, 1.000000000000000000, 0.9238795325112867385, 1.000000000000000000, 0.9238795325112867385, 1.000000000000000000, 0.9238795325112867385, 1.000000000000000000, 0.9238795325112867385, 1.000000000000000000, 0.9238795325112867385, 1.000000000000000000, 0.9238795325112867385, 1.000000000000000000, 0.9238795325112867385, 1.000000000000000000, 0.9238795325112867385, 1.000000000000000000, 0.9238795325112867385, 1.000000000000000000, 0.9238795325112867385, 1.000000000000000000, 0.9238795325112867385, 1.000000000000000000, 0.9238795325112867385, 1.000000000000000000, 0.9238795325112867385, 1.000000000000000000, 0.9238795325112867385, 1.000000000000000000, 0.9238795325112867385, 1.000000000000000000, 0.9238795325112867385, 1.000000000000000000, 0.9238795325112867385, 1.000000000000000000, 0.9238795325112867385, 1.000000000000000000, 0.9238795325112867385, 1.000000000000000000, 0.9238795325112867385, 1.000000000000000000, 0.9238795325112867385, 1.000000000000000000, 0.9238795325112867385, 1.000000000000000000, 0.9238795325112867385, 1.000000000000000000, 0.9238795325112867385, 1.000000000000000000, 0.9238795325112867385, 1.000000000000000000, 0.9238795325112867385, 1.000000000000000000, 0.9238795325112867385, 1.000000000000000000, 0.9238795325112867385, 1.000000000000000000, 0.9238795325112867385, 1.000000000000000000, 0.9238795325112867385, 1.000000000000000000, 0.9238795325112867385, 1.000000000000000000, 0.9238795325112867385, 1.000000000000000000, 0.9238795325112867385, 1.000000000000000000, 0.9238795325112867385, 1.000000000000000000, 0.9238795325112867385, 1.000000000000000000, 0.9238795325112867385, 1.000000000000000000),
 ( 0.3333333333333333703, 0.3079598441704289313, 0.3333333333333333703, 0.3079598441704289313, 0.3333333333333333703, 0.3079598441704289313, 0.3333333333333333703, 0.3079598441704289313, 0.3333333333333333703, 0.3079598441704289313, 0.3333333333333333703, 0.3079598441704289313, 0.3333333333333333703, 0.3079598441704289313, 0.3333333333333333703, 0.3079598441704289313, 0.3333333333333333703, 0.3079598441704289313, 0.3333333333333333703, 0.3079598441704289313, 0.3333333333333333703, 0.3079598441704289313, 0.3333333333333333703, 0.3079598441704289313, 0.3333333333333333703, 0.3079598441704289313, 0.3333333333333333703, 0.3079598441704289313, 0.3333333333333333703, 0.3079598441704289313, 0.3333333333333333703, 0.3079598441704289313, 0.3333333333333333703, 0.3079598441704289313, 0.3333333333333333703, 0.3079598441704289313, 0.3333333333333333703, 0.3079598441704289313, 0.3333333333333333703, 0.3079598441704289313, 0.3333333333333333703, 0.3079598441704289313, 0.3333333333333333703, 0.3079598441704289313, 0.3333333333333333703, 0.3079598441704289313, 0.3333333333333333703, 0.3079598441704289313, 0.3333333333333333703, 0.3079598441704289313, 0.3333333333333333703, 0.3079598441704289313, 0.3333333333333333703, 0.3079598441704289313, 0.3333333333333333703, 0.3079598441704289313, 0.3333333333333333703, 0.3079598441704289313, 0.3333333333333333703, 0.3079598441704289313, 0.3333333333333333703, 0.3079598441704289313, 0.3333333333333333703, 0.3079598441704289313, 0.3333333333333333703, 0.3079598441704289313, 0.3333333333333333703, 0.3079598441704289313, 0.3333333333333333703, 0.3079598441704289313, 0.3333333333333333703, 0.3079598441704289313, 0.3333333333333333703, 0.3079598441704289313, 0.3333333333333333703, 0.3079598441704289313, 0.3333333333333333703, 0.3079598441704289313, 0.3333333333333333703, 0.3079598441704289313, 0.3333333333333333703),
 ( 0.3333333333333333703, 0.3079598441704289313, 0.3333333333333333703, 0.3079598441704289313, 0.3333333333333333703, 0.3079598441704289313, 0.3333333333333333703, 0.3079598441704289313, 0.3333333333333333703, 0.3079598441704289313, 0.3333333333333333703, 0.3079598441704289313, 0.3333333333333333703, 0.3079598441704289313, 0.3333333333333333703, 0.3079598441704289313, 0.3333333333333333703, 0.3079598441704289313, 0.3333333333333333703, 0.3079598441704289313, 0.3333333333333333703, 0.3079598441704289313, 0.3333333333333333703, 0.3079598441704289313, 0.3333333333333333703, 0.3079598441704289313, 0.3333333333333333703, 0.3079598441704289313, 0.3333333333333333703, 0.3079598441704289313, 0.3333333333333333703, 0.3079598441704289313, 0.3333333333333333703, 0.3079598441704289313, 0.3333333333333333703, 0.3079598441704289313, 0.3333333333333333703, 0.3079598441704289313, 0.3333333333333333703, 0.3079598441704289313, 0.3333333333333333703, 0.3079598441704289313, 0.3333333333333333703, 0.3079598441704289313, 0.3333333333333333703, 0.3079598441704289313, 0.3333333333333333703, 0.3079598441704289313, 0.3333333333333333703, 0.3079598441704289313, 0.3333333333333333703, 0.3079598441704289313, 0.3333333333333333703, 0.3079598441704289313, 0.3333333333333333703, 0.3079598441704289313, 0.3333333333333333703, 0.3079598441704289313, 0.3333333333333333703, 0.3079598441704289313, 0.3333333333333333703, 0.3079598441704289313, 0.3333333333333333703, 0.3079598441704289313, 0.3333333333333333703, 0.3079598441704289313, 0.3333333333333333703, 0.3079598441704289313, 0.3333333333333333703, 0.3079598441704289313, 0.3333333333333333703, 0.3079598441704289313, 0.3333333333333333703, 0.3079598441704289313, 0.3333333333333333703, 0.3079598441704289313, 0.3333333333333333703, 0.3079598441704289313, 0.3333333333333333703, 0.3079598441704289313, 0.3333333333333333703),
 ( 1.000000000000000000, 0.9238795325112867385, 1.000000000000000000, 0.9238795325112867385, 1.000000000000000000, 0.9238795325112867385, 1.000000000000000000, 0.9238795325112867385, 1.000000000000000000, 0.9238795325112867385, 1.000000000000000000, 0.9238795325112867385, 1.000000000000000000, 0.9238795325112867385, 1.000000000000000000, 0.9238795325112867385, 1.000000000000000000, 0.9238795325112867385, 1.000000000000000000, 0.9238795325112867385, 1.000000000000000000, 0.9238795325112867385, 1.000000000000000000, 0.9238795325112867385, 1.000000000000000000, 0.9238795325112867385, 1.000000000000000000, 0.9238795325112867385, 1.000000000000000000, 0.9238795325112867385, 1.000000000000000000, 0.9238795325112867385, 1.000000000000000000, 0.9238795325112867385, 1.000000000000000000, 0.9238795325112867385, 1.000000000000000000, 0.9238795325112867385, 1.000000000000000000, 0.9238795325112867385, 1.000000000000000000, 0.9238795325112867385, 1.000000000000000000, 0.9238795325112867385, 1.000000000000000000, 0.9238795325112867385, 1.000000000000000000, 0.9238795325112867385, 1.000000000000000000, 0.9238795325112867385, 1.000000000000000000, 0.9238795325112867385, 1.000000000000000000, 0.9238795325112867385, 1.000000000000000000, 0.9238795325112867385, 1.000000000000000000, 0.9238795325112867385, 1.000000000000000000, 0.9238795325112867385, 1.000000000000000000, 0.9238795325112867385, 1.000000000000000000, 0.9238795325112867385, 1.000000000000000000, 0.9238795325112867385, 1.000000000000000000, 0.9238795325112867385, 1.000000000000000000, 0.9238795325112867385, 1.000000000000000000, 0.9238795325112867385, 1.000000000000000000, 0.9238795325112867385, 1.000000000000000000, 0.9238795325112867385, 1.000000000000000000, 0.9238795325112867385, 1.000000000000000000, 0.9238795325112867385, 1.000000000000000000) ) ) 
 REPRESENTATION_ITEM ( '' )  SURFACE ( )  );
#9137=CARTESIAN_POINT ( 'NONE',  ( -34.50000000000000000, -115.0140978167143402, -0.6247823525984417259 ) ) ;
#9140=CARTESIAN_POINT ( 'NONE',  ( -34.50000000000000000, -115.3279708130221479, 8.997521329298534098 ) ) ;
#9142=CARTESIAN_POINT ( 'NONE',  ( -38.45611840935523418, -115.3723087153909432, 2.066024454178448710 ) ) ;
#9143=CARTESIAN_POINT ( 'NONE',  ( -34.50000000000000000, -114.2253558743059330, 8.519800927820798009 ) ) ;
#9151=CARTESIAN_POINT ( 'NONE',  ( -39.99999999999999289, -114.0592624029313242, 7.746475545821553510 ) ) ;
#9153=CARTESIAN_POINT ( 'NONE',  ( -35.50000000000000711, -116.0140978167138712, -0.5622823525984409487 ) ) ;
#9164=ORIENTED_EDGE ( 'NONE', *, *, #2909, .F. ) ;
#9166=CARTESIAN_POINT ( 'NONE',  ( -37.76916472181486739, -116.0245472910329880, 7.465225545821551734 ) ) ;
#9171=CARTESIAN_POINT ( 'NONE',  ( -35.50000000000000000, -113.0974311500471714, -2.624782352598442614 ) ) ;
#9176=CARTESIAN_POINT ( 'NONE',  ( -37.99599240977853754, -114.9929510916434339, 12.68378527132499478 ) ) ;
#9178=CARTESIAN_POINT ( 'NONE',  ( -39.00000000000000000, -113.9929510916434339, 12.53051367006571937 ) ) ;
#9183=CARTESIAN_POINT ( 'NONE',  ( -38.42182118622945808, -113.9929510916434339, 13.81802396319329773 ) ) ;
#9186=CARTESIAN_POINT ( 'NONE',  ( -35.50025087934803736, -114.9929510916434339, 12.63488142334835196 ) ) ;
#9192=CARTESIAN_POINT ( 'NONE',  ( -35.50000000000000711, -114.9929510916434339, 12.50851088611648088 ) ) ;
#9195=CARTESIAN_POINT ( 'NONE',  ( -37.76916472181487450, -111.9754527089670404, 4.034774454178449155 ) ) ;
#9199=CARTESIAN_POINT ( 'NONE',  ( -34.50000000000000000, -114.1185248058627053, 1.007048908356900085 ) ) ;
#9201=CARTESIAN_POINT ( 'NONE',  ( -38.97545270896704039, -113.1123104723225197, 2.347274454178448710 ) ) ;
#9204=CARTESIAN_POINT ( 'NONE',  ( -35.00000000000000000, -114.0592624029313242, 3.003524454178448710 ) ) ;
#9208=CARTESIAN_POINT ( 'NONE',  ( -35.50000000000000711, -112.0460568841087223, -0.8839717462762063382 ) ) ;
#9219=CARTESIAN_POINT ( 'NONE',  ( -34.50000000000000000, -112.2144317118258527, -1.239329810084414341 ) ) ;
#9220=CARTESIAN_POINT ( 'NONE',  ( -35.50000000000000711, -112.0140978167138712, 0.5627176474015717078 ) ) ;
#9226=CARTESIAN_POINT ( 'NONE',  ( -35.87040530316090070, -113.9929510916434339, 13.10254527216545917 ) ) ;
#9227=CARTESIAN_POINT ( 'NONE',  ( -34.50000000000000000, -114.0000000000000853, 2.000000000000001776 ) ) ;
#9230=CARTESIAN_POINT ( 'NONE',  ( -36.06250000000000711, -113.9929510916434339, 13.11852480586264846 ) ) ;
#9231=CARTESIAN_POINT ( 'NONE',  ( -35.50000000000000000, -115.9929510916434481, 11.91443571948720148 ) ) ;
#9254=CARTESIAN_POINT ( 'NONE',  ( -34.50000000000000000, -115.6584342456100671, -2.522673865603758614 ) ) ;
#9259=CARTESIAN_POINT ( 'NONE',  ( -35.97545270896702618, -113.6450488405582604, 4.409774454178449155 ) ) ;
#9269=EDGE_CURVE ( 'NONE', #12261, #18157, #12223, .T. ) ;
#9271=CARTESIAN_POINT ( 'NONE',  ( -35.69272627125609176, -114.9929510916434339, 13.01835785830562209 ) ) ;
#9274=CARTESIAN_POINT ( 'NONE',  ( -34.50000000000000000, -114.9929510916434339, 10.68227981832981044 ) ) ;
#9278=CARTESIAN_POINT ( 'NONE',  ( -35.50000000000000000, -114.7000328234681206, 8.631511418192262752 ) ) ;
#9279=CARTESIAN_POINT ( 'NONE',  ( -35.50000000000000711, -113.0106174888879877, 1.881901162060937827 ) ) ;
#9292=CARTESIAN_POINT ( 'NONE',  ( -36.33479806579560289, -113.2509883718313262, 6.808975545821551734 ) ) ;
#9302=CARTESIAN_POINT ( 'NONE',  ( -35.69809690994941320, -116.9754527089670546, 2.777725545821551734 ) ) ;
#9318=CARTESIAN_POINT ( 'NONE',  ( -34.50000000000000000, -112.7472371723319355, 1.839427296857320648 ) ) ;
#9321=CARTESIAN_POINT ( 'NONE',  ( -34.50000000000000000, -115.9929510916434481, 10.72628538622835670 ) ) ;
#9323=CARTESIAN_POINT ( 'NONE',  ( -35.00000000000000000, -114.0592624029313953, 1.503524454178449599 ) ) ;
#9324=CARTESIAN_POINT ( 'NONE',  ( -37.49023442168701337, -114.9929510916434339, 14.11852773550420359 ) ) ;
#9333=CARTESIAN_POINT ( 'NONE',  ( -34.02454729103297382, -112.6980969099494132, 6.902725545821551734 ) ) ;
#9335=CARTESIAN_POINT ( 'NONE',  ( -35.50000000000000000, -113.0140978167136581, 0.8752176474015690433 ) ) ;
#9348=CARTESIAN_POINT ( 'NONE',  ( -38.97545270896704039, -114.8876895276775087, 6.152725545821551734 ) ) ;
#9353=CARTESIAN_POINT ( 'NONE',  ( -35.50000000000000000, -117.0141134414687514, -0.5779076015960331603 ) ) ;
#9356=CARTESIAN_POINT ( 'NONE',  ( -38.00000068757622529, -114.9929510916434339, 12.61439929482944855 ) ) ;
#9358=CARTESIAN_POINT ( 'NONE',  ( -37.74437085908086686, -113.9929510916434339, 14.09929883582536903 ) ) ;
#9363=CARTESIAN_POINT ( 'NONE',  ( -38.81062062679291813, -113.9929510916434339, 13.37409560816442244 ) ) ;
#9365=CARTESIAN_POINT ( 'NONE',  ( -36.31249999999995026, -114.9929510916434339, 13.11852480586264669 ) ) ;
#9371=CARTESIAN_POINT ( 'NONE',  ( -35.50000000000000711, -114.9656200615856818, 10.26631071845107179 ) ) ;
#9373=CARTESIAN_POINT ( 'NONE',  ( -38.97545270896704039, -113.1123104723225197, 2.347274454178448710 ) ) ;
#9379=CARTESIAN_POINT ( 'NONE',  ( -35.50000000000000000, -113.1807644833805426, -0.6247823525984269599 ) ) ;
#9383=CARTESIAN_POINT ( 'NONE',  ( -37.05926240293131713, -115.9999999999999858, 3.378524454178448710 ) ) ;
#9386=CARTESIAN_POINT ( 'NONE',  ( -35.50000000000000711, -112.6919296022648638, -1.573728109100751116 ) ) ;
#9391=( NAMED_UNIT ( * ) SI_UNIT ( $, .STERADIAN. ) SOLID_ANGLE_UNIT ( ) );
#9395=CARTESIAN_POINT ( 'NONE',  ( -34.50000000000000000, -114.8057644833805568, -1.624782352598427959 ) ) ;
#9396=FACE_OUTER_BOUND ( 'NONE', #27636, .T. ) ;
#9401=CARTESIAN_POINT ( 'NONE',  ( -37.49414064056232831, -113.9929510916434339, 13.11852578240983291 ) ) ;
#9404=CARTESIAN_POINT ( 'NONE',  ( -35.50000000000000000, -113.9929510916434339, 10.56126450660895699 ) ) ;
#9405=CARTESIAN_POINT ( 'NONE',  ( -35.50000000000000000, -115.9929510916434481, 12.39849696637031684 ) ) ;
#9417=CARTESIAN_POINT ( 'NONE',  ( -35.50000000000000711, -113.0106174888879877, 1.881901162060937827 ) ) ;
#9425=CARTESIAN_POINT ( 'NONE',  ( -34.50000000000000000, -117.0140814545088688, -0.6738694770610542673 ) ) ;
#9429=CARTESIAN_POINT ( 'NONE',  ( -36.64504884055823908, -115.0245472910329880, 4.784774454178448266 ) ) ;
#9434=CARTESIAN_POINT ( 'NONE',  ( -35.50000000000000000, -114.9307644833806137, -0.6247823525984269599 ) ) ;
#9440=CARTESIAN_POINT ( 'NONE',  ( -35.50160444427493189, -114.9929510916434339, 12.65937477241749853 ) ) ;
#9443=CARTESIAN_POINT ( 'NONE',  ( -36.03125000000004263, -114.9929510916434339, 14.11852480586264846 ) ) ;
#9450=CARTESIAN_POINT ( 'NONE',  ( -39.00000000000000000, -115.9929510916434481, 12.44250253426875119 ) ) ;
#9463=CARTESIAN_POINT ( 'NONE',  ( -37.99999999999998579, -114.0592624029313242, 6.246475545821551734 ) ) ;
#9469=EDGE_LOOP ( 'NONE', ( #9734, #10298, #730, #11211, #16017, #16178 ) ) ;
#9473=CARTESIAN_POINT ( 'NONE',  ( -37.05926240293131713, -111.0000000000000284, 6.621475545821551734 ) ) ;
#9491=CARTESIAN_POINT ( 'NONE',  ( -34.50000000000000000, -113.8159288351371714, 1.978028123174813802 ) ) ;
#9495=CARTESIAN_POINT ( 'NONE',  ( -34.50000000000000000, -114.7000328234681206, 8.631511418192262752 ) ) ;
#9501=CARTESIAN_POINT ( 'NONE',  ( -38.99924736195578134, -114.9929510916434339, 12.66759465831984777 ) ) ;
#9509=CARTESIAN_POINT ( 'NONE',  ( -36.94073759706868287, -116.9999999999999858, 5.871475545821551734 ) ) ;
#9511=CARTESIAN_POINT ( 'NONE',  ( -35.50000000000000000, -113.0140978167139991, 0.8595926474015699315 ) ) ;
#9524=CARTESIAN_POINT ( 'NONE',  ( -37.05926240293131713, -112.0000000000000142, 6.621475545821550845 ) ) ;
#9531=CARTESIAN_POINT ( 'NONE',  ( -35.50000000000000000, -111.0173113992184710, -0.7556348869410824953 ) ) ;
#9537=CARTESIAN_POINT ( 'NONE',  ( -37.99994980024369085, -114.9929510916434339, 12.62670525340494621 ) ) ;
#9538=CARTESIAN_POINT ( 'NONE',  ( -34.50000000000000000, -114.1091535596544873, 9.513028657562415447 ) ) ;
#9544=CARTESIAN_POINT ( 'NONE',  ( -39.00000206272865455, -113.9929510916434339, 12.61164896875035879 ) ) ;
#9547=CARTESIAN_POINT ( 'NONE',  ( -35.50000000000000711, -114.9929510916434339, 12.26648026267477221 ) ) ;
#9553=CARTESIAN_POINT ( 'NONE',  ( -35.50000000000000711, -114.9929510916434339, 10.55026311463432087 ) ) ;
#9560=CARTESIAN_POINT ( 'NONE',  ( -34.50000000000000000, -113.3822401464312719, 0.9191614010536472978 ) ) ;
#9564=CARTESIAN_POINT ( 'NONE',  ( -35.00000000000000000, -114.0592624029313242, 6.003524454178450043 ) ) ;
#9568=CARTESIAN_POINT ( 'NONE',  ( -35.50000000000000711, -112.0140978167138712, 0.2502176474015765373 ) ) ;
#9578=CARTESIAN_POINT ( 'NONE',  ( -34.50000000000000000, -114.6807644833805000, -1.624782352598427959 ) ) ;
#9580=CARTESIAN_POINT ( 'NONE',  ( -35.50000000000000711, -112.6605569508015350, 1.812590711673265575 ) ) ;
#9588=CARTESIAN_POINT ( 'NONE',  ( -35.97955704204053262, -113.9929510916434339, 13.11812344617474402 ) ) ;
#9590=CARTESIAN_POINT ( 'NONE',  ( -36.24999999999983658, -113.9929510916434339, 13.11852480586264846 ) ) ;
#9591=CARTESIAN_POINT ( 'NONE',  ( -35.50000000000000000, -115.9929510916434481, 12.59652202191340464 ) ) ;
#9603=CARTESIAN_POINT ( 'NONE',  ( -35.50000000000000711, -113.0974311500471714, -1.624782352598427959 ) ) ;
#9611=CARTESIAN_POINT ( 'NONE',  ( -34.50000000000000000, -114.3474311500471572, -2.624782352598442614 ) ) ;
#9615=CARTESIAN_POINT ( 'NONE',  ( -37.99999999999998579, -114.0592624029313242, 9.246475545821549957 ) ) ;
#9621=CARTESIAN_POINT ( 'NONE',  ( -34.50000000000000000, -113.0140978167140702, 0.8752176474015603835 ) ) ;
#9627=CARTESIAN_POINT ( 'NONE',  ( -36.15625000000007816, -114.9929510916434339, 13.11852480586264669 ) ) ;
#9633=CARTESIAN_POINT ( 'NONE',  ( -34.50075263804418313, -114.9929510916434339, 12.66759465831979981 ) ) ;
#9638=CARTESIAN_POINT ( 'NONE',  ( -36.03906250000000000, -115.9929510916434481, 13.11852480586264846 ) ) ;
#9639=CARTESIAN_POINT ( 'NONE',  ( -35.50000000000000711, -112.8835768857893527, -1.616767172155725740 ) ) ;
#9649=CARTESIAN_POINT ( 'NONE',  ( -36.33479806579560289, -113.2509883718313262, 5.308975545821551734 ) ) ;
#9659=CARTESIAN_POINT ( 'NONE',  ( -39.97545270896702618, -115.3019030900506152, 6.152725545821551734 ) ) ;
#9679=CARTESIAN_POINT ( 'NONE',  ( -35.90191880024782023, -115.9929510916434481, 14.11551573851449071 ) ) ;
#9680=DIRECTION ( 'NONE',  ( 1.000000000000000000, 0.000000000000000000, 0.000000000000000000 ) ) ;
#9682=CARTESIAN_POINT ( 'NONE',  ( -39.00000000000000711, -114.9929510916434339, 12.59652202191340820 ) ) ;
#9690=CARTESIAN_POINT ( 'NONE',  ( -37.05926240293131713, -111.0000000000000284, 6.621475545821551734 ) ) ;
#9693=CARTESIAN_POINT ( 'NONE',  ( -35.50000000000000000, -113.4742757288593964, 0.9301473394660054739 ) ) ;
#9705=CARTESIAN_POINT ( 'NONE',  ( -38.45611840935523418, -112.6276912846090568, 7.933975545821552622 ) ) ;
#9711=CARTESIAN_POINT ( 'NONE',  ( -35.50000000000000000, -117.0140978167138854, 0.0002176474015578471800 ) ) ;
#9718=CARTESIAN_POINT ( 'NONE',  ( -34.50000000000000000, -114.9929510916434339, 12.50851088611648088 ) ) ;
#9720=CARTESIAN_POINT ( 'NONE',  ( -37.34375000000001421, -114.9929510916434339, 13.11852480586264669 ) ) ;
#9722=CARTESIAN_POINT ( 'NONE',  ( -36.06250000000000711, -113.9929510916434339, 14.11852480586265024 ) ) ;
#9724=CARTESIAN_POINT ( 'NONE',  ( -37.49414064056234253, -114.9929510916434339, 13.11852578240983291 ) ) ;
#9730=CARTESIAN_POINT ( 'NONE',  ( -35.50000000000000711, -114.9929510916434339, 12.53051367006571581 ) ) ;
#9734=ORIENTED_EDGE ( 'NONE', *, *, #22366, .T. ) ;
#9737=CARTESIAN_POINT ( 'NONE',  ( -34.50000000000000000, -113.1981689815712997, 0.8971895242272823756 ) ) ;
#9743=CARTESIAN_POINT ( 'NONE',  ( -37.05926240293131713, -115.9999999999999858, 4.878524454178449155 ) ) ;
#9745=CARTESIAN_POINT ( 'NONE',  ( -35.50000000000000711, -115.8878449012421754, -1.128496220799388494 ) ) ;
#9756=CARTESIAN_POINT ( 'NONE',  ( -34.50000000000000000, -114.8474311500471572, -1.624782352598427959 ) ) ;
#9757=CARTESIAN_POINT ( 'NONE',  ( -35.50000000000000711, -112.0140978167138712, 0.8127176474015721519 ) ) ;
#9765=CARTESIAN_POINT ( 'NONE',  ( -37.97447287825094264, -113.9929510916434339, 12.77960891308616809 ) ) ;
#9767=CARTESIAN_POINT ( 'NONE',  ( -35.91854304697312728, -113.9929510916434339, 13.11211614918345703 ) ) ;
#9768=CARTESIAN_POINT ( 'NONE',  ( -35.50000000000000000, -115.9929510916434481, 10.52826033068511435 ) ) ;
#9780=CARTESIAN_POINT ( 'NONE',  ( -35.50000000000000711, -112.7472371723319355, 1.839427296857320648 ) ) ;
#9787=CARTESIAN_POINT ( 'NONE',  ( -34.50000000000000000, -117.0140978167138854, 0.8752176474015623819 ) ) ;
#9792=CARTESIAN_POINT ( 'NONE',  ( -37.97545270896701908, -113.5265240346955977, 2.347274454178448710 ) ) ;
#9796=CARTESIAN_POINT ( 'NONE',  ( -35.50000000000000000, -115.0140978167138712, -0.6247823525983134951 ) ) ;
#9800=CARTESIAN_POINT ( 'NONE',  ( -35.99386409314529800, -114.9929510916434339, 13.11852378322482515 ) ) ;
#9804=CARTESIAN_POINT ( 'NONE',  ( -37.62254989966454133, -114.9929510916434339, 14.11371147303758278 ) ) ;
#9809=CARTESIAN_POINT ( 'NONE',  ( -35.74814306589956203, -115.9929510916434481, 13.05539834812772781 ) ) ;
#9810=CARTESIAN_POINT ( 'NONE',  ( -35.50000000000000711, -116.0140978167138712, -0.3122823525984417259 ) ) ;
#9820=CARTESIAN_POINT ( 'NONE',  ( -36.02454729103298092, -114.4734759653044307, 7.597274454178449155 ) ) ;
#9828=CARTESIAN_POINT ( 'NONE',  ( -34.00000000000000000, -113.9407375970686758, 6.996475545821551734 ) ) ;
#9845=CARTESIAN_POINT ( 'NONE',  ( -37.46874999999995737, -115.9929510916434481, 14.11852480586265024 ) ) ;
#9847=CARTESIAN_POINT ( 'NONE',  ( -38.99999999999999289, -113.9407375970686900, 5.253524454178449155 ) ) ;
#9849=CARTESIAN_POINT ( 'NONE',  ( -34.50000000000000000, -115.9929510916434481, 12.53051367006571581 ) ) ;
#9861=CARTESIAN_POINT ( 'NONE',  ( -34.83677480945821259, -116.0794154965774965, 7.183975545821551734 ) ) ;
#9863=CARTESIAN_POINT ( 'NONE',  ( -35.50000000000000000, -113.0140978167137717, 0.8752176474015607166 ) ) ;
#9880=CARTESIAN_POINT ( 'NONE',  ( -35.50000000000000000, -111.0140821919592327, -0.5779076015960634694 ) ) ;
#9887=CARTESIAN_POINT ( 'NONE',  ( -34.49999793727135255, -114.9929510916434339, 12.61164896875036590 ) ) ;
#9889=CARTESIAN_POINT ( 'NONE',  ( -37.50818044754229419, -114.9929510916434339, 13.11847460610629668 ) ) ;
#9891=CARTESIAN_POINT ( 'NONE',  ( -39.00000000000000000, -113.9929510916434339, 12.56351784598954779 ) ) ;
#9893=CARTESIAN_POINT ( 'NONE',  ( -37.75185693410092824, -114.9929510916434339, 13.05539834812634581 ) ) ;
#9902=CARTESIAN_POINT ( 'NONE',  ( -35.50000000000000711, -114.9929510916434339, 10.52826033068511435 ) ) ;
#9912=CARTESIAN_POINT ( 'NONE',  ( -34.50000000000000000, -113.2441867727860227, 0.9026824934337903672 ) ) ;
#9917=CARTESIAN_POINT ( 'NONE',  ( -38.18337828418795965, -110.9754527089670546, 4.034774454178449155 ) ) ;
#9921=CARTESIAN_POINT ( 'NONE',  ( -35.50000000000000711, -112.9486715495423681, -1.623175561345890472 ) ) ;
#9928=CARTESIAN_POINT ( 'NONE',  ( -34.50000000000000000, -113.6807644833805995, -1.624782352598427959 ) ) ;
#9936=CARTESIAN_POINT ( 'NONE',  ( -38.00000000000000711, -113.9929510916434339, 12.44250253426875119 ) ) ;
#9940=CARTESIAN_POINT ( 'NONE',  ( -35.50025087934803736, -113.9929510916434339, 12.63488142334835196 ) ) ;
#9941=CARTESIAN_POINT ( 'NONE',  ( -38.00000000000000711, -115.9929510916434481, 12.53051367006571937 ) ) ;
#9956=CARTESIAN_POINT ( 'NONE',  ( -35.50000000000000711, -112.1222502514821144, 1.343475657184566296 ) ) ;
#9959=B_SPLINE_CURVE_WITH_KNOTS ( 'NONE', 3,
 ( #33238, #28191, #27839, #8907, #25137, #6222, #14846, #1003, #14479, #6392, #17356, #19531, #11444, #19872, #30537, #17006, #28541, #11612, #3179, #3705, #14655, #28361, #22585, #5867, #25670, #33768, #14137, #17535, #11980, #464, #22947, #30887, #25490, #16832, #33405, #17182, #33946, #8727, #9097, #3530, #25312, #19696, #20228, #30711, #6042, #807, #11786, #20055, #31063, #9274, #28016, #633, #1181, #31238, #6560, #3891, #3363, #25853, #22243, #14309, #32129, #23853, #31766, #12154, #29260, #12328, #34303, #20766, #15725, #1527, #26741, #9633, #1351, #12695, #7456, #23490, #15019, #23672, #26377, #7101, #18074, #18438, #12512, #17722, #4606, #15543, #26562, #4780, #34123, #29436, #7281, #29073, #23125, #34660, #9984, #9443, #15365, #4423, #26192, #23300, #17899, #20594, #1898, #20946, #4247, #20401, #31945, #31590, #10166, #28722, #12874, #34841, #31415, #4075, #6747, #34484, #26023, #6926, #28895, #1709, #15184, #18257, #9804, #21136, #10843, #13884, #30100, #8820, #11366, #33328, #11183, #16746, #33495, #11015, #552, #5789, #14049, #14229, #2925, #24874, #26, #11539, #19272, #27409, #2758, #27590, #32977, #19103, #13720, #25046, #30462, #27756, #19462, #22155, #6136, #199, #17098, #21981 ),
 .UNSPECIFIED., .F., .F.,
 ( 4, 2, 2, 2, 2, 2, 2, 2, 2, 2, 2, 2, 2, 2, 2, 2, 2, 2, 2, 2, 2, 2, 2, 2, 2, 2, 2, 2, 2, 2, 2, 2, 2, 2, 2, 2, 2, 2, 2, 2, 2, 2, 2, 2, 2, 2, 2, 2, 2, 2, 2, 2, 2, 2, 2, 2, 2, 2, 2, 2, 2, 2, 2, 2, 2, 2, 2, 2, 2, 2, 2, 2, 2, 2, 2, 2, 2, 2, 4 ),
 ( 0.000000000000000000, 0.005381740036788157898, 0.008072610055182236413, 0.009418045064379276105, 0.01009076256897779508, 0.01076348007357631580, 0.01185104180586291078, 0.01293860353814950404, 0.01511372700272269054, 0.01946397393186906355, 0.02816446779016181304, 0.04556545550674730855, 0.08036743093991829956, 0.1151694063730892975, 0.1325703940896748034, 0.1412708879479675494, 0.1456211348771139225, 0.1477962583416871090, 0.1488838200739737161, 0.1499713818062602955, 0.1507624401091536004, 0.1515534984120469053, 0.1531356150178334874, 0.1562998482294066793, 0.1626283146525530909, 0.1752852474988458864, 0.2005991131914315051, 0.2512268445766027147, 0.3018545759617738966, 0.3271684416543594875, 0.3398253745006523108, 0.3461538409237986946, 0.3493180741353718588, 0.3509001907411584686, 0.3524823073469450785, 0.3548354025267266287, 0.3571884977065081790, 0.3618946880660712795, 0.3713070687851974805, 0.3901318302234498825, 0.4277813530999547420, 0.4654308759764596015, 0.4842556374147120035, 0.4936680181338382045, 0.4983742084934013050, 0.5007273036731828553, 0.5030803988529644055, 0.5053274392295320494, 0.5075744796060996933, 0.5120685603592350921, 0.5210567218655057786, 0.5390330448780472627, 0.5749856909031301200, 0.6109383369282129772, 0.6289146599407544613, 0.6379028214470251479, 0.6423969022001605467, 0.6446439425767281906, 0.6468909829532958344, 0.6492440781330773847, 0.6515971733128589349, 0.6563033636724220354, 0.6657157443915482364, 0.6845405058298006384, 0.7221900287063054424, 0.7598395515828102464, 0.7786643130210626484, 0.7880766937401888494, 0.7927828840997519499, 0.7951359792795336112, 0.7974890744593151615, 0.7990711910651018268, 0.8006533076708883812, 0.8038175408824614898, 0.8101460073056079292, 0.8228029401519008079, 0.8481168058444863433, 0.8987445372296576362, 1.000000000000000000 ),
 .UNSPECIFIED. ) ;
#9960=CARTESIAN_POINT ( 'NONE',  ( -35.50000000000000711, -114.1489256397697289, 9.518467544735724317 ) ) ;
#9965=CARTESIAN_POINT ( 'NONE',  ( -34.50000000000000000, -117.0140978167138854, -0.3122823525984416704 ) ) ;
#9969=CARTESIAN_POINT ( 'NONE',  ( -36.94073759706868287, -115.0000000000000000, 8.871475545821548181 ) ) ;
#9973=CARTESIAN_POINT ( 'NONE',  ( -34.50000000000000000, -113.1981689815712997, 0.8971895242272823756 ) ) ;
#9980=CARTESIAN_POINT ( 'NONE',  ( -35.50000000000000000, -113.9948283797722439, 10.50648163149984171 ) ) ;
#9984=CARTESIAN_POINT ( 'NONE',  ( -36.01562499999996447, -114.9929510916434339, 14.11852480586264846 ) ) ;
#9989=CARTESIAN_POINT ( 'NONE',  ( -35.50000000000000000, -115.9929510916434481, 12.53051367006571581 ) ) ;
#10001=CARTESIAN_POINT ( 'NONE',  ( -37.97545270896701908, -113.5265240346955977, 6.847274454178448266 ) ) ;
#10011=CARTESIAN_POINT ( 'NONE',  ( -36.94073759706868287, -116.9999999999999858, 8.871475545821548181 ) ) ;
#10031=CARTESIAN_POINT ( 'NONE',  ( -34.50000000000000000, -115.9929510916434481, 12.60752341388803721 ) ) ;
#10034=CARTESIAN_POINT ( 'NONE',  ( -35.02454729103298092, -114.8876895276775087, 6.097274454178449155 ) ) ;
#10035=CARTESIAN_POINT ( 'NONE',  ( -34.50000000000000000, -115.9929510916434481, 12.60752341388803721 ) ) ;
#10042=CARTESIAN_POINT ( 'NONE',  ( -36.11231047232249125, -115.9754527089670262, 2.777725545821550845 ) ) ;
#10044=CARTESIAN_POINT ( 'NONE',  ( -35.50000000000000000, -113.0140978167140702, 0.8752176474015603835 ) ) ;
#10061=CARTESIAN_POINT ( 'NONE',  ( -35.50000000000000000, -117.0140978167138854, 0.8752176474015623819 ) ) ;
#10070=CARTESIAN_POINT ( 'NONE',  ( -34.50000000000000000, -114.9929510916434339, 12.39849696637031506 ) ) ;
#10072=CARTESIAN_POINT ( 'NONE',  ( -35.52552712174884419, -114.9929510916434339, 12.77960891308624447 ) ) ;
#10075=CARTESIAN_POINT ( 'NONE',  ( -34.50000000000000000, -114.9929296450195721, 10.49869535309826674 ) ) ;
#10085=CARTESIAN_POINT ( 'NONE',  ( -36.31249999999995026, -114.9929510916434339, 13.11852480586264669 ) ) ;
#10087=CARTESIAN_POINT ( 'NONE',  ( -37.05926240293131713, -115.9999999999999858, 4.878524454178449155 ) ) ;
#10092=CARTESIAN_POINT ( 'NONE',  ( -34.50000000000000000, -113.0140978167138712, 0.7189676474015717078 ) ) ;
#10095=CARTESIAN_POINT ( 'NONE',  ( -39.99999999999999289, -113.9407375970686758, 3.753524454178448710 ) ) ;
#10105=CARTESIAN_POINT ( 'NONE',  ( -34.50000000000000000, -112.7530559548648341, -2.608751991713152307 ) ) ;
#10116=CARTESIAN_POINT ( 'NONE',  ( -38.00000000000000711, -113.9929510916434339, 11.73841344789285657 ) ) ;
#10119=CARTESIAN_POINT ( 'NONE',  ( -34.50000000000000000, -113.9186338266397058, 10.49738657667399266 ) ) ;
#10122=CARTESIAN_POINT ( 'NONE',  ( -35.99386409314529800, -115.9929510916434481, 13.11852378322482515 ) ) ;
#10133=CARTESIAN_POINT ( 'NONE',  ( -35.50000000000000711, -112.5103839485166333, -1.498529437127682495 ) ) ;
#10142=CARTESIAN_POINT ( 'NONE',  ( -35.50000000000000000, -111.0141141789186605, -0.6738694770610589302 ) ) ;
#10146=CARTESIAN_POINT ( 'NONE',  ( -39.02454729103295961, -114.7691647218148745, 2.159774454178448710 ) ) ;
#10153=CARTESIAN_POINT ( 'NONE',  ( -34.50000000000000000, -113.0140978167137860, 0.8752176474016654106 ) ) ;
#10161=CARTESIAN_POINT ( 'NONE',  ( -35.50000000000000000, -113.9743717753924699, 10.50403980422039396 ) ) ;
#10164=CARTESIAN_POINT ( 'NONE',  ( -34.50000000000000000, -112.0140978167138712, -0.1247823525984259746 ) ) ;
#10166=CARTESIAN_POINT ( 'NONE',  ( -37.24999999999992895, -114.9929510916434339, 14.11852480586264846 ) ) ;
#10172=CARTESIAN_POINT ( 'NONE',  ( -35.97955704204053262, -115.9929510916434481, 13.11812344617474402 ) ) ;
#10184=CARTESIAN_POINT ( 'NONE',  ( -37.35495115944176092, -112.9754527089670688, 7.034774454178450043 ) ) ;
#10189=ORIENTED_EDGE ( 'NONE', *, *, #23890, .F. ) ;
#10197=CARTESIAN_POINT ( 'NONE',  ( -37.76916472181486739, -116.0245472910329880, 5.965225545821550845 ) ) ;
#10221=CARTESIAN_POINT ( 'NONE',  ( -36.94073759706868287, -112.0000000000000142, 8.628524454178448266 ) ) ;
#10222=CARTESIAN_POINT ( 'NONE',  ( -34.50000000000000000, -114.7000328234681206, 8.631511418192262752 ) ) ;
#10233=CARTESIAN_POINT ( 'NONE',  ( -38.37230871539094323, -115.4561184093552413, 3.058975545821551290 ) ) ;
#10256=CARTESIAN_POINT ( 'NONE',  ( -35.50000000000000711, -112.0140978167138712, -0.4685323525984295134 ) ) ;
#10263=CARTESIAN_POINT ( 'NONE',  ( -34.50000000000000000, -112.0577668799241309, 1.173706424699810569 ) ) ;
#10264=CARTESIAN_POINT ( 'NONE',  ( -34.50000000000000000, -114.9929510916434339, 10.53376102667243508 ) ) ;
#10266=CARTESIAN_POINT ( 'NONE',  ( -37.89983305244309975, -114.9929510916434339, 12.92579853460519246 ) ) ;
#10268=CARTESIAN_POINT ( 'NONE',  ( -34.50000000000000000, -114.0185793162512908, 9.502217742515812304 ) ) ;
#10269=DIRECTION ( 'NONE',  ( -1.000000000000000000, 0.000000000000000000, 0.000000000000000000 ) ) ;
#10270=CARTESIAN_POINT ( 'NONE',  ( -37.99359134332094357, -114.9929510916434339, 12.69998175888958158 ) ) ;
#10271=FILL_AREA_STYLE ('',( #18707 ) ) ;
#10276=CARTESIAN_POINT ( 'NONE',  ( -37.58145695302688694, -114.9929510916434339, 13.11211614918362756 ) ) ;
#10279=CARTESIAN_POINT ( 'NONE',  ( -38.97545270896704039, -113.1123104723225197, 8.347274454178448266 ) ) ;
#10289=CARTESIAN_POINT ( 'NONE',  ( -34.83677480945819838, -111.9205845034225462, 2.816024454178448710 ) ) ;
#10298=ORIENTED_EDGE ( 'NONE', *, *, #2909, .T. ) ;
#10300=CARTESIAN_POINT ( 'NONE',  ( -34.50000000000000000, -113.6807644833805995, -2.624782352598442614 ) ) ;
#10303=CARTESIAN_POINT ( 'NONE',  ( -35.50000000000000711, -114.5636144531578680, 9.676196722963288366 ) ) ;
#10305=CARTESIAN_POINT ( 'NONE',  ( -34.50000000000000000, -113.9557924591415627, 10.50182206170499555 ) ) ;
#10306=( BOUNDED_SURFACE ( )  B_SPLINE_SURFACE ( 3, 3, ( 
 ( #30180, #30534, #10921, #8904, #16652, #108, #11096, #22238, #5693, #2835, #8372, #22406, #27836, #460, #3174, #13794, #33235, #6218, #19355, #19691, #33401, #8724, #17000, #8554, #3004, #14305, #3360, #13964, #19525, #30708, #6039, #5864, #17178, #28010, #3527, #25306, #629, #11608, #22581, #21890, #32881, #8205, #19185, #5517, #34117, #29071, #14842, #4419, #22941, #14652, #3701, #33940, #31588, #6743, #26019, #4070, #20397, #31409, #25485, #17896, #9092, #6922, #17719, #6388, #28891, #25849, #803, #4243, #1348, #17353, #20763, #15182, #15014, #20050, #9440, #1174, #11977, #3885, #12150, #23122, #11783, #9271, #28717, #25665, #20224, #26189, #1525, #998, #12324, #22760, #31233, #23297, #9800, #18071, #28356, #12508, #6556, #17531, #33762, #34297, #9627, #28536, #31763, #31058, #20592, #23487, #7095, #34481, #10516, #24040, #29612, #10695, #23849, #13398, #18613, #26921, #27090, #15720, #26736, #12870, #13231, #2430, #24382, #34836, #29965, #4776, #26374, #20942, #15539, #21661, #1706, #5133, #7987, #31942, #16071, #2076, #7623, #12691, #23670, #13053, #7804, #29258, #2264, #32302, #18432, #35197, #35027, #21477, #35370, #10344, #4948, #21303, #15900, #24204, #32125, #21132, #32471, #18791 ),
 ( #34657, #32665, #7453, #4603, #26560, #29795, #10161, #7278, #1896, #18968, #15362, #9980, #18253, #29431, #2962, #25266, #13756, #25084, #5475, #8158, #588, #16428, #19492, #11574, #27626, #19826, #2607, #3313, #27449, #21843, #30495, #11223, #13923, #22190, #33535, #22021, #5824, #22544, #33191, #8863, #14266, #32836, #8518, #30320, #33016, #5307, #16785, #27795, #65, #24912, #3132, #16245, #14088, #10880, #235, #19139, #412, #27264, #11403, #22367, #27962, #11052, #13572, #30136, #16614, #24563, #8330, #35557, #5657, #2796, #33362, #8687, #19654, #24738, #19309, #30665, #5997, #16957, #23453, #6702, #17683, #1484, #34076, #14803, #9226, #6346, #950, #6882, #31015, #9588, #31372, #22903, #28145, #4027, #17312, #28850, #11743, #20556, #34255, #3487, #22721, #25448, #20182, #30837, #20009, #14437, #25809, #766, #28318, #11932, #31190, #28495, #17494, #4204, #3664, #33712, #9401, #1134, #3843, #12107, #34448, #33897, #28682, #26149, #23078, #12467, #15145, #9050, #20358, #6521, #14971, #9765, #25977, #1303, #25625, #12287, #23257, #6176, #31557, #14613, #17853, #17139, #4742, #13360, #7418, #26697, #7761, #15503, #18031, #9936, #32088, #29028, #26522, #27051, #10116, #26338, #2223, #13192 ),
 ( #32266, #1673, #16032, #24165, #10305, #15323, #15679, #21083, #7234, #34792, #18395, #29397, #7054, #4569, #2031, #20899, #1854, #10479, #35159, #31898, #13007, #24343, #12827, #23993, #5089, #35333, #12655, #21441, #18215, #23631, #4378, #34985, #21267, #34617, #2392, #29221, #7586, #23810, #20725, #29575, #15854, #18574, #4909, #31721, #26876, #18744, #32438, #29748, #22328, #11008, #21973, #8115, #8478, #33321, #8647, #30096, #25225, #22, #21614, #16203, #10839, #5953, #32615, #365, #3266, #27226, #11362, #32973, #2921, #7944, #18923, #8288, #3091, #24521, #33148, #27584, #13715, #30456, #11179, #5434, #30276, #22150, #29924, #16576, #2568, #19267, #13534, #5614, #14225, #13880, #24866, #19614, #16385, #5266, #35510, #194, #21797, #27403, #16910, #19455, #32794, #27750, #14044, #25041, #10656, #19096, #27916, #5785, #16742, #2754, #30617, #24694, #6834, #3794, #20142, #14566, #11700, #6302, #12244, #717, #14924, #1088, #28276, #33489, #9358, #22669, #34211, #17094, #25936, #3981, #8816, #28101, #30789, #25580, #547, #25403, #19778, #31148, #6130, #33660, #17271, #897, #33851, #22856, #20505, #11879, #17450, #9178, #6478, #23035, #3618, #28450, #20319, #14751, #30969, #19962, #28635, #3445 ),
 ( #8996, #25761, #12059, #14397, #34033, #31325, #6653, #17631, #1259, #23218, #9538, #31513, #17805, #28807, #4156, #15097, #11533, #22501, #4699, #32396, #12781, #5045, #23401, #24126, #12604, #7008, #15631, #32043, #34748, #7379, #18699, #7187, #26652, #21399, #18351, #7716, #35117, #17983, #29351, #15455, #18166, #10441, #1983, #34572, #10264, #26289, #28983, #29697, #1625, #12959, #26108, #23760, #1438, #34400, #12417, #23579, #4331, #23944, #34940, #10070, #21225, #9718, #29175, #32221, #20677, #7547, #31675, #15275, #9887, #18527, #26472, #4526, #20851, #29530, #4864, #31854, #21035, #15807, #1807, #26826, #2181, #13151, #18883, #16655, #8599, #2703, #21933, #3047, #10793, #13321, #5225, #27355, #24301, #21752, #22287, #5394, #21568, #33106, #8428, #19413, #19571, #2351, #11317, #11142, #32928, #30576, #27541, #2877, #33282, #19225, #10967, #30055, #27183, #32746, #27710, #16165, #30412, #16531, #8073, #35291, #24827, #2525, #14007, #32564, #5740, #16698, #10611, #7899, #29879, #16341, #15991, #13491, #24474, #8249, #35461, #19056, #13671, #24651, #30230, #5567, #325, #13839, #151, #22110, #25000, #27005, #22627, #11657, #14706, #6264, #675, #25361, #33995, #510, #852, #16873, #14888, #33620 ),
 ( #11487, #6087, #1225, #27877, #31284, #34172, #22458, #6611, #17228, #30932, #11834, #33450, #12204, #14185, #28234, #8772, #23177, #25719, #1052, #14521, #20102, #9495, #14354, #3942, #9140, #17405, #17583, #3574, #25539, #3407, #3751, #28590, #25898, #8953, #20455, #22814, #3223, #19739, #17053, #5909, #25188, #30752, #28066, #19917, #33815, #31109, #6436, #28408, #12023, #22993, #9321, #20277, #18308, #12740, #34529, #15586, #31813, #26608, #34708, #7334, #12917, #18123, #15233, #10699, #34896, #1580, #17943, #10031, #23716, #12375, #29974, #4292, #5311, #20995, #31633, #12562, #7992, #15415, #31467, #23903, #6969, #28944, #4476, #35562, #20810, #10885, #26242, #20634, #9679, #23535, #1943, #31998, #29306, #4656, #26428, #1758, #6794, #21667, #15060, #32671, #18974, #23352, #16251, #7148, #17765, #27269, #2611, #34351, #13576, #24568, #28767, #26070, #4119, #29127, #9845, #1399, #33197, #242, #8164, #5661, #11227, #22027, #16619, #11580, #593, #33021, #19496, #25452, #27631, #3139, #6184, #14443, #2801, #22548, #11058, #13760, #19144, #30142, #19832, #8335, #24744, #419, #27802, #30499, #14094, #770, #2970, #22371, #17144, #25088, #28149, #30843, #71, #11408, #22195, #13928, #3491, #33367 ),
 ( #8693, #27453, #8523, #19313, #5831, #21849, #16790, #19658, #8869, #24918, #5479, #30325, #30671, #16432, #6004, #32845, #16963, #27968, #3319, #14272, #25270, #33539, #33718, #7059, #6886, #28686, #4381, #23262, #34258, #18036, #14976, #31375, #25814, #22909, #17500, #23456, #11939, #26154, #12290, #3847, #9057, #20560, #33903, #9768, #28322, #1487, #15148, #20015, #3668, #6351, #1140, #11749, #955, #31019, #6705, #17317, #9231, #28499, #12114, #9405, #34080, #31728, #23084, #4032, #20364, #17687, #9591, #14809, #25984, #31560, #1306, #6524, #31194, #4209, #14619, #17859, #22726, #20730, #28856, #20189, #12471, #34451, #29033, #25629, #15326, #26342, #29579, #26882, #18578, #29226, #34990, #21618, #10122, #21445, #1860, #4572, #32620, #12832, #15860, #7949, #23999, #16209, #13196, #18750, #10311, #21087, #16037, #5097, #7422, #23814, #2229, #4916, #18218, #35337, #32093, #10662, #24169, #34799, #18399, #13365, #21271, #1676, #29752, #29401, #4746, #32270, #5270, #26702, #12658, #15683, #26526, #15506, #2038, #7767, #35163, #10484, #32442, #7591, #27055, #23635, #2397, #20904, #24347, #18930, #13014, #29929, #34622, #9941, #31904, #7237, #8122, #22506, #30625, #16748, #21804, #11184, #16582, #13722 ),
 ( #27592, #27410, #11016, #16917, #5958, #2759, #24875, #30798, #32978, #8483, #11540, #19783, #19104, #27925, #16392, #30101, #24526, #2927, #33154, #5439, #33496, #35514, #13885, #24702, #8822, #371, #22334, #200, #5791, #6138, #27, #25231, #30463, #3097, #3273, #22157, #19464, #21982, #25048, #14230, #553, #8293, #27230, #27757, #2572, #32801, #19274, #13539, #10845, #30282, #5621, #14050, #11367, #33329, #8652, #19619, #25410, #28456, #9547, #30976, #3987, #6310, #20324, #14402, #15105, #3626, #22862, #28813, #17276, #31518, #17638, #9186, #725, #25942, #28281, #26114, #33668, #6841, #20514, #11705, #9004, #22675, #6484, #17099, #14572, #19968, #12067, #25585, #906, #33859, #17457, #14758, #3801, #1444, #25766, #34038, #1095, #23040, #14932, #20147, #31153, #1264, #9365, #11885, #31332, #17813, #6660, #28641, #28108, #12426, #12250, #23223, #34216, #4163, #23410, #34407, #9724, #20686, #31681, #3451, #23954, #34579, #4706, #27012, #15464, #26834, #7193, #9893, #2358, #18173, #7015, #4532, #31861, #10270, #4337, #5053, #29184, #23587, #21233, #12966, #15637, #34949, #35300, #23767, #7555, #13328, #32229, #24308, #15998, #20859, #18534, #32050, #34755, #10618, #29538, #4871, #1813, #26660 ) ),
 .UNSPECIFIED., .T., .F., .T. ) 
 B_SPLINE_SURFACE_WITH_KNOTS ( ( 4, 3, 4 ),
 ( 4, 2, 2, 2, 2, 2, 2, 2, 2, 2, 2, 2, 2, 2, 2, 2, 2, 2, 2, 2, 2, 2, 2, 2, 2, 2, 2, 2, 2, 2, 2, 2, 2, 2, 2, 2, 2, 2, 2, 2, 2, 2, 2, 2, 2, 2, 2, 2, 2, 2, 2, 2, 2, 2, 2, 2, 2, 2, 2, 2, 2, 2, 2, 2, 2, 2, 2, 2, 2, 2, 2, 2, 2, 2, 2, 2, 2, 2, 4 ),
 ( 0.000000000000000000, 0.5000000000000000000, 1.000000000000000000 ),
 ( 0.000000000000000000, 0.005381740036788157898, 0.008072610055182236413, 0.009418045064379276105, 0.01009076256897779508, 0.01076348007357631580, 0.01185104180586291078, 0.01293860353814950404, 0.01511372700272269054, 0.01946397393186906355, 0.02816446779016181304, 0.04556545550674730855, 0.08036743093991829956, 0.1151694063730892975, 0.1325703940896748034, 0.1412708879479675494, 0.1456211348771139225, 0.1477962583416871090, 0.1488838200739737161, 0.1499713818062602955, 0.1507624401091536004, 0.1515534984120469053, 0.1531356150178334874, 0.1562998482294066793, 0.1626283146525530909, 0.1752852474988458864, 0.2005991131914315051, 0.2512268445766027147, 0.3018545759617738966, 0.3271684416543594875, 0.3398253745006523108, 0.3461538409237986946, 0.3493180741353718588, 0.3509001907411584686, 0.3524823073469450785, 0.3548354025267266287, 0.3571884977065081790, 0.3618946880660712795, 0.3713070687851974805, 0.3901318302234498825, 0.4277813530999547420, 0.4654308759764596015, 0.4842556374147120035, 0.4936680181338382045, 0.4983742084934013050, 0.5007273036731828553, 0.5030803988529644055, 0.5053274392295320494, 0.5075744796060996933, 0.5120685603592350921, 0.5210567218655057786, 0.5390330448780472627, 0.5749856909031301200, 0.6109383369282129772, 0.6289146599407544613, 0.6379028214470251479, 0.6423969022001605467, 0.6446439425767281906, 0.6468909829532958344, 0.6492440781330773847, 0.6515971733128589349, 0.6563033636724220354, 0.6657157443915482364, 0.6845405058298006384, 0.7221900287063054424, 0.7598395515828102464, 0.7786643130210626484, 0.7880766937401888494, 0.7927828840997519499, 0.7951359792795336112, 0.7974890744593151615, 0.7990711910651018268, 0.8006533076708883812, 0.8038175408824614898, 0.8101460073056079292, 0.8228029401519008079, 0.8481168058444863433, 0.8987445372296576362, 1.000000000000000000 ),
 .UNSPECIFIED. ) 
 GEOMETRIC_REPRESENTATION_ITEM ( )  RATIONAL_B_SPLINE_SURFACE ( (
 ( 1.000000000000000000, 1.000000000000000000, 1.000000000000000000, 1.000000000000000000, 1.000000000000000000, 1.000000000000000000, 1.000000000000000000, 1.000000000000000000, 1.000000000000000000, 1.000000000000000000, 1.000000000000000000, 1.000000000000000000, 1.000000000000000000, 1.000000000000000000, 1.000000000000000000, 1.000000000000000000, 1.000000000000000000, 1.000000000000000000, 1.000000000000000000, 1.000000000000000000, 1.000000000000000000, 1.000000000000000000, 1.000000000000000000, 1.000000000000000000, 1.000000000000000000, 1.000000000000000000, 1.000000000000000000, 1.000000000000000000, 1.000000000000000000, 1.000000000000000000, 1.000000000000000000, 1.000000000000000000, 1.000000000000000000, 1.000000000000000000, 1.000000000000000000, 1.000000000000000000, 1.000000000000000000, 1.000000000000000000, 1.000000000000000000, 1.000000000000000000, 1.000000000000000000, 1.000000000000000000, 1.000000000000000000, 1.000000000000000000, 1.000000000000000000, 1.000000000000000000, 1.000000000000000000, 1.000000000000000000, 1.000000000000000000, 1.000000000000000000, 1.000000000000000000, 1.000000000000000000, 1.000000000000000000, 1.000000000000000000, 1.000000000000000000, 1.000000000000000000, 1.000000000000000000, 1.000000000000000000, 1.000000000000000000, 1.000000000000000000, 1.000000000000000000, 1.000000000000000000, 1.000000000000000000, 1.000000000000000000, 1.000000000000000000, 1.000000000000000000, 1.000000000000000000, 1.000000000000000000, 1.000000000000000000, 1.000000000000000000, 1.000000000000000000, 1.000000000000000000, 1.000000000000000000, 1.000000000000000000, 1.000000000000000000, 1.000000000000000000, 1.000000000000000000, 1.000000000000000000, 1.000000000000000000, 1.000000000000000000, 1.000000000000000000, 1.000000000000000000, 1.000000000000000000, 1.000000000000000000, 1.000000000000000000, 1.000000000000000000, 1.000000000000000000, 1.000000000000000000, 1.000000000000000000, 1.000000000000000000, 1.000000000000000000, 1.000000000000000000, 1.000000000000000000, 1.000000000000000000, 1.000000000000000000, 1.000000000000000000, 1.000000000000000000, 1.000000000000000000, 1.000000000000000000, 1.000000000000000000, 1.000000000000000000, 1.000000000000000000, 1.000000000000000000, 1.000000000000000000, 1.000000000000000000, 1.000000000000000000, 1.000000000000000000, 1.000000000000000000, 1.000000000000000000, 1.000000000000000000, 1.000000000000000000, 1.000000000000000000, 1.000000000000000000, 1.000000000000000000, 1.000000000000000000, 1.000000000000000000, 1.000000000000000000, 1.000000000000000000, 1.000000000000000000, 1.000000000000000000, 1.000000000000000000, 1.000000000000000000, 1.000000000000000000, 1.000000000000000000, 1.000000000000000000, 1.000000000000000000, 1.000000000000000000, 1.000000000000000000, 1.000000000000000000, 1.000000000000000000, 1.000000000000000000, 1.000000000000000000, 1.000000000000000000, 1.000000000000000000, 1.000000000000000000, 1.000000000000000000, 1.000000000000000000, 1.000000000000000000, 1.000000000000000000, 1.000000000000000000, 1.000000000000000000, 1.000000000000000000, 1.000000000000000000, 1.000000000000000000, 1.000000000000000000, 1.000000000000000000, 1.000000000000000000, 1.000000000000000000, 1.000000000000000000, 1.000000000000000000, 1.000000000000000000, 1.000000000000000000, 1.000000000000000000, 1.000000000000000000, 1.000000000000000000, 1.000000000000000000, 1.000000000000000000, 1.000000000000000000),
 ( 0.3333333333333333703, 0.3333333333333333703, 0.3333333333333333703, 0.3333333333333333703, 0.3333333333333333703, 0.3333333333333333703, 0.3333333333333333703, 0.3333333333333333703, 0.3333333333333333703, 0.3333333333333333703, 0.3333333333333333703, 0.3333333333333333703, 0.3333333333333333703, 0.3333333333333333703, 0.3333333333333333703, 0.3333333333333333703, 0.3333333333333333703, 0.3333333333333333703, 0.3333333333333333703, 0.3333333333333333703, 0.3333333333333333703, 0.3333333333333333703, 0.3333333333333333703, 0.3333333333333333703, 0.3333333333333333703, 0.3333333333333333703, 0.3333333333333333703, 0.3333333333333333703, 0.3333333333333333703, 0.3333333333333333703, 0.3333333333333333703, 0.3333333333333333703, 0.3333333333333333703, 0.3333333333333333703, 0.3333333333333333703, 0.3333333333333333703, 0.3333333333333333703, 0.3333333333333333703, 0.3333333333333333703, 0.3333333333333333703, 0.3333333333333333703, 0.3333333333333333703, 0.3333333333333333703, 0.3333333333333333703, 0.3333333333333333703, 0.3333333333333333703, 0.3333333333333333703, 0.3333333333333333703, 0.3333333333333333703, 0.3333333333333333703, 0.3333333333333333703, 0.3333333333333333703, 0.3333333333333333703, 0.3333333333333333703, 0.3333333333333333703, 0.3333333333333333703, 0.3333333333333333703, 0.3333333333333333703, 0.3333333333333333703, 0.3333333333333333703, 0.3333333333333333703, 0.3333333333333333703, 0.3333333333333333703, 0.3333333333333333703, 0.3333333333333333703, 0.3333333333333333703, 0.3333333333333333703, 0.3333333333333333703, 0.3333333333333333703, 0.3333333333333333703, 0.3333333333333333703, 0.3333333333333333703, 0.3333333333333333703, 0.3333333333333333703, 0.3333333333333333703, 0.3333333333333333703, 0.3333333333333333703, 0.3333333333333333703, 0.3333333333333333703, 0.3333333333333333703, 0.3333333333333333703, 0.3333333333333333703, 0.3333333333333333703, 0.3333333333333333703, 0.3333333333333333703, 0.3333333333333333703, 0.3333333333333333703, 0.3333333333333333703, 0.3333333333333333703, 0.3333333333333333703, 0.3333333333333333703, 0.3333333333333333703, 0.3333333333333333703, 0.3333333333333333703, 0.3333333333333333703, 0.3333333333333333703, 0.3333333333333333703, 0.3333333333333333703, 0.3333333333333333703, 0.3333333333333333703, 0.3333333333333333703, 0.3333333333333333703, 0.3333333333333333703, 0.3333333333333333703, 0.3333333333333333703, 0.3333333333333333703, 0.3333333333333333703, 0.3333333333333333703, 0.3333333333333333703, 0.3333333333333333703, 0.3333333333333333703, 0.3333333333333333703, 0.3333333333333333703, 0.3333333333333333703, 0.3333333333333333703, 0.3333333333333333703, 0.3333333333333333703, 0.3333333333333333703, 0.3333333333333333703, 0.3333333333333333703, 0.3333333333333333703, 0.3333333333333333703, 0.3333333333333333703, 0.3333333333333333703, 0.3333333333333333703, 0.3333333333333333703, 0.3333333333333333703, 0.3333333333333333703, 0.3333333333333333703, 0.3333333333333333703, 0.3333333333333333703, 0.3333333333333333703, 0.3333333333333333703, 0.3333333333333333703, 0.3333333333333333703, 0.3333333333333333703, 0.3333333333333333703, 0.3333333333333333703, 0.3333333333333333703, 0.3333333333333333703, 0.3333333333333333703, 0.3333333333333333703, 0.3333333333333333703, 0.3333333333333333703, 0.3333333333333333703, 0.3333333333333333703, 0.3333333333333333703, 0.3333333333333333703, 0.3333333333333333703, 0.3333333333333333703, 0.3333333333333333703, 0.3333333333333333703, 0.3333333333333333703, 0.3333333333333333703, 0.3333333333333333703, 0.3333333333333333703, 0.3333333333333333703, 0.3333333333333333703),
 ( 0.3333333333333333703, 0.3333333333333333703, 0.3333333333333333703, 0.3333333333333333703, 0.3333333333333333703, 0.3333333333333333703, 0.3333333333333333703, 0.3333333333333333703, 0.3333333333333333703, 0.3333333333333333703, 0.3333333333333333703, 0.3333333333333333703, 0.3333333333333333703, 0.3333333333333333703, 0.3333333333333333703, 0.3333333333333333703, 0.3333333333333333703, 0.3333333333333333703, 0.3333333333333333703, 0.3333333333333333703, 0.3333333333333333703, 0.3333333333333333703, 0.3333333333333333703, 0.3333333333333333703, 0.3333333333333333703, 0.3333333333333333703, 0.3333333333333333703, 0.3333333333333333703, 0.3333333333333333703, 0.3333333333333333703, 0.3333333333333333703, 0.3333333333333333703, 0.3333333333333333703, 0.3333333333333333703, 0.3333333333333333703, 0.3333333333333333703, 0.3333333333333333703, 0.3333333333333333703, 0.3333333333333333703, 0.3333333333333333703, 0.3333333333333333703, 0.3333333333333333703, 0.3333333333333333703, 0.3333333333333333703, 0.3333333333333333703, 0.3333333333333333703, 0.3333333333333333703, 0.3333333333333333703, 0.3333333333333333703, 0.3333333333333333703, 0.3333333333333333703, 0.3333333333333333703, 0.3333333333333333703, 0.3333333333333333703, 0.3333333333333333703, 0.3333333333333333703, 0.3333333333333333703, 0.3333333333333333703, 0.3333333333333333703, 0.3333333333333333703, 0.3333333333333333703, 0.3333333333333333703, 0.3333333333333333703, 0.3333333333333333703, 0.3333333333333333703, 0.3333333333333333703, 0.3333333333333333703, 0.3333333333333333703, 0.3333333333333333703, 0.3333333333333333703, 0.3333333333333333703, 0.3333333333333333703, 0.3333333333333333703, 0.3333333333333333703, 0.3333333333333333703, 0.3333333333333333703, 0.3333333333333333703, 0.3333333333333333703, 0.3333333333333333703, 0.3333333333333333703, 0.3333333333333333703, 0.3333333333333333703, 0.3333333333333333703, 0.3333333333333333703, 0.3333333333333333703, 0.3333333333333333703, 0.3333333333333333703, 0.3333333333333333703, 0.3333333333333333703, 0.3333333333333333703, 0.3333333333333333703, 0.3333333333333333703, 0.3333333333333333703, 0.3333333333333333703, 0.3333333333333333703, 0.3333333333333333703, 0.3333333333333333703, 0.3333333333333333703, 0.3333333333333333703, 0.3333333333333333703, 0.3333333333333333703, 0.3333333333333333703, 0.3333333333333333703, 0.3333333333333333703, 0.3333333333333333703, 0.3333333333333333703, 0.3333333333333333703, 0.3333333333333333703, 0.3333333333333333703, 0.3333333333333333703, 0.3333333333333333703, 0.3333333333333333703, 0.3333333333333333703, 0.3333333333333333703, 0.3333333333333333703, 0.3333333333333333703, 0.3333333333333333703, 0.3333333333333333703, 0.3333333333333333703, 0.3333333333333333703, 0.3333333333333333703, 0.3333333333333333703, 0.3333333333333333703, 0.3333333333333333703, 0.3333333333333333703, 0.3333333333333333703, 0.3333333333333333703, 0.3333333333333333703, 0.3333333333333333703, 0.3333333333333333703, 0.3333333333333333703, 0.3333333333333333703, 0.3333333333333333703, 0.3333333333333333703, 0.3333333333333333703, 0.3333333333333333703, 0.3333333333333333703, 0.3333333333333333703, 0.3333333333333333703, 0.3333333333333333703, 0.3333333333333333703, 0.3333333333333333703, 0.3333333333333333703, 0.3333333333333333703, 0.3333333333333333703, 0.3333333333333333703, 0.3333333333333333703, 0.3333333333333333703, 0.3333333333333333703, 0.3333333333333333703, 0.3333333333333333703, 0.3333333333333333703, 0.3333333333333333703, 0.3333333333333333703, 0.3333333333333333703, 0.3333333333333333703, 0.3333333333333333703, 0.3333333333333333703),
 ( 1.000000000000000000, 1.000000000000000000, 1.000000000000000000, 1.000000000000000000, 1.000000000000000000, 1.000000000000000000, 1.000000000000000000, 1.000000000000000000, 1.000000000000000000, 1.000000000000000000, 1.000000000000000000, 1.000000000000000000, 1.000000000000000000, 1.000000000000000000, 1.000000000000000000, 1.000000000000000000, 1.000000000000000000, 1.000000000000000000, 1.000000000000000000, 1.000000000000000000, 1.000000000000000000, 1.000000000000000000, 1.000000000000000000, 1.000000000000000000, 1.000000000000000000, 1.000000000000000000, 1.000000000000000000, 1.000000000000000000, 1.000000000000000000, 1.000000000000000000, 1.000000000000000000, 1.000000000000000000, 1.000000000000000000, 1.000000000000000000, 1.000000000000000000, 1.000000000000000000, 1.000000000000000000, 1.000000000000000000, 1.000000000000000000, 1.000000000000000000, 1.000000000000000000, 1.000000000000000000, 1.000000000000000000, 1.000000000000000000, 1.000000000000000000, 1.000000000000000000, 1.000000000000000000, 1.000000000000000000, 1.000000000000000000, 1.000000000000000000, 1.000000000000000000, 1.000000000000000000, 1.000000000000000000, 1.000000000000000000, 1.000000000000000000, 1.000000000000000000, 1.000000000000000000, 1.000000000000000000, 1.000000000000000000, 1.000000000000000000, 1.000000000000000000, 1.000000000000000000, 1.000000000000000000, 1.000000000000000000, 1.000000000000000000, 1.000000000000000000, 1.000000000000000000, 1.000000000000000000, 1.000000000000000000, 1.000000000000000000, 1.000000000000000000, 1.000000000000000000, 1.000000000000000000, 1.000000000000000000, 1.000000000000000000, 1.000000000000000000, 1.000000000000000000, 1.000000000000000000, 1.000000000000000000, 1.000000000000000000, 1.000000000000000000, 1.000000000000000000, 1.000000000000000000, 1.000000000000000000, 1.000000000000000000, 1.000000000000000000, 1.000000000000000000, 1.000000000000000000, 1.000000000000000000, 1.000000000000000000, 1.000000000000000000, 1.000000000000000000, 1.000000000000000000, 1.000000000000000000, 1.000000000000000000, 1.000000000000000000, 1.000000000000000000, 1.000000000000000000, 1.000000000000000000, 1.000000000000000000, 1.000000000000000000, 1.000000000000000000, 1.000000000000000000, 1.000000000000000000, 1.000000000000000000, 1.000000000000000000, 1.000000000000000000, 1.000000000000000000, 1.000000000000000000, 1.000000000000000000, 1.000000000000000000, 1.000000000000000000, 1.000000000000000000, 1.000000000000000000, 1.000000000000000000, 1.000000000000000000, 1.000000000000000000, 1.000000000000000000, 1.000000000000000000, 1.000000000000000000, 1.000000000000000000, 1.000000000000000000, 1.000000000000000000, 1.000000000000000000, 1.000000000000000000, 1.000000000000000000, 1.000000000000000000, 1.000000000000000000, 1.000000000000000000, 1.000000000000000000, 1.000000000000000000, 1.000000000000000000, 1.000000000000000000, 1.000000000000000000, 1.000000000000000000, 1.000000000000000000, 1.000000000000000000, 1.000000000000000000, 1.000000000000000000, 1.000000000000000000, 1.000000000000000000, 1.000000000000000000, 1.000000000000000000, 1.000000000000000000, 1.000000000000000000, 1.000000000000000000, 1.000000000000000000, 1.000000000000000000, 1.000000000000000000, 1.000000000000000000, 1.000000000000000000, 1.000000000000000000, 1.000000000000000000, 1.000000000000000000, 1.000000000000000000, 1.000000000000000000, 1.000000000000000000, 1.000000000000000000),
 ( 0.3333333333333333703, 0.3333333333333333703, 0.3333333333333333703, 0.3333333333333333703, 0.3333333333333333703, 0.3333333333333333703, 0.3333333333333333703, 0.3333333333333333703, 0.3333333333333333703, 0.3333333333333333703, 0.3333333333333333703, 0.3333333333333333703, 0.3333333333333333703, 0.3333333333333333703, 0.3333333333333333703, 0.3333333333333333703, 0.3333333333333333703, 0.3333333333333333703, 0.3333333333333333703, 0.3333333333333333703, 0.3333333333333333703, 0.3333333333333333703, 0.3333333333333333703, 0.3333333333333333703, 0.3333333333333333703, 0.3333333333333333703, 0.3333333333333333703, 0.3333333333333333703, 0.3333333333333333703, 0.3333333333333333703, 0.3333333333333333703, 0.3333333333333333703, 0.3333333333333333703, 0.3333333333333333703, 0.3333333333333333703, 0.3333333333333333703, 0.3333333333333333703, 0.3333333333333333703, 0.3333333333333333703, 0.3333333333333333703, 0.3333333333333333703, 0.3333333333333333703, 0.3333333333333333703, 0.3333333333333333703, 0.3333333333333333703, 0.3333333333333333703, 0.3333333333333333703, 0.3333333333333333703, 0.3333333333333333703, 0.3333333333333333703, 0.3333333333333333703, 0.3333333333333333703, 0.3333333333333333703, 0.3333333333333333703, 0.3333333333333333703, 0.3333333333333333703, 0.3333333333333333703, 0.3333333333333333703, 0.3333333333333333703, 0.3333333333333333703, 0.3333333333333333703, 0.3333333333333333703, 0.3333333333333333703, 0.3333333333333333703, 0.3333333333333333703, 0.3333333333333333703, 0.3333333333333333703, 0.3333333333333333703, 0.3333333333333333703, 0.3333333333333333703, 0.3333333333333333703, 0.3333333333333333703, 0.3333333333333333703, 0.3333333333333333703, 0.3333333333333333703, 0.3333333333333333703, 0.3333333333333333703, 0.3333333333333333703, 0.3333333333333333703, 0.3333333333333333703, 0.3333333333333333703, 0.3333333333333333703, 0.3333333333333333703, 0.3333333333333333703, 0.3333333333333333703, 0.3333333333333333703, 0.3333333333333333703, 0.3333333333333333703, 0.3333333333333333703, 0.3333333333333333703, 0.3333333333333333703, 0.3333333333333333703, 0.3333333333333333703, 0.3333333333333333703, 0.3333333333333333703, 0.3333333333333333703, 0.3333333333333333703, 0.3333333333333333703, 0.3333333333333333703, 0.3333333333333333703, 0.3333333333333333703, 0.3333333333333333703, 0.3333333333333333703, 0.3333333333333333703, 0.3333333333333333703, 0.3333333333333333703, 0.3333333333333333703, 0.3333333333333333703, 0.3333333333333333703, 0.3333333333333333703, 0.3333333333333333703, 0.3333333333333333703, 0.3333333333333333703, 0.3333333333333333703, 0.3333333333333333703, 0.3333333333333333703, 0.3333333333333333703, 0.3333333333333333703, 0.3333333333333333703, 0.3333333333333333703, 0.3333333333333333703, 0.3333333333333333703, 0.3333333333333333703, 0.3333333333333333703, 0.3333333333333333703, 0.3333333333333333703, 0.3333333333333333703, 0.3333333333333333703, 0.3333333333333333703, 0.3333333333333333703, 0.3333333333333333703, 0.3333333333333333703, 0.3333333333333333703, 0.3333333333333333703, 0.3333333333333333703, 0.3333333333333333703, 0.3333333333333333703, 0.3333333333333333703, 0.3333333333333333703, 0.3333333333333333703, 0.3333333333333333703, 0.3333333333333333703, 0.3333333333333333703, 0.3333333333333333703, 0.3333333333333333703, 0.3333333333333333703, 0.3333333333333333703, 0.3333333333333333703, 0.3333333333333333703, 0.3333333333333333703, 0.3333333333333333703, 0.3333333333333333703, 0.3333333333333333703, 0.3333333333333333703, 0.3333333333333333703, 0.3333333333333333703, 0.3333333333333333703, 0.3333333333333333703),
 ( 0.3333333333333333703, 0.3333333333333333703, 0.3333333333333333703, 0.3333333333333333703, 0.3333333333333333703, 0.3333333333333333703, 0.3333333333333333703, 0.3333333333333333703, 0.3333333333333333703, 0.3333333333333333703, 0.3333333333333333703, 0.3333333333333333703, 0.3333333333333333703, 0.3333333333333333703, 0.3333333333333333703, 0.3333333333333333703, 0.3333333333333333703, 0.3333333333333333703, 0.3333333333333333703, 0.3333333333333333703, 0.3333333333333333703, 0.3333333333333333703, 0.3333333333333333703, 0.3333333333333333703, 0.3333333333333333703, 0.3333333333333333703, 0.3333333333333333703, 0.3333333333333333703, 0.3333333333333333703, 0.3333333333333333703, 0.3333333333333333703, 0.3333333333333333703, 0.3333333333333333703, 0.3333333333333333703, 0.3333333333333333703, 0.3333333333333333703, 0.3333333333333333703, 0.3333333333333333703, 0.3333333333333333703, 0.3333333333333333703, 0.3333333333333333703, 0.3333333333333333703, 0.3333333333333333703, 0.3333333333333333703, 0.3333333333333333703, 0.3333333333333333703, 0.3333333333333333703, 0.3333333333333333703, 0.3333333333333333703, 0.3333333333333333703, 0.3333333333333333703, 0.3333333333333333703, 0.3333333333333333703, 0.3333333333333333703, 0.3333333333333333703, 0.3333333333333333703, 0.3333333333333333703, 0.3333333333333333703, 0.3333333333333333703, 0.3333333333333333703, 0.3333333333333333703, 0.3333333333333333703, 0.3333333333333333703, 0.3333333333333333703, 0.3333333333333333703, 0.3333333333333333703, 0.3333333333333333703, 0.3333333333333333703, 0.3333333333333333703, 0.3333333333333333703, 0.3333333333333333703, 0.3333333333333333703, 0.3333333333333333703, 0.3333333333333333703, 0.3333333333333333703, 0.3333333333333333703, 0.3333333333333333703, 0.3333333333333333703, 0.3333333333333333703, 0.3333333333333333703, 0.3333333333333333703, 0.3333333333333333703, 0.3333333333333333703, 0.3333333333333333703, 0.3333333333333333703, 0.3333333333333333703, 0.3333333333333333703, 0.3333333333333333703, 0.3333333333333333703, 0.3333333333333333703, 0.3333333333333333703, 0.3333333333333333703, 0.3333333333333333703, 0.3333333333333333703, 0.3333333333333333703, 0.3333333333333333703, 0.3333333333333333703, 0.3333333333333333703, 0.3333333333333333703, 0.3333333333333333703, 0.3333333333333333703, 0.3333333333333333703, 0.3333333333333333703, 0.3333333333333333703, 0.3333333333333333703, 0.3333333333333333703, 0.3333333333333333703, 0.3333333333333333703, 0.3333333333333333703, 0.3333333333333333703, 0.3333333333333333703, 0.3333333333333333703, 0.3333333333333333703, 0.3333333333333333703, 0.3333333333333333703, 0.3333333333333333703, 0.3333333333333333703, 0.3333333333333333703, 0.3333333333333333703, 0.3333333333333333703, 0.3333333333333333703, 0.3333333333333333703, 0.3333333333333333703, 0.3333333333333333703, 0.3333333333333333703, 0.3333333333333333703, 0.3333333333333333703, 0.3333333333333333703, 0.3333333333333333703, 0.3333333333333333703, 0.3333333333333333703, 0.3333333333333333703, 0.3333333333333333703, 0.3333333333333333703, 0.3333333333333333703, 0.3333333333333333703, 0.3333333333333333703, 0.3333333333333333703, 0.3333333333333333703, 0.3333333333333333703, 0.3333333333333333703, 0.3333333333333333703, 0.3333333333333333703, 0.3333333333333333703, 0.3333333333333333703, 0.3333333333333333703, 0.3333333333333333703, 0.3333333333333333703, 0.3333333333333333703, 0.3333333333333333703, 0.3333333333333333703, 0.3333333333333333703, 0.3333333333333333703, 0.3333333333333333703, 0.3333333333333333703, 0.3333333333333333703, 0.3333333333333333703, 0.3333333333333333703),
 ( 1.000000000000000000, 1.000000000000000000, 1.000000000000000000, 1.000000000000000000, 1.000000000000000000, 1.000000000000000000, 1.000000000000000000, 1.000000000000000000, 1.000000000000000000, 1.000000000000000000, 1.000000000000000000, 1.000000000000000000, 1.000000000000000000, 1.000000000000000000, 1.000000000000000000, 1.000000000000000000, 1.000000000000000000, 1.000000000000000000, 1.000000000000000000, 1.000000000000000000, 1.000000000000000000, 1.000000000000000000, 1.000000000000000000, 1.000000000000000000, 1.000000000000000000, 1.000000000000000000, 1.000000000000000000, 1.000000000000000000, 1.000000000000000000, 1.000000000000000000, 1.000000000000000000, 1.000000000000000000, 1.000000000000000000, 1.000000000000000000, 1.000000000000000000, 1.000000000000000000, 1.000000000000000000, 1.000000000000000000, 1.000000000000000000, 1.000000000000000000, 1.000000000000000000, 1.000000000000000000, 1.000000000000000000, 1.000000000000000000, 1.000000000000000000, 1.000000000000000000, 1.000000000000000000, 1.000000000000000000, 1.000000000000000000, 1.000000000000000000, 1.000000000000000000, 1.000000000000000000, 1.000000000000000000, 1.000000000000000000, 1.000000000000000000, 1.000000000000000000, 1.000000000000000000, 1.000000000000000000, 1.000000000000000000, 1.000000000000000000, 1.000000000000000000, 1.000000000000000000, 1.000000000000000000, 1.000000000000000000, 1.000000000000000000, 1.000000000000000000, 1.000000000000000000, 1.000000000000000000, 1.000000000000000000, 1.000000000000000000, 1.000000000000000000, 1.000000000000000000, 1.000000000000000000, 1.000000000000000000, 1.000000000000000000, 1.000000000000000000, 1.000000000000000000, 1.000000000000000000, 1.000000000000000000, 1.000000000000000000, 1.000000000000000000, 1.000000000000000000, 1.000000000000000000, 1.000000000000000000, 1.000000000000000000, 1.000000000000000000, 1.000000000000000000, 1.000000000000000000, 1.000000000000000000, 1.000000000000000000, 1.000000000000000000, 1.000000000000000000, 1.000000000000000000, 1.000000000000000000, 1.000000000000000000, 1.000000000000000000, 1.000000000000000000, 1.000000000000000000, 1.000000000000000000, 1.000000000000000000, 1.000000000000000000, 1.000000000000000000, 1.000000000000000000, 1.000000000000000000, 1.000000000000000000, 1.000000000000000000, 1.000000000000000000, 1.000000000000000000, 1.000000000000000000, 1.000000000000000000, 1.000000000000000000, 1.000000000000000000, 1.000000000000000000, 1.000000000000000000, 1.000000000000000000, 1.000000000000000000, 1.000000000000000000, 1.000000000000000000, 1.000000000000000000, 1.000000000000000000, 1.000000000000000000, 1.000000000000000000, 1.000000000000000000, 1.000000000000000000, 1.000000000000000000, 1.000000000000000000, 1.000000000000000000, 1.000000000000000000, 1.000000000000000000, 1.000000000000000000, 1.000000000000000000, 1.000000000000000000, 1.000000000000000000, 1.000000000000000000, 1.000000000000000000, 1.000000000000000000, 1.000000000000000000, 1.000000000000000000, 1.000000000000000000, 1.000000000000000000, 1.000000000000000000, 1.000000000000000000, 1.000000000000000000, 1.000000000000000000, 1.000000000000000000, 1.000000000000000000, 1.000000000000000000, 1.000000000000000000, 1.000000000000000000, 1.000000000000000000, 1.000000000000000000, 1.000000000000000000, 1.000000000000000000, 1.000000000000000000, 1.000000000000000000, 1.000000000000000000, 1.000000000000000000, 1.000000000000000000) ) ) 
 REPRESENTATION_ITEM ( '' )  SURFACE ( )  );
#10309=CARTESIAN_POINT ( 'NONE',  ( -37.56526046546249376, -113.9929510916434339, 13.11451721564129258 ) ) ;
#10311=CARTESIAN_POINT ( 'NONE',  ( -36.62499999999902656, -115.9929510916434481, 13.11852480586264846 ) ) ;
#10321=CARTESIAN_POINT ( 'NONE',  ( -35.50000000000000711, -112.7549084230351752, -1.592823285203595285 ) ) ;
#10330=CARTESIAN_POINT ( 'NONE',  ( -35.50000000000000000, -113.6807644833805995, -2.624782352598442614 ) ) ;
#10333=CARTESIAN_POINT ( 'NONE',  ( -37.47347596530441649, -114.9754527089670262, 7.972274454178450043 ) ) ;
#10340=CARTESIAN_POINT ( 'NONE',  ( -34.50000000000000000, -113.8474311500459777, -0.6247823525984269599 ) ) ;
#10344=CARTESIAN_POINT ( 'NONE',  ( -38.00000000000000711, -114.9929510916434339, 12.44250253426874941 ) ) ;
#10348=CARTESIAN_POINT ( 'NONE',  ( -34.50000000000000000, -112.0414288467712112, 1.115164475686276191 ) ) ;
#10356=CARTESIAN_POINT ( 'NONE',  ( -36.06250000000000711, -115.9929510916434481, 13.11852480586264846 ) ) ;
#10379=CARTESIAN_POINT ( 'NONE',  ( -36.11231047232249125, -115.9754527089670262, 4.277725545821551734 ) ) ;
#10393=CARTESIAN_POINT ( 'NONE',  ( -35.00000000000000000, -113.9407375970687895, 2.496475545821554398 ) ) ;
#10401=CARTESIAN_POINT ( 'NONE',  ( -35.54388159064475872, -112.6276912846090568, 4.316024454178448266 ) ) ;
#10403=CARTESIAN_POINT ( 'NONE',  ( -34.51202277066418844, -115.9929510916434481, 12.81430620224972294 ) ) ;
#10414=CARTESIAN_POINT ( 'NONE',  ( -38.97545270896704039, -114.8876895276775087, 6.152725545821551734 ) ) ;
#10432=CARTESIAN_POINT ( 'NONE',  ( -35.50000000000000711, -112.6605569508015350, 1.812590711673265575 ) ) ;
#10439=CARTESIAN_POINT ( 'NONE',  ( -34.50000000000000000, -112.0141053790792114, 0.9054673897245171243 ) ) ;
#10441=CARTESIAN_POINT ( 'NONE',  ( -34.50000000000000000, -114.9929510916434339, 10.51725893871048889 ) ) ;
#10443=CARTESIAN_POINT ( 'NONE',  ( -37.99974912065192711, -114.9929510916434339, 12.63488142334838571 ) ) ;
#10445=CARTESIAN_POINT ( 'NONE',  ( -34.50000000000000000, -114.9922651054798308, 10.46846006712531008 ) ) ;
#10453=CARTESIAN_POINT ( 'NONE',  ( -38.00000000000000711, -114.9929510916434339, 12.59652202191340820 ) ) ;
#10456=CARTESIAN_POINT ( 'NONE',  ( -35.54388159064475872, -112.6276912846090568, 8.816024454178448266 ) ) ;
#10465=CARTESIAN_POINT ( 'NONE',  ( -39.07941549657748936, -111.8367748094582055, 2.441024454178448710 ) ) ;
#10474=CARTESIAN_POINT ( 'NONE',  ( -34.50000000000000000, -111.0360125565790383, 1.176611260687384419 ) ) ;
#10477=CARTESIAN_POINT ( 'NONE',  ( -35.50000000000000711, -114.1152303497977414, 9.513755561829650986 ) ) ;
#10479=CARTESIAN_POINT ( 'NONE',  ( -34.50000000000000000, -113.9929510916434339, 10.50625754673588474 ) ) ;
#10483=CARTESIAN_POINT ( 'NONE',  ( -37.51635661748575501, -113.9929510916434339, 13.11827392651459512 ) ) ;
#10484=CARTESIAN_POINT ( 'NONE',  ( -37.99839555572501837, -115.9929510916434481, 12.65937477241749143 ) ) ;
#10494=CARTESIAN_POINT ( 'NONE',  ( -35.50000000000000711, -115.5178116849130276, -1.498529437126731034 ) ) ;
#10496=CARTESIAN_POINT ( 'NONE',  ( -35.50000000000000711, -114.9929510916434339, 11.73841344789270202 ) ) ;
#10500=CARTESIAN_POINT ( 'NONE',  ( -35.50000000000000000, -111.0140978167138570, 0.3752176474015639918 ) ) ;
#10504=CARTESIAN_POINT ( 'NONE',  ( -37.66520193420439000, -113.2509883718312977, 8.441024454178448266 ) ) ;
#10510=CARTESIAN_POINT ( 'NONE',  ( -34.50000000000000000, -114.9307644833806137, -0.6247823525984269599 ) ) ;
#10516=CARTESIAN_POINT ( 'NONE',  ( -37.24999999999992895, -114.9929510916434339, 13.11852480586264669 ) ) ;
#10519=CARTESIAN_POINT ( 'NONE',  ( -34.50000000000000000, -112.0140978167138712, 0.0002176474015661141945 ) ) ;
#10527=CARTESIAN_POINT ( 'NONE',  ( -35.50000000000000711, -114.0371586325023117, 9.504435485030890973 ) ) ;
#10548=CARTESIAN_POINT ( 'NONE',  ( -38.45611840935523418, -112.6276912846090568, 7.933975545821552622 ) ) ;
#10569=CARTESIAN_POINT ( 'NONE',  ( -38.37230871539094323, -112.5438815906447729, 3.941024454178448710 ) ) ;
#10571=CARTESIAN_POINT ( 'NONE',  ( -35.51674767832922441, -115.9929510916434481, 14.04194344061634325 ) ) ;
#10582=CARTESIAN_POINT ( 'NONE',  ( -37.05926240293131713, -111.0000000000000284, 8.121475545821549957 ) ) ;
#10601=CARTESIAN_POINT ( 'NONE',  ( -35.50000000000000000, -117.0140978167138854, 0.3752176474015736507 ) ) ;
#10610=CARTESIAN_POINT ( 'NONE',  ( -34.50000000000000000, -112.0221129971568104, -0.7553032835231431319 ) ) ;
#10611=CARTESIAN_POINT ( 'NONE',  ( -37.98325232167028531, -114.9929510916434339, 14.04194344061727406 ) ) ;
#10613=CARTESIAN_POINT ( 'NONE',  ( -35.50000000000000000, -113.9929510916434339, 10.50625754673588474 ) ) ;
#10615=CARTESIAN_POINT ( 'NONE',  ( -34.50000000000000000, -114.9929510916434339, 10.59426868253284226 ) ) ;
#10618=CARTESIAN_POINT ( 'NONE',  ( -38.00000000000000711, -114.9929510916434339, 11.91443571948719615 ) ) ;
#10624=CARTESIAN_POINT ( 'NONE',  ( -36.15625000000007816, -114.9929510916434339, 13.11852480586264669 ) ) ;
#10626=CARTESIAN_POINT ( 'NONE',  ( -39.02454729103295961, -114.7691647218148745, 8.159774454178448266 ) ) ;
#10636=CARTESIAN_POINT ( 'NONE',  ( -38.18337828418795965, -110.9754527089670546, 5.534774454178449155 ) ) ;
#10649=CARTESIAN_POINT ( 'NONE',  ( -34.50000000000000000, -111.0140978167138570, -0.3122823525984338988 ) ) ;
#10654=CARTESIAN_POINT ( 'NONE',  ( -35.50000000000000711, -114.9929510916434339, 10.51175824272318415 ) ) ;
#10656=CARTESIAN_POINT ( 'NONE',  ( -36.62499999999902656, -113.9929510916434339, 14.11852480586265024 ) ) ;
#10660=CARTESIAN_POINT ( 'NONE',  ( -38.00000000000000711, -113.9929510916434339, 11.21034663311206181 ) ) ;
#10662=CARTESIAN_POINT ( 'NONE',  ( -37.48437500000004263, -115.9929510916434481, 13.11852480586264846 ) ) ;
#10674=CARTESIAN_POINT ( 'NONE',  ( -35.50000000000000000, -113.1061333991432321, 0.8862035858144284850 ) ) ;
#10676=CARTESIAN_POINT ( 'NONE',  ( -35.50000000000000711, -114.9929510916434339, 10.56126450660895699 ) ) ;
#10683=CARTESIAN_POINT ( 'NONE',  ( -35.50000000000000000, -111.0140821919592327, -0.5779076015960634694 ) ) ;
#10686=CARTESIAN_POINT ( 'NONE',  ( -35.02454729103298803, -114.8876895276775087, 3.097274454178448710 ) ) ;
#10691=CARTESIAN_POINT ( 'NONE',  ( -34.50000000000000000, -113.0140978167139991, 0.8595926474015699315 ) ) ;
#10695=CARTESIAN_POINT ( 'NONE',  ( -37.42187499999997158, -114.9929510916434339, 13.11852480586264669 ) ) ;
#10698=CARTESIAN_POINT ( 'NONE',  ( -34.50000000000000000, -112.1222502514821144, 1.343475657184566296 ) ) ;
#10699=CARTESIAN_POINT ( 'NONE',  ( -34.50000000000000000, -115.9929510916434481, 12.56351784598954424 ) ) ;
#10704=CARTESIAN_POINT ( 'NONE',  ( -35.50000000000000711, -114.1264797827112574, 9.515205387299289441 ) ) ;
#10727=CARTESIAN_POINT ( 'NONE',  ( -36.23083527818512550, -111.9754527089670404, 6.715225545821551734 ) ) ;
#10735=AXIS2_PLACEMENT_3D ( 'NONE', #29539, #15638, #32051 ) ;
#10750=CARTESIAN_POINT ( 'NONE',  ( -37.88878409051687157, -115.9929510916434481, 14.07058620477052280 ) ) ;
#10760=CARTESIAN_POINT ( 'NONE',  ( -38.97545270896704039, -114.8876895276775087, 4.652725545821551734 ) ) ;
#10791=CARTESIAN_POINT ( 'NONE',  ( -34.50000000000000000, -115.0468226098135744, -1.624774171496087716 ) ) ;
#10793=CARTESIAN_POINT ( 'NONE',  ( -35.90191880024783444, -114.9929510916434339, 14.11551573851448893 ) ) ;
#10795=CARTESIAN_POINT ( 'NONE',  ( -35.50000000000000000, -113.8814751941377352, 10.49295109164313722 ) ) ;
#10797=CARTESIAN_POINT ( 'NONE',  ( -34.50015059926905536, -114.9929510916434339, 12.64306614848962695 ) ) ;
#10807=CARTESIAN_POINT ( 'NONE',  ( -36.07812499999994316, -114.9929510916434339, 13.11852480586264669 ) ) ;
#10809=CARTESIAN_POINT ( 'NONE',  ( -38.99999999999999289, -113.9407375970686900, 6.753524454178448266 ) ) ;
#10822=CARTESIAN_POINT ( 'NONE',  ( -37.05926240293133134, -116.9999999999999858, 6.378524454178448266 ) ) ;
#10831=EDGE_CURVE ( 'NONE', #12890, #35474, #24750, .T. ) ;
#10835=CARTESIAN_POINT ( 'NONE',  ( -34.50000000000000000, -114.3474311500471572, -2.624782352598442614 ) ) ;
#10838=CARTESIAN_POINT ( 'NONE',  ( -35.50000000000000711, -114.0371586325023117, 9.504435485030890973 ) ) ;
#10839=CARTESIAN_POINT ( 'NONE',  ( -34.50000000000000000, -113.9929510916434339, 12.44250253426871033 ) ) ;
#10842=CARTESIAN_POINT ( 'NONE',  ( -34.50000000000000000, -113.9929510916434339, 12.59102132592610346 ) ) ;
#10843=CARTESIAN_POINT ( 'NONE',  ( -37.74437085908087397, -114.9929510916434339, 14.09929883582536903 ) ) ;
#10845=CARTESIAN_POINT ( 'NONE',  ( -35.50000000000000711, -114.9929510916434339, 10.61627146648203812 ) ) ;
#10857=CARTESIAN_POINT ( 'NONE',  ( -35.50000000000000000, -113.7503824761461004, 0.9631051547057219997 ) ) ;
#10859=CARTESIAN_POINT ( 'NONE',  ( -37.99999999999998579, -113.9407375970686758, 6.753524454178450043 ) ) ;
#10862=CARTESIAN_POINT ( 'NONE',  ( -35.50000000000000711, -114.9929510916434339, 12.59102132592610523 ) ) ;
#10866=CARTESIAN_POINT ( 'NONE',  ( -35.50000000000000000, -111.0140978167138570, 0.7189676474015717078 ) ) ;
#10869=CARTESIAN_POINT ( 'NONE',  ( -37.05926240293131713, -115.9999999999999858, 1.878524454178448710 ) ) ;
#10876=CARTESIAN_POINT ( 'NONE',  ( -34.50000000000000000, -115.0140978167138712, -0.6247823525984408377 ) ) ;
#10880=CARTESIAN_POINT ( 'NONE',  ( -35.50000000000000000, -113.9929510916434339, 11.21034663311132107 ) ) ;
#10883=CARTESIAN_POINT ( 'NONE',  ( -34.50000000000000000, -114.9307644833806137, -1.624782352598427959 ) ) ;
#10885=CARTESIAN_POINT ( 'NONE',  ( -35.75562914091914024, -115.9929510916434481, 14.09929883582542409 ) ) ;
#10891=CARTESIAN_POINT ( 'NONE',  ( -37.99599240977853754, -115.9929510916434481, 12.68378527132499656 ) ) ;
#10912=CARTESIAN_POINT ( 'NONE',  ( -39.02454729103295961, -113.2308352781851539, 9.340225545821549957 ) ) ;
#10921=CARTESIAN_POINT ( 'NONE',  ( -35.50000000000000711, -114.0371586325023117, 9.504435485030890973 ) ) ;
#10931=CARTESIAN_POINT ( 'NONE',  ( -36.31249999999994316, -115.9929510916434481, 14.11852480586265024 ) ) ;
#10940=CARTESIAN_POINT ( 'NONE',  ( -37.88768952767750875, -112.0245472910329880, 6.527725545821550845 ) ) ;
#10965=CARTESIAN_POINT ( 'NONE',  ( -34.50000000000000000, -112.0140900043366088, -0.5935324770972457697 ) ) ;
#10967=CARTESIAN_POINT ( 'NONE',  ( -37.37500000000009237, -114.9929510916434339, 14.11852480586264846 ) ) ;
#10969=CARTESIAN_POINT ( 'NONE',  ( -38.00000000000000711, -114.9929510916434339, 12.17846912687782179 ) ) ;
#10972=CARTESIAN_POINT ( 'NONE',  ( -34.50000000000000000, -114.9929510916434339, 11.91443571948719971 ) ) ;
#10983=CARTESIAN_POINT ( 'NONE',  ( -39.07941549657748936, -111.8367748094582055, 5.441024454178449155 ) ) ;
#10990=CARTESIAN_POINT ( 'NONE',  ( -34.00000000000000000, -113.9407375970686758, 3.996475545821551734 ) ) ;
#11002=CARTESIAN_POINT ( 'NONE',  ( -35.50000000000000000, -111.0140978167138570, 0.2502176474015764263 ) ) ;
#11008=CARTESIAN_POINT ( 'NONE',  ( -34.50000000000000000, -113.9929510916434339, 10.68227981832981044 ) ) ;
#11014=CARTESIAN_POINT ( 'NONE',  ( -34.68937937320795584, -113.9929510916434339, 13.37409560816408671 ) ) ;
#11015=CARTESIAN_POINT ( 'NONE',  ( -38.98077402996267438, -114.9929510916434339, 12.86289566494346204 ) ) ;
#11016=CARTESIAN_POINT ( 'NONE',  ( -35.50000000000000711, -114.0371586325023117, 9.504435485030890973 ) ) ;
#11023=MECHANICAL_DESIGN_GEOMETRIC_PRESENTATION_REPRESENTATION('',(#14466),#7568);
#11032=CARTESIAN_POINT ( 'NONE',  ( -35.50000000000000000, -112.9990795116828650, 0.8734249692896993711 ) ) ;
#11034=CARTESIAN_POINT ( 'NONE',  ( -37.47347596530441649, -114.9754527089670262, 4.972274454178449155 ) ) ;
#11038=CARTESIAN_POINT ( 'NONE',  ( -35.50000000000000000, -117.0140978167138854, 0.0002176474015578471800 ) ) ;
#11041=CARTESIAN_POINT ( 'NONE',  ( -36.11231047232249125, -112.0245472910329880, 7.222274454178451819 ) ) ;
#11046=CARTESIAN_POINT ( 'NONE',  ( -34.50000000000000000, -115.0140978167143402, -0.6247823525984417259 ) ) ;
#11052=CARTESIAN_POINT ( 'NONE',  ( -35.50000000000000000, -113.9929510916434339, 12.50851088611648265 ) ) ;
#11057=CARTESIAN_POINT ( 'NONE',  ( -34.50000000000000000, -115.5178116849130276, -1.498529437126731034 ) ) ;
#11058=CARTESIAN_POINT ( 'NONE',  ( -38.98797722933581866, -115.9929510916434481, 12.81430620224974959 ) ) ;
#11064=CARTESIAN_POINT ( 'NONE',  ( -35.50000000000000711, -114.2598117360253696, 9.542047897280109936 ) ) ;
#11085=CARTESIAN_POINT ( 'NONE',  ( -37.97545270896702618, -114.4734759653044023, 4.652725545821551734 ) ) ;
#11096=CARTESIAN_POINT ( 'NONE',  ( -35.50000000000000711, -114.0928965812550757, 9.511088712577292270 ) ) ;
#11106=CARTESIAN_POINT ( 'NONE',  ( -38.99999693208653895, -115.9929510916434481, 12.62875129555797749 ) ) ;
#11114=CARTESIAN_POINT ( 'NONE',  ( -36.23083527818512550, -111.9754527089670404, 6.715225545821551734 ) ) ;
#11140=CARTESIAN_POINT ( 'NONE',  ( -34.50000000000000000, -114.1807644833817648, -1.624782352598427959 ) ) ;
#11142=CARTESIAN_POINT ( 'NONE',  ( -36.50000000000011369, -114.9929510916434339, 14.11852480586264846 ) ) ;
#11144=CARTESIAN_POINT ( 'NONE',  ( -38.00000068757622529, -114.9929510916434339, 12.61439929482944855 ) ) ;
#11146=CARTESIAN_POINT ( 'NONE',  ( -34.50000306791346816, -114.9929510916434339, 12.62875129555796150 ) ) ;
#11155=CARTESIAN_POINT ( 'NONE',  ( -39.07941549657748936, -111.8367748094582055, 3.941024454178448710 ) ) ;
#11162=CARTESIAN_POINT ( 'NONE',  ( -34.02454729103298092, -115.3019030900506294, 6.097274454178449155 ) ) ;
#11174=CARTESIAN_POINT ( 'NONE',  ( -35.50000000000000000, -112.8230659962028994, 2.866612799894348029 ) ) ;
#11178=CARTESIAN_POINT ( 'NONE',  ( -36.00585935943767169, -114.9929510916434339, 13.11852578240983291 ) ) ;
#11179=CARTESIAN_POINT ( 'NONE',  ( -34.57658136524561598, -113.9929510916434339, 13.10177712753338675 ) ) ;
#11182=CARTESIAN_POINT ( 'NONE',  ( -34.50000000000000000, -113.9929510916434197, 10.50625754673586876 ) ) ;
#11183=CARTESIAN_POINT ( 'NONE',  ( -38.81062062679291103, -114.9929510916434339, 13.37409560816442067 ) ) ;
#11184=CARTESIAN_POINT ( 'NONE',  ( -38.00000000000000711, -115.9929510916434481, 11.21034663311206181 ) ) ;
#11197=CARTESIAN_POINT ( 'NONE',  ( -35.50000000000000000, -113.0140978167137860, 0.8752176474016654106 ) ) ;
#11199=CARTESIAN_POINT ( 'NONE',  ( -35.02454729103298803, -114.8876895276775087, 6.097274454178449155 ) ) ;
#11204=CARTESIAN_POINT ( 'NONE',  ( -35.50000000000000711, -112.7765286249690035, 1.847058736912741583 ) ) ;
#11208=CARTESIAN_POINT ( 'NONE',  ( -37.76916472181487450, -111.9754527089670404, 8.534774454178448266 ) ) ;
#11211=ORIENTED_EDGE ( 'NONE', *, *, #9124, .T. ) ;
#11212=CARTESIAN_POINT ( 'NONE',  ( -34.50000000000000000, -113.8159288351371714, 1.978028123174813802 ) ) ;
#11223=CARTESIAN_POINT ( 'NONE',  ( -35.50000000000000000, -113.9929510916435049, 10.50625754673586876 ) ) ;
#11226=CARTESIAN_POINT ( 'NONE',  ( -34.50000000000000000, -111.6790780953339066, 2.383953864837686343 ) ) ;
#11227=CARTESIAN_POINT ( 'NONE',  ( -37.56132887387857267, -115.9929510916434481, 14.11732072679899197 ) ) ;
#11232=CARTESIAN_POINT ( 'NONE',  ( -35.50000000000000711, -114.4026847875275337, 9.592046023459676718 ) ) ;
#11252=CARTESIAN_POINT ( 'NONE',  ( -37.47347596530441649, -113.0245472910329880, 5.027725545821551734 ) ) ;
#11260=CARTESIAN_POINT ( 'NONE',  ( -35.50000000000000711, -113.0106174888879877, 1.881901162060937827 ) ) ;
#11273=CARTESIAN_POINT ( 'NONE',  ( -37.24999999999992184, -115.9929510916434481, 14.11852480586265024 ) ) ;
#11286=CARTESIAN_POINT ( 'NONE',  ( -37.05926240293131713, -112.0000000000000142, 9.621475545821551734 ) ) ;
#11316=CARTESIAN_POINT ( 'NONE',  ( -34.50000000000000000, -113.6807644833805995, -1.624782352598427959 ) ) ;
#11317=CARTESIAN_POINT ( 'NONE',  ( -36.31249999999995026, -114.9929510916434339, 14.11852480586264846 ) ) ;
#11319=CARTESIAN_POINT ( 'NONE',  ( -38.00000000000000711, -114.9929510916434339, 12.60752341388803721 ) ) ;
#11321=CARTESIAN_POINT ( 'NONE',  ( -34.50000000000000000, -114.9929510916434339, 11.38636890470581164 ) ) ;
#11336=CARTESIAN_POINT ( 'NONE',  ( -38.30190309005061522, -116.9754527089670546, 4.972274454178449155 ) ) ;
#11339=CARTESIAN_POINT ( 'NONE',  ( -35.50000000000000711, -115.9630435732166518, -0.9469505670456015434 ) ) ;
#11356=CARTESIAN_POINT ( 'NONE',  ( -34.50000000000000000, -114.9515981487115823, -2.624803185604625000 ) ) ;
#11361=CARTESIAN_POINT ( 'NONE',  ( -35.56312645773537895, -114.9929510916434339, 12.87038173996308998 ) ) ;
#11362=CARTESIAN_POINT ( 'NONE',  ( -34.50000000000000000, -113.9929510916434339, 12.59652202191340464 ) ) ;
#11365=CARTESIAN_POINT ( 'NONE',  ( -34.50000000000000000, -113.9929510916434339, 12.50851088611648265 ) ) ;
#11366=CARTESIAN_POINT ( 'NONE',  ( -38.42182118622945808, -114.9929510916434339, 13.81802396319329773 ) ) ;
#11367=CARTESIAN_POINT ( 'NONE',  ( -35.50000000000000711, -114.9929510916434339, 10.94631322572069365 ) ) ;
#11384=CARTESIAN_POINT ( 'NONE',  ( -35.50000000000000000, -114.9307644833806137, -0.6247823525984269599 ) ) ;
#11386=CARTESIAN_POINT ( 'NONE',  ( -37.76916472181487450, -111.9754527089670404, 2.534774454178448710 ) ) ;
#11392=CARTESIAN_POINT ( 'NONE',  ( -35.50000000000000000, -116.9119893297194324, -1.269118781492768910 ) ) ;
#11395=CARTESIAN_POINT ( 'NONE',  ( -35.62769128460905677, -115.4561184093552413, 4.691024454178448266 ) ) ;
#11399=CARTESIAN_POINT ( 'NONE',  ( -34.50000000000000000, -112.0140900043112282, 0.8439677466545482121 ) ) ;
#11403=CARTESIAN_POINT ( 'NONE',  ( -35.50000000000000000, -113.9929510916434339, 12.26648026267477398 ) ) ;
#11407=CARTESIAN_POINT ( 'NONE',  ( -34.50000000000000000, -113.5133328644208746, 2.949007337991939259 ) ) ;
#11408=CARTESIAN_POINT ( 'NONE',  ( -39.00000000000000000, -115.9929510916434481, 11.91443571948719615 ) ) ;
#11432=CARTESIAN_POINT ( 'NONE',  ( -35.02454729103298803, -113.1123104723225197, 9.902725545821557063 ) ) ;
#11438=CARTESIAN_POINT ( 'NONE',  ( -35.50000000000000711, -116.0140978167138712, -0.3122823525984417259 ) ) ;
#11444=CARTESIAN_POINT ( 'NONE',  ( -34.50000000000000000, -114.1189822439768449, 9.514224058074130852 ) ) ;
#11451=CARTESIAN_POINT ( 'NONE',  ( -35.50000000000000000, -114.1185248058629611, 8.507048908356933836 ) ) ;
#11452=CARTESIAN_POINT ( 'NONE',  ( -35.50000000000000711, -112.0141059978162019, -0.6575071456984691309 ) ) ;
#11459=CARTESIAN_POINT ( 'NONE',  ( -34.97545270896703329, -114.7691647218148745, 7.090225545821550845 ) ) ;
#11484=CARTESIAN_POINT ( 'NONE',  ( -34.50000000000000000, -115.0140978167138712, -0.3122823525984416704 ) ) ;
#11487=CARTESIAN_POINT ( 'NONE',  ( -34.50000000000000000, -114.1185248058629611, 8.507048908356933836 ) ) ;
#11493=CARTESIAN_POINT ( 'NONE',  ( -36.99999999999989342, -114.9929510916434339, 14.11852480586264846 ) ) ;
#11504=CARTESIAN_POINT ( 'NONE',  ( -34.92058450342251064, -116.1632251905417945, 7.691024454178450043 ) ) ;
#11506=CARTESIAN_POINT ( 'NONE',  ( -35.50000000000000711, -113.2224311500466030, -1.624782352598427959 ) ) ;
#11525=CARTESIAN_POINT ( 'NONE',  ( -35.50000000000000000, -111.0687598768285369, 1.355111303971038073 ) ) ;
#11532=CARTESIAN_POINT ( 'NONE',  ( -35.50000000000000711, -114.9929510916434339, 11.91443571948719971 ) ) ;
#11533=CARTESIAN_POINT ( 'NONE',  ( -34.50000000000000000, -114.1489256397697289, 9.518467544735724317 ) ) ;
#11538=CARTESIAN_POINT ( 'NONE',  ( -34.51202277066418844, -113.9929510916434339, 12.81430620224972294 ) ) ;
#11539=CARTESIAN_POINT ( 'NONE',  ( -39.00000206272865455, -114.9929510916434339, 12.61164896875035701 ) ) ;
#11540=CARTESIAN_POINT ( 'NONE',  ( -35.50000000000000711, -114.1091535596544873, 9.513028657562415447 ) ) ;
#11551=CARTESIAN_POINT ( 'NONE',  ( -35.50000000000000000, -113.0140978167138996, -0.6247823525984302906 ) ) ;
#11553=CARTESIAN_POINT ( 'NONE',  ( -37.99999999999998579, -113.9407375970686758, 8.253524454178448266 ) ) ;
#11560=CARTESIAN_POINT ( 'NONE',  ( -35.50000000000000711, -112.7472371723319355, 1.839427296857320648 ) ) ;
#11568=CARTESIAN_POINT ( 'NONE',  ( -34.50000000000000000, -112.0221129971568104, -0.7553032835231431319 ) ) ;
#11574=CARTESIAN_POINT ( 'NONE',  ( -35.50000000000000000, -113.9929510916438460, 10.50625754673626133 ) ) ;
#11579=CARTESIAN_POINT ( 'NONE',  ( -34.50000000000000000, -111.3577635893106361, 2.022004269840791402 ) ) ;
#11580=CARTESIAN_POINT ( 'NONE',  ( -37.69578139638701941, -115.9929510916434481, 14.10650203519847778 ) ) ;
#11598=CARTESIAN_POINT ( 'NONE',  ( -37.35495115944176803, -115.0245472910329880, 5.965225545821550845 ) ) ;
#11608=CARTESIAN_POINT ( 'NONE',  ( -35.50000000000000711, -114.9929296450195721, 10.49869535309826674 ) ) ;
#11612=CARTESIAN_POINT ( 'NONE',  ( -34.50000000000000000, -114.1712995509219724, 9.522174004479579068 ) ) ;
#11615=CARTESIAN_POINT ( 'NONE',  ( -35.50000000000000000, -115.9915791193162420, 10.43066258751475139 ) ) ;
#11617=CARTESIAN_POINT ( 'NONE',  ( -35.50000000000000711, -112.3995503592287690, -1.424448457485529618 ) ) ;
#11624=CARTESIAN_POINT ( 'NONE',  ( -37.76916472181486739, -116.0245472910329880, 7.465225545821551734 ) ) ;
#11653=CARTESIAN_POINT ( 'NONE',  ( -34.50000000000000000, -115.0140978167138712, -0.6247823525983134951 ) ) ;
#11657=CARTESIAN_POINT ( 'NONE',  ( -39.00000000000000711, -114.9929510916434339, 12.53051367006571937 ) ) ;
#11661=CARTESIAN_POINT ( 'NONE',  ( -38.99984940073101569, -114.9929510916434339, 12.64306614848957189 ) ) ;
#11672=CARTESIAN_POINT ( 'NONE',  ( -39.99999999999999289, -113.9407375970686758, 5.253524454178449155 ) ) ;
#11675=CARTESIAN_POINT ( 'NONE',  ( -35.50000000000000711, -113.0974311500471714, -1.624782352598427959 ) ) ;
#11687=CARTESIAN_POINT ( 'NONE',  ( -37.76916472181486739, -116.0245472910329880, 2.965225545821551290 ) ) ;
#11692=CARTESIAN_POINT ( 'NONE',  ( -34.50000000000000000, -117.0140978167138854, -0.4685323525984310122 ) ) ;
#11698=CARTESIAN_POINT ( 'NONE',  ( -35.69272627125609176, -114.9929510916434339, 13.01835785830562209 ) ) ;
#11700=CARTESIAN_POINT ( 'NONE',  ( -37.49023442168701337, -113.9929510916434339, 14.11852773550420359 ) ) ;
#11703=CARTESIAN_POINT ( 'NONE',  ( -35.61121590948313553, -113.9929510916434339, 14.07058620477040733 ) ) ;
#11705=CARTESIAN_POINT ( 'NONE',  ( -35.56312645773537895, -114.9929510916434339, 12.87038173996308998 ) ) ;
#11719=CARTESIAN_POINT ( 'NONE',  ( -35.50000000000000000, -115.0140978167137860, -0.6247823525984395054 ) ) ;
#11722=CARTESIAN_POINT ( 'NONE',  ( -34.97545270896703329, -113.2308352781851539, 4.409774454178448266 ) ) ;
#11724=CARTESIAN_POINT ( 'NONE',  ( -36.94073759706868287, -112.0000000000000142, 5.628524454178449155 ) ) ;
#11727=CARTESIAN_POINT ( 'NONE',  ( -35.50000000000000711, -113.6318576702834804, 1.956056246348823580 ) ) ;
#11731=CARTESIAN_POINT ( 'NONE',  ( -37.05926240293131713, -115.9999999999999858, 4.878524454178449155 ) ) ;
#11737=CARTESIAN_POINT ( 'NONE',  ( -34.50000000000000000, -112.0140978167138712, -0.1247823525984259746 ) ) ;
#11743=CARTESIAN_POINT ( 'NONE',  ( -36.03906250000000000, -113.9929510916434339, 13.11852480586264846 ) ) ;
#11747=CARTESIAN_POINT ( 'NONE',  ( -34.50000000000000000, -111.0140978167138570, 0.0002176474015659786963 ) ) ;
#11749=CARTESIAN_POINT ( 'NONE',  ( -35.50000000000000000, -115.9929510916434481, 10.85830208992344303 ) ) ;
#11774=CARTESIAN_POINT ( 'NONE',  ( -37.35495115944176803, -115.0245472910329880, 7.465225545821552622 ) ) ;
#11780=CARTESIAN_POINT ( 'NONE',  ( -35.50000000000000711, -115.9821387493194891, -0.8839717462762166633 ) ) ;
#11783=CARTESIAN_POINT ( 'NONE',  ( -35.60016694755736921, -114.9929510916434339, 12.92579853460621209 ) ) ;
#11786=CARTESIAN_POINT ( 'NONE',  ( -34.50000000000000000, -114.9929510916434339, 10.56126450660895699 ) ) ;
#11793=CARTESIAN_POINT ( 'NONE',  ( -39.00000000000000000, -115.9929510916434481, 12.50851088611646311 ) ) ;
#11804=CARTESIAN_POINT ( 'NONE',  ( -37.47347596530441649, -113.0245472910329880, 6.527725545821552622 ) ) ;
#11813=CARTESIAN_POINT ( 'NONE',  ( -39.99999999999999289, -114.0592624029313242, 4.746475545821549957 ) ) ;
#11831=CARTESIAN_POINT ( 'NONE',  ( -34.50000000000000000, -113.8474311500459777, -0.6247823525984269599 ) ) ;
#11833=CARTESIAN_POINT ( 'NONE',  ( -34.50000000000000000, -116.0140978167138712, 0.8752176474015622709 ) ) ;
#11834=CARTESIAN_POINT ( 'NONE',  ( -34.50000000000000000, -114.2265172349312508, 8.519938377296172760 ) ) ;
#11836=CARTESIAN_POINT ( 'NONE',  ( -37.05926240293131713, -115.9999999999999858, 1.878524454178448710 ) ) ;
#11837=CARTESIAN_POINT ( 'NONE',  ( -39.00000000000000711, -114.9929510916434339, 10.50625754673587231 ) ) ;
#11848=CARTESIAN_POINT ( 'NONE',  ( -39.97545270896702618, -115.3019030900506152, 3.152725545821551734 ) ) ;
#11852=CARTESIAN_POINT ( 'NONE',  ( -35.50000000000000711, -116.0124910254613297, -0.6902086197697608894 ) ) ;
#11866=ORIENTED_EDGE ( 'NONE', *, *, #2185, .F. ) ;
#11867=CARTESIAN_POINT ( 'NONE',  ( -35.02454729103298092, -113.1123104723225055, 6.902725545821551734 ) ) ;
#11873=CARTESIAN_POINT ( 'NONE',  ( -35.50000000000000000, -111.0397324434303101, -0.9506101647064429949 ) ) ;
#11876=CARTESIAN_POINT ( 'NONE',  ( -36.24999999999983658, -114.9929510916434339, 13.11852480586264669 ) ) ;
#11879=CARTESIAN_POINT ( 'NONE',  ( -39.00000000000000000, -113.9929510916434339, 12.57451923796417681 ) ) ;
#11883=CARTESIAN_POINT ( 'NONE',  ( -37.54906985245723661, -113.9929510916434339, 14.11777216781844757 ) ) ;
#11885=CARTESIAN_POINT ( 'NONE',  ( -36.50000000000011369, -114.9929510916434339, 13.11852480586264669 ) ) ;
#11893=CARTESIAN_POINT ( 'NONE',  ( -35.87040530316090070, -114.9929510916434339, 13.10254527216545917 ) ) ;
#11903=CARTESIAN_POINT ( 'NONE',  ( -35.50000000000000000, -115.0140978167138712, 0.0002176474015578471800 ) ) ;
#11905=CARTESIAN_POINT ( 'NONE',  ( -35.54388159064475872, -112.6276912846090568, 2.816024454178448710 ) ) ;
#11908=CARTESIAN_POINT ( 'NONE',  ( -35.02454729103298803, -114.8876895276775087, 1.597274454178448710 ) ) ;
#11913=CARTESIAN_POINT ( 'NONE',  ( -35.50000000000000711, -116.0140978167138712, -0.5622823525984409487 ) ) ;
#11923=CARTESIAN_POINT ( 'NONE',  ( -34.50000000000000000, -116.0140896356112989, -0.6575071456984549201 ) ) ;
#11932=CARTESIAN_POINT ( 'NONE',  ( -37.34375000000001421, -113.9929510916434339, 13.11852480586264846 ) ) ;
#11934=CARTESIAN_POINT ( 'NONE',  ( -34.50000000000000000, -113.3557509229967764, 1.923098431109107054 ) ) ;
#11937=CARTESIAN_POINT ( 'NONE',  ( -36.00585935943765747, -113.9929510916434339, 13.11852578240983291 ) ) ;
#11939=CARTESIAN_POINT ( 'NONE',  ( -35.50000000000000000, -115.9927366631908825, 10.47601115720670073 ) ) ;
#11965=CARTESIAN_POINT ( 'NONE',  ( -36.25098837183129774, -113.3347980657956242, 2.816024454178448710 ) ) ;
#11977=CARTESIAN_POINT ( 'NONE',  ( -35.50640865667918433, -114.9929510916434339, 12.69998175888958514 ) ) ;
#11980=CARTESIAN_POINT ( 'NONE',  ( -34.50000000000000000, -114.9656200615856818, 10.26631071845107179 ) ) ;
#11985=CARTESIAN_POINT ( 'NONE',  ( -35.50000000000000000, -115.9929510916434481, 10.52000928670414126 ) ) ;
#11986=CARTESIAN_POINT ( 'NONE',  ( -35.50000000000000711, -112.9415908020655195, 1.873661708251232572 ) ) ;
#11991=DIRECTION ( 'NONE',  ( 0.000000000000000000, 0.000000000000000000, -1.000000000000000000 ) ) ;
#11998=CARTESIAN_POINT ( 'NONE',  ( -36.94073759706868287, -115.0000000000000000, 5.871475545821551734 ) ) ;
#12006=CARTESIAN_POINT ( 'NONE',  ( -34.00000000000000000, -114.0592624029313242, 7.503524454178450043 ) ) ;
#12020=CARTESIAN_POINT ( 'NONE',  ( -34.50000000000000000, -112.8655373925166572, 1.864575885149403423 ) ) ;
#12023=CARTESIAN_POINT ( 'NONE',  ( -34.50000000000000000, -115.9929510916434481, 10.61627146648203990 ) ) ;
#12026=CARTESIAN_POINT ( 'NONE',  ( -38.25557080230232998, -114.9929510916434339, 13.92914543265419525 ) ) ;
#12034=CARTESIAN_POINT ( 'NONE',  ( -35.81662171581203324, -110.9754527089670546, 5.215225545821552622 ) ) ;
#12036=CARTESIAN_POINT ( 'NONE',  ( -35.50000000000000711, -116.0140978167138712, -0.3747823525984422255 ) ) ;
#12047=CARTESIAN_POINT ( 'NONE',  ( -35.54388159064475872, -115.3723087153909432, 4.183975545821551734 ) ) ;
#12052=CARTESIAN_POINT ( 'NONE',  ( -35.50000000000000000, -115.3399256288223569, -2.599147725881697291 ) ) ;
#12059=CARTESIAN_POINT ( 'NONE',  ( -34.50000000000000000, -114.0371586325023117, 9.504435485030890973 ) ) ;
#12064=CARTESIAN_POINT ( 'NONE',  ( -36.00976557831293690, -113.9929510916434339, 14.11852773550420359 ) ) ;
#12067=CARTESIAN_POINT ( 'NONE',  ( -35.93473953453761283, -114.9929510916434339, 13.11451721564123574 ) ) ;
#12073=CARTESIAN_POINT ( 'NONE',  ( -35.50000000000000711, -114.8847986568751907, 10.03799953695244618 ) ) ;
#12079=CARTESIAN_POINT ( 'NONE',  ( -35.50000000000000000, -113.0140978167136581, -0.6247823525984268489 ) ) ;
#12084=CARTESIAN_POINT ( 'NONE',  ( -37.05926240293131713, -115.9999999999999858, 1.878524454178448710 ) ) ;
#12089=CARTESIAN_POINT ( 'NONE',  ( -35.50000000000000711, -115.1770117227680998, -1.611965039240062181 ) ) ;
#12098=CARTESIAN_POINT ( 'NONE',  ( -34.50000000000000000, -115.3362660311619692, -1.573728109101206085 ) ) ;
#12107=CARTESIAN_POINT ( 'NONE',  ( -37.51635661748575501, -113.9929510916434339, 13.11827392651459512 ) ) ;
#12108=CARTESIAN_POINT ( 'NONE',  ( -34.50000000000000000, -112.7765286249690035, 1.847058736912741583 ) ) ;
#12112=CARTESIAN_POINT ( 'NONE',  ( -35.97955704204053262, -113.9929510916434339, 13.11812344617474402 ) ) ;
#12114=CARTESIAN_POINT ( 'NONE',  ( -35.50000000000000000, -115.9929510916434481, 12.26648026267477398 ) ) ;
#12125=CARTESIAN_POINT ( 'NONE',  ( -35.50000000000000711, -113.6318576702834804, 1.956056246348823580 ) ) ;
#12132=CARTESIAN_POINT ( 'NONE',  ( -34.50000000000000000, -111.1162063037085801, -1.269118781493287607 ) ) ;
#12137=CARTESIAN_POINT ( 'NONE',  ( -37.35495115944176092, -112.9754527089670688, 4.034774454178449155 ) ) ;
#12142=CARTESIAN_POINT ( 'NONE',  ( -35.50000000000000000, -114.8057644833805853, -0.6247823525984269599 ) ) ;
#12150=CARTESIAN_POINT ( 'NONE',  ( -35.52552712174884419, -114.9929510916434339, 12.77960891308624447 ) ) ;
#12154=CARTESIAN_POINT ( 'NONE',  ( -34.50000000000000000, -114.9929510916434339, 12.56351784598954424 ) ) ;
#12158=CARTESIAN_POINT ( 'NONE',  ( -35.50000000000000000, -115.9929510916434481, 10.53376102667243508 ) ) ;
#12159=CARTESIAN_POINT ( 'NONE',  ( -35.50000000000000711, -112.0140978167138712, 0.0002176474015661141945 ) ) ;
#12169=( GEOMETRIC_REPRESENTATION_CONTEXT ( 3 ) GLOBAL_UNCERTAINTY_ASSIGNED_CONTEXT ( ( #30555 ) ) GLOBAL_UNIT_ASSIGNED_CONTEXT ( ( #8317, #401, #9391 ) ) REPRESENTATION_CONTEXT ( 'NONE', 'WORKASPACE' ) );
#12170=CARTESIAN_POINT ( 'NONE',  ( -35.97545270896705460, -114.3549511594417680, 8.590225545821549957 ) ) ;
#12182=CARTESIAN_POINT ( 'NONE',  ( -35.69809690994941320, -116.9754527089670546, 8.777725545821549957 ) ) ;
#12201=CARTESIAN_POINT ( 'NONE',  ( -34.50000000000000000, -115.0140978167138428, -0.6247823525979866455 ) ) ;
#12204=CARTESIAN_POINT ( 'NONE',  ( -34.50000000000000000, -114.2450133963102843, 8.522190569412378736 ) ) ;
#12207=CARTESIAN_POINT ( 'NONE',  ( -37.52454134262690388, -114.9929510916434339, 14.11837420659362152 ) ) ;
#12215=CARTESIAN_POINT ( 'NONE',  ( -39.07941549657749647, -116.1632251905417803, 4.558975545821549957 ) ) ;
#12217=CARTESIAN_POINT ( 'NONE',  ( -35.50000000000000000, -113.0140978167138712, -0.4997823525984338988 ) ) ;
#12223=B_SPLINE_CURVE_WITH_KNOTS ( 'NONE', 3,
 ( #31246, #17010, #1010, #20063, #6226, #22954, #14485, #9279, #28367, #11986, #20235, #25495, #33580, #17542, #6566, #8914, #25320, #3710, #31069, #19700, #1187, #9103, #812, #30891, #23132, #28548, #3896, #19878, #22773, #14852, #14142, #25861, #8733, #33774, #6048, #12159, #31422, #34128, #20410, #6752, #17728, #3185, #469, #11452, #22418, #33410, #30716, #28020, #3367, #14314, #639, #11617, #17188, #4082, #34848, #4615, #9639, #24052, #32135, #18262, #23310, #12701, #7106, #4252, #34491, #4787, #28903, #7465, #29267, #20773, #26029, #1905, #15189, #26747, #20600, #18445, #29442, #1357, #31598, #34310, #18079, #15730, #31774, #12333, #12880, #26198, #2088, #6933, #13067, #35037, #17906, #1536, #12519, #29080, #28731, #23496, #9810, #23677, #4429, #15372, #26383, #1717 ),
 .UNSPECIFIED., .F., .F.,
 ( 4, 2, 2, 2, 2, 2, 2, 2, 2, 2, 2, 2, 2, 2, 2, 2, 2, 2, 2, 2, 2, 2, 2, 2, 2, 2, 2, 2, 2, 2, 2, 2, 2, 2, 2, 2, 2, 2, 2, 2, 2, 2, 2, 2, 2, 2, 2, 2, 2, 2, 4 ),
 ( 0.000000000000000000, 0.05194669433742771930, 0.07792004150614158242, 0.09090671509049851051, 0.09740005188267697456, 0.1038933886748554386, 0.1123700156520060500, 0.1208466426291566476, 0.1377998965834578704, 0.1717064044920602883, 0.2056129124006627062, 0.2225661663549639291, 0.2310427933321145266, 0.2395194203092651519, 0.2482763131408625423, 0.2570332059724599327, 0.2745469916356546580, 0.3095745629620442196, 0.3446021342884337813, 0.3621159199516285621, 0.3708728127832259247, 0.3796297056148233429, 0.3887999023441631730, 0.3979700990735030031, 0.4163104925321826633, 0.4529912794495420392, 0.4896720663669014151, 0.5080124598255810753, 0.5171826565549209054, 0.5263528532842607355, 0.5380287103930572190, 0.5497045675018538136, 0.5730562817194468916, 0.6197597101546329368, 0.6664631385898189819, 0.6898148528074120600, 0.7014907099162086546, 0.7131665670250051381, 0.7223367637543449682, 0.7315069604836847983, 0.7498473539423643475, 0.7865281408597235568, 0.8232089277770826552, 0.8415493212357623154, 0.8507195179651021455, 0.8598897146944418646, 0.8686466075260392827, 0.8774035003576365899, 0.8949172860208314262, 0.9299448573472208768, 1.000000000000000000 ),
 .UNSPECIFIED. ) ;
#12231=CARTESIAN_POINT ( 'NONE',  ( -36.94073759706868287, -115.9999999999999858, 2.871475545821551290 ) ) ;
#12237=CARTESIAN_POINT ( 'NONE',  ( -35.50000000000000000, -116.7615919857705080, -1.632210089000343700 ) ) ;
#12242=CARTESIAN_POINT ( 'NONE',  ( -38.00000000000000711, -114.9929510916434339, 12.26648026267477043 ) ) ;
#12244=CARTESIAN_POINT ( 'NONE',  ( -37.52454134262689678, -113.9929510916434339, 14.11837420659362152 ) ) ;
#12248=CARTESIAN_POINT ( 'NONE',  ( -38.99879592093640213, -113.9929510916434339, 12.67985367974111277 ) ) ;
#12250=CARTESIAN_POINT ( 'NONE',  ( -37.37500000000009237, -114.9929510916434339, 13.11852480586264669 ) ) ;
#12256=CARTESIAN_POINT ( 'NONE',  ( -35.50000000000000711, -114.9929510916434339, 12.56351784598954424 ) ) ;
#12261=VERTEX_POINT ( 'NONE', #1390 ) ;
#12264=CARTESIAN_POINT ( 'NONE',  ( -34.50000000000000000, -113.0140978167140702, 0.8752176474015694874 ) ) ;
#12268=CARTESIAN_POINT ( 'NONE',  ( -35.54388159064475872, -112.6276912846090568, 4.316024454178448266 ) ) ;
#12271=CARTESIAN_POINT ( 'NONE',  ( -35.50000000000000711, -114.9307644833806137, -1.624782352598427959 ) ) ;
#12277=CIRCLE ( 'NONE', #19181, 0.5000000000000004441 ) ;
#12278=PRESENTATION_STYLE_ASSIGNMENT (( #4190 ) ) ;
#12282=CARTESIAN_POINT ( 'NONE',  ( -34.50000000000000000, -112.1403507321855528, -1.128496220798856253 ) ) ;
#12287=CARTESIAN_POINT ( 'NONE',  ( -37.99839555572501837, -113.9929510916434339, 12.65937477241749143 ) ) ;
#12289=CARTESIAN_POINT ( 'NONE',  ( -35.50000000000000000, -113.9929510916434339, 11.38636890470581164 ) ) ;
#12290=CARTESIAN_POINT ( 'NONE',  ( -35.50000000000000000, -115.9929492010520846, 10.50058572605509966 ) ) ;
#12304=CARTESIAN_POINT ( 'NONE',  ( -35.50000000000000711, -114.1712995509219724, 9.522174004479579068 ) ) ;
#12309=CARTESIAN_POINT ( 'NONE',  ( -34.50000000000000000, -114.8057644833805853, -2.624782352598442614 ) ) ;
#12313=CARTESIAN_POINT ( 'NONE',  ( -36.64504884055821776, -112.9754527089670688, 9.715225545821551734 ) ) ;
#12319=CARTESIAN_POINT ( 'NONE',  ( -35.50000000000000000, -115.0140978167138712, -0.6247823525984407267 ) ) ;
#12324=CARTESIAN_POINT ( 'NONE',  ( -35.96730626674924025, -114.9929510916434339, 13.11752178341330044 ) ) ;
#12328=CARTESIAN_POINT ( 'NONE',  ( -34.50000000000000000, -114.9929510916434339, 12.59102132592610523 ) ) ;
#12332=CARTESIAN_POINT ( 'NONE',  ( -35.50000000000000000, -115.9929510916434481, 12.44250253426871033 ) ) ;
#12333=CARTESIAN_POINT ( 'NONE',  ( -35.50000000000000711, -115.8137639216009234, -1.239329810084483841 ) ) ;
#12346=CARTESIAN_POINT ( 'NONE',  ( -37.74901162816868805, -113.3347980657955958, 7.933975545821553510 ) ) ;
#12354=CARTESIAN_POINT ( 'NONE',  ( -34.02454729103297382, -112.6980969099494132, 6.902725545821551734 ) ) ;
#12371=CARTESIAN_POINT ( 'NONE',  ( -34.50000000000000000, -112.0140900043112282, 0.8439677466545482121 ) ) ;
#12375=CARTESIAN_POINT ( 'NONE',  ( -34.50000306791346816, -115.9929510916434481, 12.62875129555796150 ) ) ;
#12380=CARTESIAN_POINT ( 'NONE',  ( -39.00000000000000711, -114.9929510916434339, 11.21034663311206181 ) ) ;
#12389=CARTESIAN_POINT ( 'NONE',  ( -38.18337828418795965, -110.9754527089670546, 8.534774454178448266 ) ) ;
#12392=CARTESIAN_POINT ( 'NONE',  ( -35.50000000000000000, -113.0140978167139991, -0.6247823525984269599 ) ) ;
#12405=CARTESIAN_POINT ( 'NONE',  ( -36.11231047232249836, -115.9754527089670262, 7.277725545821551734 ) ) ;
#12410=CARTESIAN_POINT ( 'NONE',  ( -35.50000000000000000, -114.1807644833817648, -2.624782352598442614 ) ) ;
#12414=CARTESIAN_POINT ( 'NONE',  ( -38.00000000000000711, -114.9929510916434339, 12.17846912687782179 ) ) ;
#12417=CARTESIAN_POINT ( 'NONE',  ( -34.50000000000000000, -114.9929510916434339, 11.38636890470581164 ) ) ;
#12420=CARTESIAN_POINT ( 'NONE',  ( -37.37500000000009237, -114.9929510916434339, 13.11852480586264669 ) ) ;
#12422=CARTESIAN_POINT ( 'NONE',  ( -36.87500000000098765, -113.9929510916434339, 14.11852480586265024 ) ) ;
#12426=CARTESIAN_POINT ( 'NONE',  ( -37.34375000000001421, -114.9929510916434339, 13.11852480586264669 ) ) ;
#12433=CARTESIAN_POINT ( 'NONE',  ( -35.50000000000000711, -114.9860996047076895, 10.38555023491505835 ) ) ;
#12435=CARTESIAN_POINT ( 'NONE',  ( -36.11231047232249125, -112.0245472910329880, 2.722274454178448266 ) ) ;
#12441=CARTESIAN_POINT ( 'NONE',  ( -34.50000000000000000, -113.0140978167138996, -0.6247823525984302906 ) ) ;
#12445=CARTESIAN_POINT ( 'NONE',  ( -38.37230871539094323, -112.5438815906447729, 6.941024454178449155 ) ) ;
#12447=CARTESIAN_POINT ( 'NONE',  ( -35.50000000000000711, -114.6807644833805000, -1.624782352598427959 ) ) ;
#12457=CARTESIAN_POINT ( 'NONE',  ( -34.50000000000000000, -116.0140978167138712, 0.6252176474015648244 ) ) ;
#12459=CARTESIAN_POINT ( 'NONE',  ( -35.50000000000000711, -114.0000000000000853, 2.000000000000001776 ) ) ;
#12467=CARTESIAN_POINT ( 'NONE',  ( -37.62959469683911351, -113.9929510916434339, 13.10254527216511633 ) ) ;
#12469=CARTESIAN_POINT ( 'NONE',  ( -35.50000000000000000, -113.9929510916434339, 12.59102132592610346 ) ) ;
#12471=CARTESIAN_POINT ( 'NONE',  ( -35.60016694755736211, -115.9929510916434481, 12.92579853460621386 ) ) ;
#12480=( GEOMETRIC_REPRESENTATION_CONTEXT ( 3 ) GLOBAL_UNCERTAINTY_ASSIGNED_CONTEXT ( ( #16835 ) ) GLOBAL_UNIT_ASSIGNED_CONTEXT ( ( #29362, #21045, #26483 ) ) REPRESENTATION_CONTEXT ( 'NONE', 'WORKASPACE' ) );
#12485=CARTESIAN_POINT ( 'NONE',  ( -35.50000000000000711, -114.3474311500471430, -1.624782352598427959 ) ) ;
#12492=CARTESIAN_POINT ( 'NONE',  ( -34.50000000000000000, -117.0140978167138854, 0.0002176474015577929428 ) ) ;
#12496=CARTESIAN_POINT ( 'NONE',  ( -36.33479806579561000, -114.7490116281687165, 3.191024454178448710 ) ) ;
#12500=CARTESIAN_POINT ( 'NONE',  ( -35.50000000000000000, -113.0974311500471714, -0.6247823525984269599 ) ) ;
#12508=CARTESIAN_POINT ( 'NONE',  ( -36.03125000000004263, -114.9929510916434339, 13.11852480586264669 ) ) ;
#12512=CARTESIAN_POINT ( 'NONE',  ( -35.24442919769869320, -114.9929510916434339, 13.92914543265605509 ) ) ;
#12518=CARTESIAN_POINT ( 'NONE',  ( -35.49999931242378182, -115.9929510916434481, 12.61439929482945743 ) ) ;
#12519=CARTESIAN_POINT ( 'NONE',  ( -35.50000000000000711, -116.0140978167138712, -0.5622823525984409487 ) ) ;
#12526=CIRCLE ( 'NONE', #17103, 0.5000000000000004441 ) ;
#12531=CARTESIAN_POINT ( 'NONE',  ( -37.74901162816868805, -113.3347980657955958, 9.433975545821549957 ) ) ;
#12541=CARTESIAN_POINT ( 'NONE',  ( -34.00000000000000000, -113.9407375970686758, 5.496475545821551734 ) ) ;
#12562=CARTESIAN_POINT ( 'NONE',  ( -34.51202277066418844, -115.9929510916434481, 12.81430620224972294 ) ) ;
#12564=CARTESIAN_POINT ( 'NONE',  ( -36.11231047232249836, -112.0245472910329880, 2.722274454178448710 ) ) ;
#12566=CARTESIAN_POINT ( 'NONE',  ( -34.80050084267116972, -115.9929510916434481, 13.54034599209289347 ) ) ;
#12576=CARTESIAN_POINT ( 'NONE',  ( -38.18337828418796676, -117.0245472910329738, 5.965225545821550845 ) ) ;
#12578=CARTESIAN_POINT ( 'NONE',  ( -35.50000000000000000, -113.0601156079281253, 0.8807106166081309917 ) ) ;
#12587=ADVANCED_FACE ( 'NONE', ( #27666 ), #10306, .F. ) ;
#12597=CARTESIAN_POINT ( 'NONE',  ( -35.50000000000000000, -114.6807644833805000, -2.624782352598442614 ) ) ;
#12604=CARTESIAN_POINT ( 'NONE',  ( -34.50000000000000000, -114.6604609523327838, 9.751889438017201428 ) ) ;
#12607=CARTESIAN_POINT ( 'NONE',  ( -37.56526046546250086, -114.9929510916434339, 13.11451721564129258 ) ) ;
#12609=CARTESIAN_POINT ( 'NONE',  ( -34.50000000000000000, -114.0650276068786582, 9.507762098804159123 ) ) ;
#12618=CARTESIAN_POINT ( 'NONE',  ( -35.50025087934803736, -114.9929510916434339, 12.63488142334835196 ) ) ;
#12621=CARTESIAN_POINT ( 'NONE',  ( -35.54388159064475872, -112.6276912846090568, 2.816024454178448710 ) ) ;
#12626=CARTESIAN_POINT ( 'NONE',  ( -34.50000000000000000, -113.0140978167141128, -0.6247823525984907977 ) ) ;
#12628=CARTESIAN_POINT ( 'NONE',  ( -37.05926240293131713, -115.9999999999999858, 7.878524454178450043 ) ) ;
#12630=CARTESIAN_POINT ( 'NONE',  ( -38.30190309005061522, -116.9754527089670546, 3.472274454178448710 ) ) ;
#12634=CARTESIAN_POINT ( 'NONE',  ( -35.50000000000000711, -112.0140978167138712, 0.3752176474015640473 ) ) ;
#12644=CARTESIAN_POINT ( 'NONE',  ( -34.50000000000000000, -115.9821387493194891, -0.8839717462762166633 ) ) ;
#12655=CARTESIAN_POINT ( 'NONE',  ( -34.50000000000000000, -113.9929510916430075, 10.50625754673586876 ) ) ;
#12657=CARTESIAN_POINT ( 'NONE',  ( -36.62499999999902656, -113.9929510916434339, 13.11852480586264846 ) ) ;
#12658=CARTESIAN_POINT ( 'NONE',  ( -37.80727372874345349, -115.9929510916434481, 13.01835785830664705 ) ) ;
#12669=CARTESIAN_POINT ( 'NONE',  ( -35.50000000000000711, -112.7765286249690035, 1.847058736912741583 ) ) ;
#12675=CARTESIAN_POINT ( 'NONE',  ( -35.50000000000000711, -114.0371586325023117, 9.504435485030890973 ) ) ;
#12680=CARTESIAN_POINT ( 'NONE',  ( -34.50000000000000000, -111.0397324434303101, -0.9506101647064429949 ) ) ;
#12684=CARTESIAN_POINT ( 'NONE',  ( -37.66520193420439000, -113.2509883718312977, 5.441024454178449155 ) ) ;
#12687=CARTESIAN_POINT ( 'NONE',  ( -35.50000000000000000, -115.0140978167138712, 0.6252176474015650465 ) ) ;
#12690=AXIS2_PLACEMENT_3D ( 'NONE', #6442, #858, #8958 ) ;
#12691=CARTESIAN_POINT ( 'NONE',  ( -37.99959864031215773, -114.9929510916434339, 12.63896776382213538 ) ) ;
#12695=CARTESIAN_POINT ( 'NONE',  ( -34.50300906734827322, -114.9929510916434339, 12.71660600561482468 ) ) ;
#12700=CARTESIAN_POINT ( 'NONE',  ( -35.99386409314529800, -115.9929510916434481, 13.11852378322482515 ) ) ;
#12701=CARTESIAN_POINT ( 'NONE',  ( -35.50000000000000711, -113.1807644833805426, -1.624782352598427959 ) ) ;
#12712=CARTESIAN_POINT ( 'NONE',  ( -35.99999999999999289, -114.0592624029313242, 3.003524454178448710 ) ) ;
#12721=CARTESIAN_POINT ( 'NONE',  ( -38.97545270896704039, -114.8876895276775087, 3.152725545821551290 ) ) ;
#12725=DIRECTION ( 'NONE',  ( 0.000000000000000000, 0.000000000000000000, 1.000000000000000000 ) ) ;
#12740=CARTESIAN_POINT ( 'NONE',  ( -34.50000000000000000, -115.9929510916434481, 11.21034663311132107 ) ) ;
#12742=CARTESIAN_POINT ( 'NONE',  ( -35.00000000000000000, -114.0592624029313242, 3.003524454178448710 ) ) ;
#12744=CARTESIAN_POINT ( 'NONE',  ( -34.50120407906360498, -115.9929510916434481, 12.67985367974112343 ) ) ;
#12753=CARTESIAN_POINT ( 'NONE',  ( -35.02454729103298803, -113.1123104723225197, 3.902725545821551290 ) ) ;
#12755=CARTESIAN_POINT ( 'NONE',  ( -35.50000000000000000, -113.0140978167156902, -0.6247823525984268489 ) ) ;
#12774=CARTESIAN_POINT ( 'NONE',  ( -35.50000000000000711, -112.0141053790792114, 0.9054673897245171243 ) ) ;
#12780=CARTESIAN_POINT ( 'NONE',  ( -34.50000000000000000, -112.0414288467712112, 1.115164475686276191 ) ) ;
#12781=CARTESIAN_POINT ( 'NONE',  ( -34.50000000000000000, -114.2598117360253696, 9.542047897280109936 ) ) ;
#12783=CARTESIAN_POINT ( 'NONE',  ( -35.56312645773537895, -114.9929510916434339, 12.87038173996308998 ) ) ;
#12785=CARTESIAN_POINT ( 'NONE',  ( -34.50000000000000000, -114.9928438774171582, 10.49113435197128652 ) ) ;
#12795=CARTESIAN_POINT ( 'NONE',  ( -37.34375000000001421, -114.9929510916434339, 13.11852480586264669 ) ) ;
#12799=CARTESIAN_POINT ( 'NONE',  ( -38.97545270896704039, -113.1123104723225197, 3.847274454178449599 ) ) ;
#12805=CARTESIAN_POINT ( 'NONE',  ( -34.50000000000000000, -113.0140978167140702, 0.8752176474015603835 ) ) ;
#12811=CARTESIAN_POINT ( 'NONE',  ( -34.02454729103298092, -115.3019030900506294, 1.597274454178448932 ) ) ;
#12821=CARTESIAN_POINT ( 'NONE',  ( -34.50000000000000000, -111.8727710936879589, 2.535339294948415922 ) ) ;
#12827=CARTESIAN_POINT ( 'NONE',  ( -34.50000000000000000, -113.9929510916432207, 10.50625754673563250 ) ) ;
#12828=( BOUNDED_SURFACE ( )  B_SPLINE_SURFACE ( 3, 2, ( 
 ( #9025, #11908, #31172, #3821, #12084, #1114, #34426, #25791, #31351, #23060, #14781, #1282, #6501, #20167, #23242, #34057, #9204, #33877, #6861, #19988, #9383, #25427, #23428, #17476, #3644, #14593, #20342, #28474, #30993, #25607, #12268, #6678, #4008, #17659, #6327, #28664, #9743, #22885, #34235, #7034, #20704, #17832, #18009, #17298, #11724, #31704, #28301, #14951, #9564, #25958, #20532, #31538, #28833, #4181, #15121, #26133, #1464, #928, #12445, #29007, #14421, #742, #22697, #33689, #18551, #4552, #21062, #16014, #23970, #4357, #21423, #15483, #26500, #12984, #7926, #29376, #18908, #4722, #32068, #24325, #21250 ),
 ( #1836, #12811, #34965, #15303, #15657, #26316, #23789, #29204, #18193, #34773, #10465, #32245, #4890, #29556, #10289, #7571, #1653, #32419, #23608, #7743, #18375, #12630, #18725, #7403, #10095, #34601, #26679, #9917, #35316, #29727, #15832, #20879, #26853, #2011, #2205, #13174, #24148, #35141, #31880, #5071, #27031, #2375, #13346, #10636, #21594, #32594, #7211, #33975, #5, #11162, #14683, #22971, #10822, #20081, #19080, #21779, #27208, #19249, #174, #32773, #1031, #2551, #5594, #8097, #12006, #3556, #25515, #2903, #8934, #25697, #2730, #28386, #33601, #6247, #6417, #30255, #16555, #27382, #28215, #17385, #3729 ),
 ( #5247, #35489, #30078, #9302, #16188, #31090, #29905, #5419, #13517, #27565, #22132, #24498, #16367, #13694, #33796, #24676, #10990, #21956, #32950, #8273, #13864, #14502, #19898, #17208, #11813, #24849, #30911, #9121, #832, #22793, #6775, #34509, #12541, #1203, #18287, #28747, #17560, #15042, #26587, #9659, #25879, #4453, #34151, #29288, #9473, #4100, #31266, #12354, #9828, #12901, #31794, #7129, #1925, #23514, #4274, #34329, #31443, #26049, #31975, #20428, #34688, #20792, #23331, #28569, #29105, #17747, #4633, #12182, #10011, #23697, #3920, #23154, #14870, #20617, #20256, #1379, #31616, #15212, #6951, #17926, #28923 ),
 ( #15567, #26219, #1559, #18102, #15395, #26404, #1737, #12721, #20971, #7311, #23883, #34871, #6587, #4807, #5163, #21167, #19172, #26952, #35059, #10379, #35229, #4979, #26767, #21337, #32696, #2461, #35400, #27122, #2112, #7836, #30170, #18643, #29999, #13265, #24413, #16463, #5337, #10197, #7655, #32330, #13432, #7485, #8192, #29642, #13088, #10727, #16105, #18824, #21696, #2827, #2294, #8017, #5507, #19000, #27481, #13786, #24074, #16279, #10548, #24238, #24771, #27295, #2639, #15934, #29826, #13602, #32156, #24597, #15750, #32502, #21505, #35588, #18463, #10912, #21877, #32869, #29464, #33048, #24944, #11432, #20041 ),
 ( #8361, #30699, #30353, #33224, #16816, #25117, #33389, #22396, #31046, #8714, #16988, #19682, #446, #22571, #27826, #5853, #8894, #6028, #30522, #19517, #28173, #5686, #27995, #11085, #9079, #3162, #267, #11252, #3346, #14118, #16644, #22223, #33563, #14295, #25296, #617, #27656, #11598, #6377, #8546, #19856, #30869, #6205, #17341, #17167, #95, #3515, #14463, #25474, #19342, #33748, #794, #2994, #11774, #22752, #28344, #3691, #14642, #22054, #13954, #20928, #31581, #31927, #23661, #6547, #6912, #15001, #17708, #9969, #17884, #26179, #20386, #9615, #1514, #986, #28879, #31222, #12313, #28525, #20582, #18243 ),
 ( #31398, #22931, #14834, #1334, #33929, #6732, #7264, #26005, #17522, #9792, #3875, #34647, #25840, #34106, #11965, #28710, #15172, #29248, #12496, #23478, #4593, #4232, #34473, #4058, #1162, #23285, #1698, #12137, #4407, #20754, #34284, #9259, #31752, #23107, #25654, #9429, #15352, #29059, #20211, #7084, #18059, #26364, #12684, #29953, #18953, #21294, #2063, #29780, #7791, #32115, #13560, #24026, #24551, #5120, #15710, #32291, #27254, #35188, #15529, #32649, #26726, #13038, #24194, #19127, #4940, #30125, #35013, #4767, #29421, #10333, #21647, #32464, #16059, #27078, #10504, #21468, #26550, #7973, #34824, #5294, #29601 ),
 ( #7611, #1884, #18602, #21116, #10869, #16233, #2419, #10146, #18777, #15888, #26908, #2251, #13219, #13388, #12859, #24369, #35357, #10686, #2595, #35543, #21830, #32826, #8145, #23837, #7445, #18422, #25434, #33697, #22006, #30822, #30307, #33003, #2784, #30485, #11395, #8315, #11731, #13746, #16773, #19296, #22704, #14255, #575, #14074, #19644, #752, #13912, #3474, #8677, #16942, #17126, #5816, #27785, #2953, #3301, #28130, #14427, #24899, #19994, #3121, #16415, #11041, #5644, #9035, #27435, #6161, #5463, #16604, #24726, #25070, #33350, #54, #27616, #224, #8850, #11208, #22178, #33181, #8509, #19483, #399 ) ),
 .UNSPECIFIED., .T., .F., .F. ) 
 B_SPLINE_SURFACE_WITH_KNOTS ( ( 4, 3, 4 ),
 ( 3, 2, 2, 2, 2, 2, 2, 2, 2, 2, 2, 2, 2, 2, 2, 2, 2, 2, 2, 2, 2, 2, 2, 2, 2, 2, 2, 2, 2, 2, 2, 2, 2, 2, 2, 2, 2, 2, 2, 2, 3 ),
 ( 0.000000000000000000, 0.5000000000000000000, 1.000000000000000000 ),
 ( 0.000000000000000000, 0.02500000000000000139, 0.05000000000000000278, 0.07499999999999999722, 0.1000000000000000056, 0.1250000000000000000, 0.1499999999999999944, 0.1749999999999999889, 0.2000000000000000111, 0.2250000000000000056, 0.2500000000000000000, 0.2750000000000000222, 0.2999999999999999889, 0.3250000000000000111, 0.3499999999999999778, 0.3750000000000000000, 0.4000000000000000222, 0.4249999999999999889, 0.4500000000000000111, 0.4749999999999999778, 0.5000000000000000000, 0.5250000000000000222, 0.5500000000000000444, 0.5749999999999999556, 0.5999999999999999778, 0.6250000000000000000, 0.6500000000000000222, 0.6750000000000000444, 0.6999999999999999556, 0.7249999999999999778, 0.7500000000000000000, 0.7750000000000000222, 0.8000000000000000444, 0.8249999999999999556, 0.8499999999999999778, 0.8750000000000000000, 0.9000000000000000222, 0.9250000000000000444, 0.9499999999999999556, 0.9749999999999999778, 1.000000000000000000 ),
 .UNSPECIFIED. ) 
 GEOMETRIC_REPRESENTATION_ITEM ( )  RATIONAL_B_SPLINE_SURFACE ( (
 ( 1.000000000000000000, 0.9238795325112867385, 1.000000000000000000, 0.9238795325112867385, 1.000000000000000000, 0.9238795325112867385, 1.000000000000000000, 0.9238795325112867385, 1.000000000000000000, 0.9238795325112867385, 1.000000000000000000, 0.9238795325112867385, 1.000000000000000000, 0.9238795325112867385, 1.000000000000000000, 0.9238795325112867385, 1.000000000000000000, 0.9238795325112867385, 1.000000000000000000, 0.9238795325112867385, 1.000000000000000000, 0.9238795325112867385, 1.000000000000000000, 0.9238795325112867385, 1.000000000000000000, 0.9238795325112867385, 1.000000000000000000, 0.9238795325112867385, 1.000000000000000000, 0.9238795325112867385, 1.000000000000000000, 0.9238795325112867385, 1.000000000000000000, 0.9238795325112867385, 1.000000000000000000, 0.9238795325112867385, 1.000000000000000000, 0.9238795325112867385, 1.000000000000000000, 0.9238795325112867385, 1.000000000000000000, 0.9238795325112867385, 1.000000000000000000, 0.9238795325112867385, 1.000000000000000000, 0.9238795325112867385, 1.000000000000000000, 0.9238795325112867385, 1.000000000000000000, 0.9238795325112867385, 1.000000000000000000, 0.9238795325112867385, 1.000000000000000000, 0.9238795325112867385, 1.000000000000000000, 0.9238795325112867385, 1.000000000000000000, 0.9238795325112867385, 1.000000000000000000, 0.9238795325112867385, 1.000000000000000000, 0.9238795325112867385, 1.000000000000000000, 0.9238795325112867385, 1.000000000000000000, 0.9238795325112867385, 1.000000000000000000, 0.9238795325112867385, 1.000000000000000000, 0.9238795325112867385, 1.000000000000000000, 0.9238795325112867385, 1.000000000000000000, 0.9238795325112867385, 1.000000000000000000, 0.9238795325112867385, 1.000000000000000000, 0.9238795325112867385, 1.000000000000000000, 0.9238795325112867385, 1.000000000000000000),
 ( 0.3333333333333333703, 0.3079598441704289313, 0.3333333333333333703, 0.3079598441704289313, 0.3333333333333333703, 0.3079598441704289313, 0.3333333333333333703, 0.3079598441704289313, 0.3333333333333333703, 0.3079598441704289313, 0.3333333333333333703, 0.3079598441704289313, 0.3333333333333333703, 0.3079598441704289313, 0.3333333333333333703, 0.3079598441704289313, 0.3333333333333333703, 0.3079598441704289313, 0.3333333333333333703, 0.3079598441704289313, 0.3333333333333333703, 0.3079598441704289313, 0.3333333333333333703, 0.3079598441704289313, 0.3333333333333333703, 0.3079598441704289313, 0.3333333333333333703, 0.3079598441704289313, 0.3333333333333333703, 0.3079598441704289313, 0.3333333333333333703, 0.3079598441704289313, 0.3333333333333333703, 0.3079598441704289313, 0.3333333333333333703, 0.3079598441704289313, 0.3333333333333333703, 0.3079598441704289313, 0.3333333333333333703, 0.3079598441704289313, 0.3333333333333333703, 0.3079598441704289313, 0.3333333333333333703, 0.3079598441704289313, 0.3333333333333333703, 0.3079598441704289313, 0.3333333333333333703, 0.3079598441704289313, 0.3333333333333333703, 0.3079598441704289313, 0.3333333333333333703, 0.3079598441704289313, 0.3333333333333333703, 0.3079598441704289313, 0.3333333333333333703, 0.3079598441704289313, 0.3333333333333333703, 0.3079598441704289313, 0.3333333333333333703, 0.3079598441704289313, 0.3333333333333333703, 0.3079598441704289313, 0.3333333333333333703, 0.3079598441704289313, 0.3333333333333333703, 0.3079598441704289313, 0.3333333333333333703, 0.3079598441704289313, 0.3333333333333333703, 0.3079598441704289313, 0.3333333333333333703, 0.3079598441704289313, 0.3333333333333333703, 0.3079598441704289313, 0.3333333333333333703, 0.3079598441704289313, 0.3333333333333333703, 0.3079598441704289313, 0.3333333333333333703, 0.3079598441704289313, 0.3333333333333333703),
 ( 0.3333333333333333703, 0.3079598441704289313, 0.3333333333333333703, 0.3079598441704289313, 0.3333333333333333703, 0.3079598441704289313, 0.3333333333333333703, 0.3079598441704289313, 0.3333333333333333703, 0.3079598441704289313, 0.3333333333333333703, 0.3079598441704289313, 0.3333333333333333703, 0.3079598441704289313, 0.3333333333333333703, 0.3079598441704289313, 0.3333333333333333703, 0.3079598441704289313, 0.3333333333333333703, 0.3079598441704289313, 0.3333333333333333703, 0.3079598441704289313, 0.3333333333333333703, 0.3079598441704289313, 0.3333333333333333703, 0.3079598441704289313, 0.3333333333333333703, 0.3079598441704289313, 0.3333333333333333703, 0.3079598441704289313, 0.3333333333333333703, 0.3079598441704289313, 0.3333333333333333703, 0.3079598441704289313, 0.3333333333333333703, 0.3079598441704289313, 0.3333333333333333703, 0.3079598441704289313, 0.3333333333333333703, 0.3079598441704289313, 0.3333333333333333703, 0.3079598441704289313, 0.3333333333333333703, 0.3079598441704289313, 0.3333333333333333703, 0.3079598441704289313, 0.3333333333333333703, 0.3079598441704289313, 0.3333333333333333703, 0.3079598441704289313, 0.3333333333333333703, 0.3079598441704289313, 0.3333333333333333703, 0.3079598441704289313, 0.3333333333333333703, 0.3079598441704289313, 0.3333333333333333703, 0.3079598441704289313, 0.3333333333333333703, 0.3079598441704289313, 0.3333333333333333703, 0.3079598441704289313, 0.3333333333333333703, 0.3079598441704289313, 0.3333333333333333703, 0.3079598441704289313, 0.3333333333333333703, 0.3079598441704289313, 0.3333333333333333703, 0.3079598441704289313, 0.3333333333333333703, 0.3079598441704289313, 0.3333333333333333703, 0.3079598441704289313, 0.3333333333333333703, 0.3079598441704289313, 0.3333333333333333703, 0.3079598441704289313, 0.3333333333333333703, 0.3079598441704289313, 0.3333333333333333703),
 ( 1.000000000000000000, 0.9238795325112867385, 1.000000000000000000, 0.9238795325112867385, 1.000000000000000000, 0.9238795325112867385, 1.000000000000000000, 0.9238795325112867385, 1.000000000000000000, 0.9238795325112867385, 1.000000000000000000, 0.9238795325112867385, 1.000000000000000000, 0.9238795325112867385, 1.000000000000000000, 0.9238795325112867385, 1.000000000000000000, 0.9238795325112867385, 1.000000000000000000, 0.9238795325112867385, 1.000000000000000000, 0.9238795325112867385, 1.000000000000000000, 0.9238795325112867385, 1.000000000000000000, 0.9238795325112867385, 1.000000000000000000, 0.9238795325112867385, 1.000000000000000000, 0.9238795325112867385, 1.000000000000000000, 0.9238795325112867385, 1.000000000000000000, 0.9238795325112867385, 1.000000000000000000, 0.9238795325112867385, 1.000000000000000000, 0.9238795325112867385, 1.000000000000000000, 0.9238795325112867385, 1.000000000000000000, 0.9238795325112867385, 1.000000000000000000, 0.9238795325112867385, 1.000000000000000000, 0.9238795325112867385, 1.000000000000000000, 0.9238795325112867385, 1.000000000000000000, 0.9238795325112867385, 1.000000000000000000, 0.9238795325112867385, 1.000000000000000000, 0.9238795325112867385, 1.000000000000000000, 0.9238795325112867385, 1.000000000000000000, 0.9238795325112867385, 1.000000000000000000, 0.9238795325112867385, 1.000000000000000000, 0.9238795325112867385, 1.000000000000000000, 0.9238795325112867385, 1.000000000000000000, 0.9238795325112867385, 1.000000000000000000, 0.9238795325112867385, 1.000000000000000000, 0.9238795325112867385, 1.000000000000000000, 0.9238795325112867385, 1.000000000000000000, 0.9238795325112867385, 1.000000000000000000, 0.9238795325112867385, 1.000000000000000000, 0.9238795325112867385, 1.000000000000000000, 0.9238795325112867385, 1.000000000000000000),
 ( 0.3333333333333333703, 0.3079598441704289313, 0.3333333333333333703, 0.3079598441704289313, 0.3333333333333333703, 0.3079598441704289313, 0.3333333333333333703, 0.3079598441704289313, 0.3333333333333333703, 0.3079598441704289313, 0.3333333333333333703, 0.3079598441704289313, 0.3333333333333333703, 0.3079598441704289313, 0.3333333333333333703, 0.3079598441704289313, 0.3333333333333333703, 0.3079598441704289313, 0.3333333333333333703, 0.3079598441704289313, 0.3333333333333333703, 0.3079598441704289313, 0.3333333333333333703, 0.3079598441704289313, 0.3333333333333333703, 0.3079598441704289313, 0.3333333333333333703, 0.3079598441704289313, 0.3333333333333333703, 0.3079598441704289313, 0.3333333333333333703, 0.3079598441704289313, 0.3333333333333333703, 0.3079598441704289313, 0.3333333333333333703, 0.3079598441704289313, 0.3333333333333333703, 0.3079598441704289313, 0.3333333333333333703, 0.3079598441704289313, 0.3333333333333333703, 0.3079598441704289313, 0.3333333333333333703, 0.3079598441704289313, 0.3333333333333333703, 0.3079598441704289313, 0.3333333333333333703, 0.3079598441704289313, 0.3333333333333333703, 0.3079598441704289313, 0.3333333333333333703, 0.3079598441704289313, 0.3333333333333333703, 0.3079598441704289313, 0.3333333333333333703, 0.3079598441704289313, 0.3333333333333333703, 0.3079598441704289313, 0.3333333333333333703, 0.3079598441704289313, 0.3333333333333333703, 0.3079598441704289313, 0.3333333333333333703, 0.3079598441704289313, 0.3333333333333333703, 0.3079598441704289313, 0.3333333333333333703, 0.3079598441704289313, 0.3333333333333333703, 0.3079598441704289313, 0.3333333333333333703, 0.3079598441704289313, 0.3333333333333333703, 0.3079598441704289313, 0.3333333333333333703, 0.3079598441704289313, 0.3333333333333333703, 0.3079598441704289313, 0.3333333333333333703, 0.3079598441704289313, 0.3333333333333333703),
 ( 0.3333333333333333703, 0.3079598441704289313, 0.3333333333333333703, 0.3079598441704289313, 0.3333333333333333703, 0.3079598441704289313, 0.3333333333333333703, 0.3079598441704289313, 0.3333333333333333703, 0.3079598441704289313, 0.3333333333333333703, 0.3079598441704289313, 0.3333333333333333703, 0.3079598441704289313, 0.3333333333333333703, 0.3079598441704289313, 0.3333333333333333703, 0.3079598441704289313, 0.3333333333333333703, 0.3079598441704289313, 0.3333333333333333703, 0.3079598441704289313, 0.3333333333333333703, 0.3079598441704289313, 0.3333333333333333703, 0.3079598441704289313, 0.3333333333333333703, 0.3079598441704289313, 0.3333333333333333703, 0.3079598441704289313, 0.3333333333333333703, 0.3079598441704289313, 0.3333333333333333703, 0.3079598441704289313, 0.3333333333333333703, 0.3079598441704289313, 0.3333333333333333703, 0.3079598441704289313, 0.3333333333333333703, 0.3079598441704289313, 0.3333333333333333703, 0.3079598441704289313, 0.3333333333333333703, 0.3079598441704289313, 0.3333333333333333703, 0.3079598441704289313, 0.3333333333333333703, 0.3079598441704289313, 0.3333333333333333703, 0.3079598441704289313, 0.3333333333333333703, 0.3079598441704289313, 0.3333333333333333703, 0.3079598441704289313, 0.3333333333333333703, 0.3079598441704289313, 0.3333333333333333703, 0.3079598441704289313, 0.3333333333333333703, 0.3079598441704289313, 0.3333333333333333703, 0.3079598441704289313, 0.3333333333333333703, 0.3079598441704289313, 0.3333333333333333703, 0.3079598441704289313, 0.3333333333333333703, 0.3079598441704289313, 0.3333333333333333703, 0.3079598441704289313, 0.3333333333333333703, 0.3079598441704289313, 0.3333333333333333703, 0.3079598441704289313, 0.3333333333333333703, 0.3079598441704289313, 0.3333333333333333703, 0.3079598441704289313, 0.3333333333333333703, 0.3079598441704289313, 0.3333333333333333703),
 ( 1.000000000000000000, 0.9238795325112867385, 1.000000000000000000, 0.9238795325112867385, 1.000000000000000000, 0.9238795325112867385, 1.000000000000000000, 0.9238795325112867385, 1.000000000000000000, 0.9238795325112867385, 1.000000000000000000, 0.9238795325112867385, 1.000000000000000000, 0.9238795325112867385, 1.000000000000000000, 0.9238795325112867385, 1.000000000000000000, 0.9238795325112867385, 1.000000000000000000, 0.9238795325112867385, 1.000000000000000000, 0.9238795325112867385, 1.000000000000000000, 0.9238795325112867385, 1.000000000000000000, 0.9238795325112867385, 1.000000000000000000, 0.9238795325112867385, 1.000000000000000000, 0.9238795325112867385, 1.000000000000000000, 0.9238795325112867385, 1.000000000000000000, 0.9238795325112867385, 1.000000000000000000, 0.9238795325112867385, 1.000000000000000000, 0.9238795325112867385, 1.000000000000000000, 0.9238795325112867385, 1.000000000000000000, 0.9238795325112867385, 1.000000000000000000, 0.9238795325112867385, 1.000000000000000000, 0.9238795325112867385, 1.000000000000000000, 0.9238795325112867385, 1.000000000000000000, 0.9238795325112867385, 1.000000000000000000, 0.9238795325112867385, 1.000000000000000000, 0.9238795325112867385, 1.000000000000000000, 0.9238795325112867385, 1.000000000000000000, 0.9238795325112867385, 1.000000000000000000, 0.9238795325112867385, 1.000000000000000000, 0.9238795325112867385, 1.000000000000000000, 0.9238795325112867385, 1.000000000000000000, 0.9238795325112867385, 1.000000000000000000, 0.9238795325112867385, 1.000000000000000000, 0.9238795325112867385, 1.000000000000000000, 0.9238795325112867385, 1.000000000000000000, 0.9238795325112867385, 1.000000000000000000, 0.9238795325112867385, 1.000000000000000000, 0.9238795325112867385, 1.000000000000000000, 0.9238795325112867385, 1.000000000000000000) ) ) 
 REPRESENTATION_ITEM ( '' )  SURFACE ( )  );
#12830=CARTESIAN_POINT ( 'NONE',  ( -37.62959469683911351, -113.9929510916434339, 13.10254527216511633 ) ) ;
#12832=CARTESIAN_POINT ( 'NONE',  ( -36.06250000000000711, -115.9929510916434481, 13.11852480586264846 ) ) ;
#12846=CARTESIAN_POINT ( 'NONE',  ( -35.50000000000000711, -112.0140978167138712, 0.3752176474015640473 ) ) ;
#12851=CARTESIAN_POINT ( 'NONE',  ( -35.50000000000000711, -114.1091535596544873, 9.513028657562415447 ) ) ;
#12855=CARTESIAN_POINT ( 'NONE',  ( -34.50000000000000000, -111.0780159515033034, -1.143161139953928762 ) ) ;
#12859=CARTESIAN_POINT ( 'NONE',  ( -35.54388159064475872, -112.6276912846090568, 2.816024454178448710 ) ) ;
#12865=CARTESIAN_POINT ( 'NONE',  ( -35.50000000000000000, -115.0140978167138712, -0.6247823525984403936 ) ) ;
#12870=CARTESIAN_POINT ( 'NONE',  ( -37.51635661748575501, -114.9929510916434339, 13.11827392651459157 ) ) ;
#12874=CARTESIAN_POINT ( 'NONE',  ( -37.37500000000009237, -114.9929510916434339, 14.11852480586264846 ) ) ;
#12879=CARTESIAN_POINT ( 'NONE',  ( -36.62499999999902656, -115.9929510916434481, 13.11852480586264846 ) ) ;
#12880=CARTESIAN_POINT ( 'NONE',  ( -35.50000000000000711, -115.8878449012421754, -1.128496220799388494 ) ) ;
#12890=VERTEX_POINT ( 'NONE', #14360 ) ;
#12891=CARTESIAN_POINT ( 'NONE',  ( -37.66520193420439000, -113.2509883718312977, 3.941024454178448710 ) ) ;
#12901=CARTESIAN_POINT ( 'NONE',  ( -33.97545270896703329, -115.1833782841879810, 7.090225545821551734 ) ) ;
#12917=CARTESIAN_POINT ( 'NONE',  ( -34.50000000000000000, -115.9929510916434481, 12.44250253426871033 ) ) ;
#12920=CARTESIAN_POINT ( 'NONE',  ( -38.99999999999999289, -113.9407375970686900, 8.253524454178448266 ) ) ;
#12921=CARTESIAN_POINT ( 'NONE',  ( -34.50000000000000000, -115.3279708130221479, 8.997521329298534098 ) ) ;
#12931=CARTESIAN_POINT ( 'NONE',  ( -35.00000000000000000, -113.9407375970686900, 5.496475545821551734 ) ) ;
#12933=CARTESIAN_POINT ( 'NONE',  ( -35.50000000000000000, -113.0140978167138712, 0.8752176474015934682 ) ) ;
#12944=CARTESIAN_POINT ( 'NONE',  ( -35.02454729103298092, -113.1123104723225055, 9.902725545821553510 ) ) ;
#12950=CARTESIAN_POINT ( 'NONE',  ( -35.50000000000000711, -112.0140978167138712, 0.2502176474015765373 ) ) ;
#12957=CARTESIAN_POINT ( 'NONE',  ( -34.50000000000000000, -112.6043641208289188, 1.789429170677330649 ) ) ;
#12959=CARTESIAN_POINT ( 'NONE',  ( -34.50000000000000000, -114.9929510916434339, 10.68227981832981044 ) ) ;
#12960=EDGE_CURVE ( 'NONE', #18157, #18380, #21881, .T. ) ;
#12962=CARTESIAN_POINT ( 'NONE',  ( -37.66108410722335265, -114.9929510916434339, 13.09299768411426790 ) ) ;
#12964=CARTESIAN_POINT ( 'NONE',  ( -34.50000000000000000, -114.1712995509219724, 9.522174004479579068 ) ) ;
#12966=CARTESIAN_POINT ( 'NONE',  ( -37.99994980024369085, -114.9929510916434339, 12.62670525340494621 ) ) ;
#12973=CARTESIAN_POINT ( 'NONE',  ( -37.50818044754229419, -114.9929510916434339, 13.11847460610629668 ) ) ;
#12976=CARTESIAN_POINT ( 'NONE',  ( -38.37230871539094323, -112.5438815906447729, 6.941024454178449155 ) ) ;
#12984=CARTESIAN_POINT ( 'NONE',  ( -38.97545270896704039, -113.1123104723225197, 8.347274454178448266 ) ) ;
#12996=CARTESIAN_POINT ( 'NONE',  ( -34.50000000000000000, -113.2224311500466030, -2.624782352598442614 ) ) ;
#13001=CARTESIAN_POINT ( 'NONE',  ( -35.50000000000000711, -114.8847986568751907, 10.03799953695244618 ) ) ;
#13007=CARTESIAN_POINT ( 'NONE',  ( -34.50000000000000000, -113.9929510916434339, 10.50625754673577994 ) ) ;
#13012=CARTESIAN_POINT ( 'NONE',  ( -34.50000000000000000, -113.9813390189866027, 10.50487145766371100 ) ) ;
#13014=CARTESIAN_POINT ( 'NONE',  ( -38.00000000000000711, -115.9929510916434481, 12.59102132592609102 ) ) ;
#13026=CARTESIAN_POINT ( 'NONE',  ( -35.50000000000000711, -114.5974311500472425, -1.624782352598427959 ) ) ;
#13028=CARTESIAN_POINT ( 'NONE',  ( -35.50000000000000711, -114.9492820284331742, 10.20776876943783940 ) ) ;
#13033=CARTESIAN_POINT ( 'NONE',  ( -35.50000000000000000, -111.0168437565048691, 0.9961850632443862708 ) ) ;
#13038=CARTESIAN_POINT ( 'NONE',  ( -36.52652403469556930, -113.0245472910329880, 7.222274454178449155 ) ) ;
#13045=CARTESIAN_POINT ( 'NONE',  ( -34.50000000000000000, -113.0140978167137717, 0.8903425666012282358 ) ) ;
#13053=CARTESIAN_POINT ( 'NONE',  ( -37.99994980024369085, -114.9929510916434339, 12.62670525340494621 ) ) ;
#13058=CARTESIAN_POINT ( 'NONE',  ( -34.50000000000000000, -112.0140978167138712, -0.3122823525984337878 ) ) ;
#13066=CARTESIAN_POINT ( 'NONE',  ( -37.34375000000001421, -115.9929510916434481, 13.11852480586264846 ) ) ;
#13067=CARTESIAN_POINT ( 'NONE',  ( -35.50000000000000711, -116.0060826362711595, -0.7553032835231661135 ) ) ;
#13077=CARTESIAN_POINT ( 'NONE',  ( -36.64504884055823908, -115.0245472910329880, 3.284774454178449155 ) ) ;
#13088=CARTESIAN_POINT ( 'NONE',  ( -37.05926240293131713, -112.0000000000000142, 6.621475545821550845 ) ) ;
#13113=CARTESIAN_POINT ( 'NONE',  ( -34.97545270896703329, -113.2308352781851397, 5.909774454178449155 ) ) ;
#13114=CARTESIAN_POINT ( 'NONE',  ( -34.50300906734826611, -115.9929510916434481, 12.71660600561482468 ) ) ;
#13124=CARTESIAN_POINT ( 'NONE',  ( -38.37230871539094323, -115.4561184093552413, 6.058975545821551734 ) ) ;
#13142=CARTESIAN_POINT ( 'NONE',  ( -35.50000000000000711, -113.2637153405686519, 1.912112492696748989 ) ) ;
#13151=CARTESIAN_POINT ( 'NONE',  ( -35.07817881376918479, -114.9929510916434339, 13.81802396319203297 ) ) ;
#13153=CARTESIAN_POINT ( 'NONE',  ( -37.99959864031215773, -114.9929510916434339, 12.63896776382213538 ) ) ;
#13155=CARTESIAN_POINT ( 'NONE',  ( -34.50000000000000000, -114.1489256397697289, 9.518467544735724317 ) ) ;
#13163=CARTESIAN_POINT ( 'NONE',  ( -38.00000000000000711, -114.9929510916434339, 12.60752341388803721 ) ) ;
#13166=CARTESIAN_POINT ( 'NONE',  ( -38.45611840935523418, -115.3723087153909432, 5.066024454178449155 ) ) ;
#13174=CARTESIAN_POINT ( 'NONE',  ( -35.81662171581204746, -117.0245472910329738, 4.784774454178448266 ) ) ;
#13177=CARTESIAN_POINT ( 'NONE',  ( -35.50000000000000711, -116.0140978167138712, 0.3752176474015736507 ) ) ;
#13185=CARTESIAN_POINT ( 'NONE',  ( -34.50000000000000000, -112.6882700046066645, -2.599147725882136939 ) ) ;
#13190=CARTESIAN_POINT ( 'NONE',  ( -35.50000000000000711, -114.1068310684433129, 9.512752019463897923 ) ) ;
#13192=CARTESIAN_POINT ( 'NONE',  ( -38.00000000000000711, -113.9929510916434339, 10.50625754673587053 ) ) ;
#13195=CARTESIAN_POINT ( 'NONE',  ( -37.93687354226506869, -113.9929510916434339, 12.87038173996323565 ) ) ;
#13196=CARTESIAN_POINT ( 'NONE',  ( -36.31249999999994316, -115.9929510916434481, 13.11852480586264846 ) ) ;
#13206=CARTESIAN_POINT ( 'NONE',  ( -35.50000000000000000, -113.0140978167140702, 0.8752176474015603835 ) ) ;
#13209=CARTESIAN_POINT ( 'NONE',  ( -35.50400759022159036, -114.9929510916434339, 12.68378527132497524 ) ) ;
#13215=CARTESIAN_POINT ( 'NONE',  ( -35.50000000000000000, -112.7319952733504635, 2.855726801009121463 ) ) ;
#13219=CARTESIAN_POINT ( 'NONE',  ( -36.94073759706868287, -112.0000000000000142, 2.628524454178448710 ) ) ;
#13226=CARTESIAN_POINT ( 'NONE',  ( -34.50000000000000000, -113.0140978167138712, 0.5627176474015715968 ) ) ;
#13231=CARTESIAN_POINT ( 'NONE',  ( -37.52044295795950291, -114.9929510916434339, 13.11812344617477244 ) ) ;
#13234=CARTESIAN_POINT ( 'NONE',  ( -34.50000000000000000, -112.0140978167138712, 0.3752176474015640473 ) ) ;
#13241=CARTESIAN_POINT ( 'NONE',  ( -37.99899697755054717, -115.9929510916434481, 12.65121853911336913 ) ) ;
#13265=CARTESIAN_POINT ( 'NONE',  ( -34.97545270896703329, -114.7691647218148745, 5.590225545821552622 ) ) ;
#13275=EDGE_LOOP ( 'NONE', ( #10189, #8134 ) ) ;
#13283=CARTESIAN_POINT ( 'NONE',  ( -38.37230871539094323, -112.5438815906447729, 5.441024454178449155 ) ) ;
#13284=CARTESIAN_POINT ( 'NONE',  ( -34.50000000000000000, -115.9056129652226872, 9.909279992139808257 ) ) ;
#13296=CARTESIAN_POINT ( 'NONE',  ( -38.99999999999999289, -114.0592624029313242, 3.246475545821551734 ) ) ;
#13314=CARTESIAN_POINT ( 'NONE',  ( -35.50000000000000711, -112.2144317118258527, -1.239329810084414341 ) ) ;
#13320=CARTESIAN_POINT ( 'NONE',  ( -34.50000000000000000, -116.0124910254613297, -0.6902086197697608894 ) ) ;
#13321=CARTESIAN_POINT ( 'NONE',  ( -35.93867112612154813, -114.9929510916434339, 14.11732072679899197 ) ) ;
#13323=CARTESIAN_POINT ( 'NONE',  ( -35.50000000000000000, -113.9929510916434339, 10.55026311463432087 ) ) ;
#13325=CARTESIAN_POINT ( 'NONE',  ( -34.50000000000000000, -114.1021862393805577, 9.512197583835053649 ) ) ;
#13328=CARTESIAN_POINT ( 'NONE',  ( -38.00000000000000711, -114.9929510916434339, 12.57451923796417503 ) ) ;
#13335=CARTESIAN_POINT ( 'NONE',  ( -38.00000000000000711, -114.9929510916434339, 12.26648026267477043 ) ) ;
#13337=CARTESIAN_POINT ( 'NONE',  ( -35.02454729103298803, -114.8876895276775087, 4.597274454178448266 ) ) ;
#13346=CARTESIAN_POINT ( 'NONE',  ( -39.07941549657748936, -111.8367748094582055, 5.441024454178449155 ) ) ;
#13356=CARTESIAN_POINT ( 'NONE',  ( -34.50000000000000000, -112.1946304249441795, 2.703640693953100804 ) ) ;
#13359=CARTESIAN_POINT ( 'NONE',  ( -35.50000000000000711, -114.0000000000003411, 9.500000000000035527 ) ) ;
#13360=CARTESIAN_POINT ( 'NONE',  ( -38.00000000000000711, -113.9929510916434339, 12.59652202191340820 ) ) ;
#13364=CARTESIAN_POINT ( 'NONE',  ( -37.66108410722335265, -113.9929510916434339, 13.09299768411426612 ) ) ;
#13365=CARTESIAN_POINT ( 'NONE',  ( -37.51635661748575501, -115.9929510916434481, 13.11827392651459512 ) ) ;
#13377=CARTESIAN_POINT ( 'NONE',  ( -35.50000000000000000, -113.0140978167138712, -0.3122823525984338988 ) ) ;
#13380=CARTESIAN_POINT ( 'NONE',  ( -35.50000000000000711, -114.9929510916434339, 10.52826033068511435 ) ) ;
#13384=CARTESIAN_POINT ( 'NONE',  ( -35.50000000000000000, -111.1014359431343905, 1.472195201997948510 ) ) ;
#13388=CARTESIAN_POINT ( 'NONE',  ( -36.11231047232249125, -112.0245472910329880, 2.722274454178448266 ) ) ;
#13393=CARTESIAN_POINT ( 'NONE',  ( -34.50000000000000000, -113.0140978167138712, 0.7189676474015717078 ) ) ;
#13398=CARTESIAN_POINT ( 'NONE',  ( -37.46093750000000711, -114.9929510916434339, 13.11852480586264669 ) ) ;
#13402=CARTESIAN_POINT ( 'NONE',  ( -34.50000000000000000, -115.1770117227680998, -1.611965039240062181 ) ) ;
#13405=ADVANCED_FACE ( 'NONE', ( #30717 ), #6051, .F. ) ;
#13410=CARTESIAN_POINT ( 'NONE',  ( -38.00000000000000711, -115.9929510916434481, 10.85830208992306822 ) ) ;
#13432=CARTESIAN_POINT ( 'NONE',  ( -38.99999999999999289, -114.0592624029313242, 6.246475545821550845 ) ) ;
#13451=CARTESIAN_POINT ( 'NONE',  ( -35.62769128460905677, -115.4561184093552413, 6.191024454178448266 ) ) ;
#13453=CARTESIAN_POINT ( 'NONE',  ( -37.74437085908086686, -115.9929510916434481, 14.09929883582536903 ) ) ;
#13463=CARTESIAN_POINT ( 'NONE',  ( -34.00000000000000000, -113.9407375970686758, 8.496475545821549957 ) ) ;
#13481=CARTESIAN_POINT ( 'NONE',  ( -35.50000000000000711, -112.0140978167138712, -0.4997823525984337878 ) ) ;
#13490=CARTESIAN_POINT ( 'NONE',  ( -34.50000000000000000, -112.8511839106603247, -1.611965039240275122 ) ) ;
#13491=CARTESIAN_POINT ( 'NONE',  ( -38.92341863475394348, -114.9929510916434339, 13.10177712753322155 ) ) ;
#13494=CARTESIAN_POINT ( 'NONE',  ( -35.50000000000000000, -113.9697269463297431, 10.50348536859153370 ) ) ;
#13497=CARTESIAN_POINT ( 'NONE',  ( -34.50000000000000000, -114.9929510916434339, 12.50851088611648088 ) ) ;
#13505=CARTESIAN_POINT ( 'NONE',  ( -36.62499999999902656, -114.9929510916434339, 13.11852480586264669 ) ) ;
#13507=CARTESIAN_POINT ( 'NONE',  ( -39.02454729103295961, -114.7691647218148745, 6.659774454178450043 ) ) ;
#13517=CARTESIAN_POINT ( 'NONE',  ( -39.99999999999999289, -114.0592624029313242, 3.246475545821551734 ) ) ;
#13529=CARTESIAN_POINT ( 'NONE',  ( -34.50000000000000000, -114.1807644833817648, -2.624782352598442614 ) ) ;
#13533=CARTESIAN_POINT ( 'NONE',  ( -35.50000000000000711, -114.1264797827112574, 9.515205387299289441 ) ) ;
#13534=CARTESIAN_POINT ( 'NONE',  ( -35.80421860361284558, -113.9929510916434339, 14.10650203519841916 ) ) ;
#13538=CARTESIAN_POINT ( 'NONE',  ( -37.37500000000009237, -113.9929510916434339, 13.11852480586264846 ) ) ;
#13539=CARTESIAN_POINT ( 'NONE',  ( -35.50000000000000711, -114.9929510916434339, 10.59426868253284226 ) ) ;
#13550=CARTESIAN_POINT ( 'NONE',  ( -35.50000000000000000, -113.1291422947505936, 0.8889500704178361357 ) ) ;
#13552=CARTESIAN_POINT ( 'NONE',  ( -35.50000000000000711, -114.9929510916434339, 10.53376102667243508 ) ) ;
#13557=CARTESIAN_POINT ( 'NONE',  ( -35.50000000000000000, -111.0140978167138570, -0.3747823525984258497 ) ) ;
#13560=CARTESIAN_POINT ( 'NONE',  ( -36.33479806579561000, -114.7490116281687165, 6.191024454178448266 ) ) ;
#13567=CARTESIAN_POINT ( 'NONE',  ( -34.50000000000000000, -114.9932644833805426, -0.6247823525982824089 ) ) ;
#13572=CARTESIAN_POINT ( 'NONE',  ( -35.50000000000000000, -113.9929510916434339, 12.53051367006571581 ) ) ;
#13575=CARTESIAN_POINT ( 'NONE',  ( -34.50000000000000000, -112.1859307030124739, 1.448610958621386224 ) ) ;
#13576=CARTESIAN_POINT ( 'NONE',  ( -37.24999999999992184, -115.9929510916434481, 14.11852480586265024 ) ) ;
#13581=CARTESIAN_POINT ( 'NONE',  ( -38.00000000000000711, -115.9929510916434481, 12.39849696637031151 ) ) ;
#13602=CARTESIAN_POINT ( 'NONE',  ( -34.97545270896703329, -114.7691647218148745, 8.590225545821551734 ) ) ;
#13605=EDGE_LOOP ( 'NONE', ( #29645, #20097, #34772, #20753, #18818, #19520 ) ) ;
#13624=CARTESIAN_POINT ( 'NONE',  ( -38.99518666717493431, -115.9929510916434481, 12.74107470552714894 ) ) ;
#13634=CARTESIAN_POINT ( 'NONE',  ( -36.94073759706868287, -115.0000000000000000, 4.371475545821550845 ) ) ;
#13670=CARTESIAN_POINT ( 'NONE',  ( -34.50000000000000000, -116.0060826362711595, -0.7553032835231661135 ) ) ;
#13671=CARTESIAN_POINT ( 'NONE',  ( -38.99699093265173389, -114.9929510916434339, 12.71660600561481402 ) ) ;
#13672=CARTESIAN_POINT ( 'NONE',  ( -35.50000000000000000, -113.9929510916436470, 10.50625754673586876 ) ) ;
#13674=CARTESIAN_POINT ( 'NONE',  ( -34.50075263804418313, -114.9929510916434339, 12.66759465831979981 ) ) ;
#13685=CARTESIAN_POINT ( 'NONE',  ( -38.18337828418795965, -110.9754527089670546, 7.034774454178450043 ) ) ;
#13694=CARTESIAN_POINT ( 'NONE',  ( -35.81662171581203324, -110.9754527089670546, 3.715225545821552178 ) ) ;
#13710=CARTESIAN_POINT ( 'NONE',  ( -34.50000000000000000, -115.5324766040685631, -2.560864217809699195 ) ) ;
#13713=CARTESIAN_POINT ( 'NONE',  ( -35.50000000000000711, -114.9929510916434339, 11.21034663311131929 ) ) ;
#13715=CARTESIAN_POINT ( 'NONE',  ( -34.51922597003733273, -113.9929510916434339, 12.86289566494349224 ) ) ;
#13719=CARTESIAN_POINT ( 'NONE',  ( -34.50000000000000000, -113.9929510916434339, 12.39849696637031684 ) ) ;
#13720=CARTESIAN_POINT ( 'NONE',  ( -39.00000000000000711, -114.9929510916434339, 12.50851088611646311 ) ) ;
#13722=CARTESIAN_POINT ( 'NONE',  ( -38.00000000000000711, -115.9929510916434481, 10.50625754673587053 ) ) ;
#13735=CARTESIAN_POINT ( 'NONE',  ( -35.50000000000000000, -113.0140978167139991, 0.8595926474015699315 ) ) ;
#13738=CARTESIAN_POINT ( 'NONE',  ( -37.35495115944176092, -112.9754527089670688, 2.534774454178448710 ) ) ;
#13742=CARTESIAN_POINT ( 'NONE',  ( -35.50000000000000000, -112.6572589393539516, 2.844055607295835397 ) ) ;
#13746=CARTESIAN_POINT ( 'NONE',  ( -37.88768952767750164, -115.9754527089670262, 4.972274454178448266 ) ) ;
#13752=CARTESIAN_POINT ( 'NONE',  ( -34.50000000000000000, -115.0140978167138428, -0.6247823525979866455 ) ) ;
#13756=CARTESIAN_POINT ( 'NONE',  ( -35.50000000000000000, -113.9929510916434339, 10.50625754673588474 ) ) ;
#13759=CARTESIAN_POINT ( 'NONE',  ( -34.50000000000000000, -116.0140978167138712, -0.4997823525984418369 ) ) ;
#13760=CARTESIAN_POINT ( 'NONE',  ( -38.99518666717493431, -115.9929510916434481, 12.74107470552714894 ) ) ;
#13766=CARTESIAN_POINT ( 'NONE',  ( -38.00000000000000711, -115.9929510916434481, 12.44250253426875119 ) ) ;
#13786=CARTESIAN_POINT ( 'NONE',  ( -38.97545270896704039, -114.8876895276775087, 7.652725545821552622 ) ) ;
#13794=CARTESIAN_POINT ( 'NONE',  ( -35.50000000000000711, -114.1414532730574507, 9.517316564499758158 ) ) ;
#13803=CARTESIAN_POINT ( 'NONE',  ( -37.46093750000000711, -115.9929510916434481, 14.11852480586265024 ) ) ;
#13804=DIRECTION ( 'NONE',  ( 0.000000000000000000, 0.9929510916431029122, -0.1185248058626136303 ) ) ;
#13812=CARTESIAN_POINT ( 'NONE',  ( -37.66520193420439711, -114.7490116281687023, 4.558975545821549957 ) ) ;
#13838=CARTESIAN_POINT ( 'NONE',  ( -34.50000000000000000, -112.6919296022648638, -1.573728109100751116 ) ) ;
#13839=CARTESIAN_POINT ( 'NONE',  ( -39.00000206272865455, -114.9929510916434339, 12.61164896875035701 ) ) ;
#13840=CARTESIAN_POINT ( 'NONE',  ( -35.50000000000000000, -113.9929510916430075, 10.50625754673586876 ) ) ;
#13844=CARTESIAN_POINT ( 'NONE',  ( -34.50000000000000000, -114.9929510916434339, 12.60752341388803544 ) ) ;
#13854=CARTESIAN_POINT ( 'NONE',  ( -38.00000000000000711, -114.9929510916434339, 10.50625754673587231 ) ) ;
#13856=CARTESIAN_POINT ( 'NONE',  ( -36.94073759706866156, -111.0000000000000284, 7.128524454178450043 ) ) ;
#13864=CARTESIAN_POINT ( 'NONE',  ( -36.94073759706868287, -116.9999999999999858, 4.371475545821550845 ) ) ;
#13875=CARTESIAN_POINT ( 'NONE',  ( -34.50000000000000000, -117.0141134414687514, -0.5779076015960331603 ) ) ;
#13878=CARTESIAN_POINT ( 'NONE',  ( -37.50818044754229419, -114.9929510916434339, 13.11847460610629668 ) ) ;
#13880=CARTESIAN_POINT ( 'NONE',  ( -35.93867112612154102, -113.9929510916434339, 14.11732072679899197 ) ) ;
#13883=CARTESIAN_POINT ( 'NONE',  ( -34.50000000000000000, -113.9929510916434339, 10.50625754673588474 ) ) ;
#13884=CARTESIAN_POINT ( 'NONE',  ( -37.88878409051687868, -114.9929510916434339, 14.07058620477052102 ) ) ;
#13885=CARTESIAN_POINT ( 'NONE',  ( -35.50000000000000711, -114.4026847875275337, 9.592046023459676718 ) ) ;
#13900=CARTESIAN_POINT ( 'NONE',  ( -35.50000000000000000, -113.0140978167136581, 0.8752176474015604946 ) ) ;
#13902=CARTESIAN_POINT ( 'NONE',  ( -35.97545270896702618, -113.6450488405582604, 2.909774454178449155 ) ) ;
#13909=CARTESIAN_POINT ( 'NONE',  ( -35.50000000000000711, -112.9876085932806262, 1.879154677457530065 ) ) ;
#13912=CARTESIAN_POINT ( 'NONE',  ( -35.54388159064475872, -112.6276912846090568, 5.816024454178449155 ) ) ;
#13916=CARTESIAN_POINT ( 'NONE',  ( -34.50000000000000000, -112.0140978167138712, -0.4685323525984295134 ) ) ;
#13923=CARTESIAN_POINT ( 'NONE',  ( -35.50000000000000000, -113.9929510916435049, 10.50625754673586876 ) ) ;
#13927=CARTESIAN_POINT ( 'NONE',  ( -34.50000000000000000, -112.6572589393539516, 2.844055607295835397 ) ) ;
#13928=CARTESIAN_POINT ( 'NONE',  ( -39.00000000000000000, -115.9929510916434481, 11.21034663311206181 ) ) ;
#13935=CARTESIAN_POINT ( 'NONE',  ( -38.00000068757622529, -115.9929510916434481, 12.61439929482944855 ) ) ;
#13954=CARTESIAN_POINT ( 'NONE',  ( -37.47347596530441649, -113.0245472910329880, 8.027725545821551734 ) ) ;
#13964=CARTESIAN_POINT ( 'NONE',  ( -35.50000000000000711, -114.9492820284331742, 10.20776876943783940 ) ) ;
#13973=CARTESIAN_POINT ( 'NONE',  ( -39.00000000000000000, -115.9929510916434481, 12.56351784598954779 ) ) ;
#13974=CARTESIAN_POINT ( 'NONE',  ( -35.00000000000000000, -114.0000000000003411, 9.500000000000035527 ) ) ;
#13981=CARTESIAN_POINT ( 'NONE',  ( -35.00000000000000000, -113.9407375970686900, 8.496475545821551734 ) ) ;
#14005=CARTESIAN_POINT ( 'NONE',  ( -34.50000000000000000, -114.3474311500471430, -1.624782352598427959 ) ) ;
#14007=CARTESIAN_POINT ( 'NONE',  ( -37.62254989966454133, -114.9929510916434339, 14.11371147303758278 ) ) ;
#14008=CARTESIAN_POINT ( 'NONE',  ( -35.50000000000000000, -113.9917898843777522, 10.50611893782865813 ) ) ;
#14011=CARTESIAN_POINT ( 'NONE',  ( -36.15625000000007816, -114.9929510916434339, 14.11852480586264846 ) ) ;
#14021=CARTESIAN_POINT ( 'NONE',  ( -37.05926240293133134, -116.9999999999999858, 4.878524454178448266 ) ) ;
#14023=CARTESIAN_POINT ( 'NONE',  ( -35.50000000000000711, -112.8835768857893527, -1.616767172155725740 ) ) ;
#14038=CARTESIAN_POINT ( 'NONE',  ( -35.50000000000000000, -113.6974040292745656, 2.970979214817929481 ) ) ;
#14043=CARTESIAN_POINT ( 'NONE',  ( -36.15625000000007816, -114.9929510916434339, 13.11852480586264669 ) ) ;
#14044=CARTESIAN_POINT ( 'NONE',  ( -36.31249999999994316, -113.9929510916434339, 14.11852480586265024 ) ) ;
#14048=CARTESIAN_POINT ( 'NONE',  ( -34.50000000000000000, -113.9929510916434339, 12.26648026267477398 ) ) ;
#14049=CARTESIAN_POINT ( 'NONE',  ( -38.99699093265173389, -114.9929510916434339, 12.71660600561481402 ) ) ;
#14050=CARTESIAN_POINT ( 'NONE',  ( -35.50000000000000711, -114.9929510916434339, 10.85830208992344303 ) ) ;
#14063=CARTESIAN_POINT ( 'NONE',  ( -35.50000000000000000, -112.9977353549762000, -0.6247823525983134951 ) ) ;
#14065=CARTESIAN_POINT ( 'NONE',  ( -36.11231047232249125, -112.0245472910329880, 4.222274454178449155 ) ) ;
#14071=CARTESIAN_POINT ( 'NONE',  ( -35.50000000000000000, -117.0140814545088688, -0.6738694770610542673 ) ) ;
#14074=CARTESIAN_POINT ( 'NONE',  ( -37.76916472181487450, -111.9754527089670404, 5.534774454178449155 ) ) ;
#14079=CARTESIAN_POINT ( 'NONE',  ( -34.50000000000000000, -112.1222502514821144, 1.343475657184566296 ) ) ;
#14088=CARTESIAN_POINT ( 'NONE',  ( -35.50000000000000000, -113.9929510916434339, 10.94631322572069365 ) ) ;
#14092=CARTESIAN_POINT ( 'NONE',  ( -34.50000000000000000, -116.0140978167138712, 0.6252176474015648244 ) ) ;
#14094=CARTESIAN_POINT ( 'NONE',  ( -39.00000000000000000, -115.9929510916434481, 12.59102132592609102 ) ) ;
#14118=CARTESIAN_POINT ( 'NONE',  ( -36.64504884055821776, -112.9754527089670688, 5.215225545821552622 ) ) ;
#14128=CARTESIAN_POINT ( 'NONE',  ( -35.50000000000000711, -113.2224311500466030, -1.624782352598427959 ) ) ;
#14137=CARTESIAN_POINT ( 'NONE',  ( -34.50000000000000000, -114.8847986568751907, 10.03799953695244618 ) ) ;
#14141=CARTESIAN_POINT ( 'NONE',  ( -37.34375000000001421, -115.9929510916434481, 14.11852480586265024 ) ) ;
#14142=CARTESIAN_POINT ( 'NONE',  ( -35.50000000000000711, -112.0140978167138712, 0.7189676474015718188 ) ) ;
#14150=CARTESIAN_POINT ( 'NONE',  ( -35.02454729103298803, -113.1123104723225197, 9.902725545821557063 ) ) ;
#14185=CARTESIAN_POINT ( 'NONE',  ( -34.50000000000000000, -114.2600084737790809, 8.524153227862690585 ) ) ;
#14189=CARTESIAN_POINT ( 'NONE',  ( -34.50000000000000000, -114.9929510916434339, 11.21034663311131929 ) ) ;
#14200=CARTESIAN_POINT ( 'NONE',  ( -38.18337828418795965, -110.9754527089670546, 2.534774454178448710 ) ) ;
#14202=CARTESIAN_POINT ( 'NONE',  ( -35.50000000000000711, -112.2144317118258527, -1.239329810084414341 ) ) ;
#14213=ORIENTED_EDGE ( 'NONE', *, *, #9269, .T. ) ;
#14220=CARTESIAN_POINT ( 'NONE',  ( -34.50000000000000000, -116.9884631899972476, -0.9506101647064282290 ) ) ;
#14224=CARTESIAN_POINT ( 'NONE',  ( -37.24999999999992895, -114.9929510916434339, 13.11852480586264669 ) ) ;
#14225=CARTESIAN_POINT ( 'NONE',  ( -35.90191880024782023, -113.9929510916434339, 14.11551573851449071 ) ) ;
#14228=CARTESIAN_POINT ( 'NONE',  ( -34.50000000000000000, -113.9929510916434339, 10.52000928670414126 ) ) ;
#14229=CARTESIAN_POINT ( 'NONE',  ( -38.99879592093640923, -114.9929510916434339, 12.67985367974111455 ) ) ;
#14230=CARTESIAN_POINT ( 'NONE',  ( -35.50000000000000711, -114.9929517792218689, 10.50900788599415314 ) ) ;
#14244=CARTESIAN_POINT ( 'NONE',  ( -35.50000000000000000, -115.0140978167138428, -0.6247823525986679893 ) ) ;
#14246=CARTESIAN_POINT ( 'NONE',  ( -35.54388159064475872, -112.6276912846090568, 4.316024454178448266 ) ) ;
#14252=CARTESIAN_POINT ( 'NONE',  ( -35.50000000000000711, -113.2637153405686519, 1.912112492696748989 ) ) ;
#14255=CARTESIAN_POINT ( 'NONE',  ( -38.97545270896704039, -113.1123104723225197, 5.347274454178449155 ) ) ;
#14260=CARTESIAN_POINT ( 'NONE',  ( -34.50000000000000000, -112.0140978167138712, -0.3122823525984337878 ) ) ;
#14266=CARTESIAN_POINT ( 'NONE',  ( -35.50000000000000000, -113.9929510916434339, 10.51175824272318415 ) ) ;
#14270=CARTESIAN_POINT ( 'NONE',  ( -34.50000000000000000, -112.1946304249441795, 2.703640693953100804 ) ) ;
#14272=CARTESIAN_POINT ( 'NONE',  ( -35.50000000000000000, -114.4680894751352156, 8.562575367713533225 ) ) ;
#14295=CARTESIAN_POINT ( 'NONE',  ( -35.97545270896705460, -114.3549511594417680, 5.590225545821552622 ) ) ;
#14303=CARTESIAN_POINT ( 'NONE',  ( -35.50000000000000711, -116.0140978167138712, -0.4997823525984418369 ) ) ;
#14305=CARTESIAN_POINT ( 'NONE',  ( -35.50000000000000711, -114.8211182053456838, 9.932864235516914775 ) ) ;
#14309=CARTESIAN_POINT ( 'NONE',  ( -34.50000000000000000, -114.9929510916434339, 12.39849696637031506 ) ) ;
#14313=CARTESIAN_POINT ( 'NONE',  ( -39.00000000000000000, -115.9929510916434481, 11.21034663311206181 ) ) ;
#14314=CARTESIAN_POINT ( 'NONE',  ( -35.50000000000000711, -112.1403507321855528, -1.128496220798856253 ) ) ;
#14325=CARTESIAN_POINT ( 'NONE',  ( -37.47347596530441649, -113.0245472910329880, 3.527725545821551734 ) ) ;
#14351=CARTESIAN_POINT ( 'NONE',  ( -34.50000000000000000, -115.0140978167138712, -0.5622823525984408377 ) ) ;
#14354=CARTESIAN_POINT ( 'NONE',  ( -34.50000000000000000, -114.8124184834118324, 8.677834500183694288 ) ) ;
#14358=CARTESIAN_POINT ( 'NONE',  ( -34.50000000000000000, -114.2356323198232673, 8.521029492159460261 ) ) ;
#14360=CARTESIAN_POINT ( 'NONE',  ( -34.50000000000000000, -114.0000000000003411, 9.500000000000035527 ) ) ;
#14369=CARTESIAN_POINT ( 'NONE',  ( -34.57658136524562309, -114.9929510916434339, 13.10177712753338497 ) ) ;
#14370=CARTESIAN_POINT ( 'NONE',  ( -36.94073759706866156, -111.0000000000000284, 5.628524454178450043 ) ) ;
#14373=CARTESIAN_POINT ( 'NONE',  ( -35.50000000000000711, -112.5103839485166333, -1.498529437127682495 ) ) ;
#14389=CARTESIAN_POINT ( 'NONE',  ( -34.50000000000000000, -116.9501796819249222, -1.143161139954000260 ) ) ;
#14394=CARTESIAN_POINT ( 'NONE',  ( -37.34375000000001421, -114.9929510916434339, 13.11852480586264669 ) ) ;
#14397=CARTESIAN_POINT ( 'NONE',  ( -34.50000000000000000, -114.0650276068786582, 9.507762098804159123 ) ) ;
#14400=CARTESIAN_POINT ( 'NONE',  ( -34.50000000000000000, -113.9929510916434339, 10.53376102667243508 ) ) ;
#14402=CARTESIAN_POINT ( 'NONE',  ( -35.50000000000000711, -114.9929510916434339, 12.56351784598954424 ) ) ;
#14414=CARTESIAN_POINT ( 'NONE',  ( -35.50000000000000000, -113.0140978167138712, -0.6247823525988807081 ) ) ;
#14416=CARTESIAN_POINT ( 'NONE',  ( -35.62769128460905677, -115.4561184093552413, 6.191024454178448266 ) ) ;
#14421=CARTESIAN_POINT ( 'NONE',  ( -36.94073759706868287, -112.0000000000000142, 7.128524454178449155 ) ) ;
#14424=CARTESIAN_POINT ( 'NONE',  ( -35.50000000000000000, -116.9980674558286040, -0.8858242144478970514 ) ) ;
#14427=CARTESIAN_POINT ( 'NONE',  ( -38.99999999999999289, -113.9407375970686900, 6.753524454178448266 ) ) ;
#14431=CARTESIAN_POINT ( 'NONE',  ( -34.50000000000000000, -112.8655373925166572, 1.864575885149403423 ) ) ;
#14437=CARTESIAN_POINT ( 'NONE',  ( -36.87500000000098765, -113.9929510916434339, 13.11852480586264846 ) ) ;
#14442=CARTESIAN_POINT ( 'NONE',  ( -34.50000000000000000, -111.0140821919084715, 0.8283428459075261596 ) ) ;
#14443=CARTESIAN_POINT ( 'NONE',  ( -38.92341863475394348, -115.9929510916434481, 13.10177712753322155 ) ) ;
#14462=VERTEX_POINT ( 'NONE', #21497 ) ;
#14463=CARTESIAN_POINT ( 'NONE',  ( -36.02454729103297382, -113.5265240346956261, 6.902725545821551734 ) ) ;
#14466=STYLED_ITEM ( 'NONE', ( #12278 ), #30145 ) ;
#14472=CARTESIAN_POINT ( 'NONE',  ( -35.50000000000000711, -114.5974311500472425, -1.624782352598427959 ) ) ;
#14479=CARTESIAN_POINT ( 'NONE',  ( -34.50000000000000000, -114.1021862393805577, 9.512197583835053649 ) ) ;
#14484=CARTESIAN_POINT ( 'NONE',  ( -35.50000000000000000, -115.9929510916434481, 11.21034663311132107 ) ) ;
#14485=CARTESIAN_POINT ( 'NONE',  ( -35.50000000000000711, -113.0796441757086939, 1.890140615870383956 ) ) ;
#14493=CARTESIAN_POINT ( 'NONE',  ( -36.64504884055821776, -112.9754527089670688, 8.215225545821551734 ) ) ;
#14502=CARTESIAN_POINT ( 'NONE',  ( -38.18337828418796676, -117.0245472910329738, 4.465225545821550845 ) ) ;
#14518=CARTESIAN_POINT ( 'NONE',  ( -34.50000000000000000, -114.8057644833805853, -0.6247823525984269599 ) ) ;
#14520=CARTESIAN_POINT ( 'NONE',  ( -34.50000000000000000, -116.0140978167138712, 0.6252176474015648244 ) ) ;
#14521=CARTESIAN_POINT ( 'NONE',  ( -34.50000000000000000, -114.4680894751352156, 8.562575367713533225 ) ) ;
#14526=CARTESIAN_POINT ( 'NONE',  ( -38.42182118622945808, -114.9929510916434339, 13.81802396319329773 ) ) ;
#14537=CARTESIAN_POINT ( 'NONE',  ( -34.00000000000000000, -113.9407375970686758, 6.996475545821551734 ) ) ;
#14539=CARTESIAN_POINT ( 'NONE',  ( -35.50000000000000711, -115.3362660311619692, -1.573728109101206085 ) ) ;
#14552=CARTESIAN_POINT ( 'NONE',  ( -34.97545270896703329, -114.7691647218148745, 7.090225545821551734 ) ) ;
#14557=CARTESIAN_POINT ( 'NONE',  ( -35.50000000000000000, -111.0140978167138570, -0.4685323525984296800 ) ) ;
#14565=CARTESIAN_POINT ( 'NONE',  ( -37.18750000000006395, -114.9929510916434339, 13.11852480586264669 ) ) ;
#14566=CARTESIAN_POINT ( 'NONE',  ( -37.48437500000004263, -113.9929510916434339, 14.11852480586265024 ) ) ;
#14569=CARTESIAN_POINT ( 'NONE',  ( -36.50000000000010658, -113.9929510916434339, 14.11852480586265024 ) ) ;
#14572=CARTESIAN_POINT ( 'NONE',  ( -35.87040530316090070, -114.9929510916434339, 13.10254527216545917 ) ) ;
#14580=CARTESIAN_POINT ( 'NONE',  ( -35.50000000000000711, -114.9929510916434339, 12.26648026267477221 ) ) ;
#14589=CARTESIAN_POINT ( 'NONE',  ( -35.50000000000000000, -113.0140978167141128, -0.6247823525984907977 ) ) ;
#14591=CARTESIAN_POINT ( 'NONE',  ( -36.23083527818512550, -116.0245472910329880, 1.784774454178448932 ) ) ;
#14593=CARTESIAN_POINT ( 'NONE',  ( -38.97545270896704039, -113.1123104723225197, 3.847274454178449599 ) ) ;
#14597=CARTESIAN_POINT ( 'NONE',  ( -35.50000000000000711, -114.3474311500471430, -1.624782352598427959 ) ) ;
#14605=CARTESIAN_POINT ( 'NONE',  ( -34.50000000000000000, -112.0140978167138712, 0.0002176474015661141945 ) ) ;
#14613=CARTESIAN_POINT ( 'NONE',  ( -37.99994980024369085, -113.9929510916434339, 12.62670525340494621 ) ) ;
#14615=CARTESIAN_POINT ( 'NONE',  ( -34.50000000000000000, -112.0140978167138712, 0.7189676474015718188 ) ) ;
#14617=CARTESIAN_POINT ( 'NONE',  ( -35.87040530316090070, -113.9929510916434339, 13.10254527216545917 ) ) ;
#14619=CARTESIAN_POINT ( 'NONE',  ( -35.50160444427493189, -115.9929510916434481, 12.65937477241749853 ) ) ;
#14642=CARTESIAN_POINT ( 'NONE',  ( -38.02454729103295961, -113.6450488405582462, 7.840225545821554398 ) ) ;
#14646=ORIENTED_EDGE ( 'NONE', *, *, #2381, .F. ) ;
#14652=CARTESIAN_POINT ( 'NONE',  ( -35.50000000000000711, -114.9929510916434339, 10.68227981832981044 ) ) ;
#14655=CARTESIAN_POINT ( 'NONE',  ( -34.50000000000000000, -114.2598117360253696, 9.542047897280109936 ) ) ;
#14662=CARTESIAN_POINT ( 'NONE',  ( -35.50000000000000000, -115.9929510916434481, 10.51725893871049067 ) ) ;
#14673=CARTESIAN_POINT ( 'NONE',  ( -37.47347596530441649, -114.9754527089670262, 1.972274454178448932 ) ) ;
#14683=CARTESIAN_POINT ( 'NONE',  ( -34.92058450342251064, -116.1632251905417945, 6.191024454178448266 ) ) ;
#14703=CARTESIAN_POINT ( 'NONE',  ( -34.50000000000000000, -113.0796441757086939, 1.890140615870383956 ) ) ;
#14706=CARTESIAN_POINT ( 'NONE',  ( -39.00000000000000711, -114.9929510916434339, 12.50851088611646311 ) ) ;
#14709=CARTESIAN_POINT ( 'NONE',  ( -34.50000000000000000, -114.2067765580549832, 8.517583185305328541 ) ) ;
#14719=CARTESIAN_POINT ( 'NONE',  ( -37.05926240293131713, -111.0000000000000284, 5.121475545821551734 ) ) ;
#14723=CARTESIAN_POINT ( 'NONE',  ( -35.50000000000000711, -113.3474311500483935, -1.624782352598427959 ) ) ;
#14737=CARTESIAN_POINT ( 'NONE',  ( -38.99999999999999289, -114.0592624029313242, 4.746475545821550845 ) ) ;
#14745=CARTESIAN_POINT ( 'NONE',  ( -35.50000000000000000, -111.0140978167138570, -0.1247823525984260717 ) ) ;
#14751=CARTESIAN_POINT ( 'NONE',  ( -39.00000000000000000, -113.9929510916434339, 11.91443571948719615 ) ) ;
#14755=CARTESIAN_POINT ( 'NONE',  ( -37.48437500000004263, -113.9929510916434339, 14.11852480586265024 ) ) ;
#14758=CARTESIAN_POINT ( 'NONE',  ( -35.99181955245763476, -114.9929510916434339, 13.11847460610632687 ) ) ;
#14766=CARTESIAN_POINT ( 'NONE',  ( -35.56312645773537895, -114.9929510916434339, 12.87038173996308998 ) ) ;
#14775=CARTESIAN_POINT ( 'NONE',  ( -35.50000000000000000, -113.0140978167136581, -0.6247823525984261828 ) ) ;
#14781=CARTESIAN_POINT ( 'NONE',  ( -38.37230871539094323, -112.5438815906447729, 2.441024454178448710 ) ) ;
#14785=CARTESIAN_POINT ( 'NONE',  ( -35.50000000000000711, -112.8511839106603247, -1.611965039240275122 ) ) ;
#14795=CARTESIAN_POINT ( 'NONE',  ( -34.50000000000000000, -112.9486715495423681, -1.623175561345890472 ) ) ;
#14803=CARTESIAN_POINT ( 'NONE',  ( -35.83891589277641287, -113.9929510916434339, 13.09299768411358400 ) ) ;
#14804=CARTESIAN_POINT ( 'NONE',  ( -34.50000000000000000, -113.1256619669233885, 1.895633585076891947 ) ) ;
#14806=CARTESIAN_POINT ( 'NONE',  ( -36.03125000000003553, -113.9929510916434339, 13.11852480586264846 ) ) ;
#14809=CARTESIAN_POINT ( 'NONE',  ( -35.50000000000000000, -115.9929510916434481, 12.60752341388803721 ) ) ;
#14822=CARTESIAN_POINT ( 'NONE',  ( -35.50000000000000711, -113.2637153405686519, 1.912112492696748989 ) ) ;
#14830=CARTESIAN_POINT ( 'NONE',  ( -34.50000000000000000, -112.6882700046066645, -2.599147725882136939 ) ) ;
#14831=DIRECTION ( 'NONE',  ( 0.000000000000000000, -0.9929510916431035783, 0.1185248058626076212 ) ) ;
#14834=CARTESIAN_POINT ( 'NONE',  ( -36.33479806579561000, -114.7490116281687165, 1.691024454178448932 ) ) ;
#14839=CARTESIAN_POINT ( 'NONE',  ( -35.50000000000000000, -115.0140978167140986, -0.6247823525984417259 ) ) ;
#14842=CARTESIAN_POINT ( 'NONE',  ( -35.50000000000000711, -114.9929510916434339, 10.56126450660895699 ) ) ;
#14846=CARTESIAN_POINT ( 'NONE',  ( -34.50000000000000000, -114.0928965812550757, 9.511088712577292270 ) ) ;
#14851=CARTESIAN_POINT ( 'NONE',  ( -35.50000000000000000, -114.2114213871176958, 8.518137620934190579 ) ) ;
#14852=CARTESIAN_POINT ( 'NONE',  ( -35.50000000000000711, -112.0140978167138712, 0.7502176474015694874 ) ) ;
#14862=CARTESIAN_POINT ( 'NONE',  ( -36.64504884055821776, -112.9754527089670688, 5.215225545821552622 ) ) ;
#14870=CARTESIAN_POINT ( 'NONE',  ( -39.99999999999999289, -114.0592624029313242, 9.246475545821549957 ) ) ;
#14884=CARTESIAN_POINT ( 'NONE',  ( -34.50000000000000000, -114.5974311500472567, -0.6247823525984269599 ) ) ;
#14888=CARTESIAN_POINT ( 'NONE',  ( -39.00000000000000711, -114.9929510916434339, 10.85830208992306822 ) ) ;
#14890=CARTESIAN_POINT ( 'NONE',  ( -39.00000000000000711, -114.9929510916434339, 11.73841344789285657 ) ) ;
#14900=CARTESIAN_POINT ( 'NONE',  ( -38.18337828418796676, -117.0245472910329738, 4.465225545821550845 ) ) ;
#14902=CARTESIAN_POINT ( 'NONE',  ( -35.50000000000000000, -113.0140978167138712, 0.5627176474015715968 ) ) ;
#14918=CARTESIAN_POINT ( 'NONE',  ( -35.50000000000000000, -115.1449503510569059, -2.621568770093253953 ) ) ;
#14921=CARTESIAN_POINT ( 'NONE',  ( -37.62959469683911351, -114.9929510916434339, 13.10254527216511633 ) ) ;
#14924=CARTESIAN_POINT ( 'NONE',  ( -37.56132887387857267, -113.9929510916434339, 14.11732072679899197 ) ) ;
#14929=CARTESIAN_POINT ( 'NONE',  ( -38.99518666717493431, -113.9929510916434339, 12.74107470552714894 ) ) ;
#14932=CARTESIAN_POINT ( 'NONE',  ( -36.07812499999994316, -114.9929510916434339, 13.11852480586264669 ) ) ;
#14938=CARTESIAN_POINT ( 'NONE',  ( -35.50000000000000711, -114.9929510916434339, 10.61627146648203812 ) ) ;
#14941=CARTESIAN_POINT ( 'NONE',  ( -37.05926240293131713, -115.9999999999999858, 3.378524454178448710 ) ) ;
#14947=CARTESIAN_POINT ( 'NONE',  ( -34.50000000000000000, -113.0140978167137860, 0.8752176474016654106 ) ) ;
#14949=CARTESIAN_POINT ( 'NONE',  ( -36.94073759706868287, -112.0000000000000142, 8.628524454178448266 ) ) ;
#14951=CARTESIAN_POINT ( 'NONE',  ( -34.97545270896703329, -113.2308352781851539, 5.909774454178449155 ) ) ;
#14954=CARTESIAN_POINT ( 'NONE',  ( -35.50000000000000711, -114.1807644833817648, -1.624782352598427959 ) ) ;
#14964=CARTESIAN_POINT ( 'NONE',  ( -34.50000000000000000, -113.0071371610607684, 2.888584676720006961 ) ) ;
#14965=CARTESIAN_POINT ( 'NONE',  ( -35.50000000000000711, -112.7472371723319355, 1.839427296857320648 ) ) ;
#14971=CARTESIAN_POINT ( 'NONE',  ( -37.93687354226506869, -113.9929510916434339, 12.87038173996323565 ) ) ;
#14975=CARTESIAN_POINT ( 'NONE',  ( -35.50000000000000000, -113.9929510916434339, 12.17846912687782712 ) ) ;
#14976=CARTESIAN_POINT ( 'NONE',  ( -35.50000000000000000, -115.9792481177720731, 10.26484292309424795 ) ) ;
#14991=CARTESIAN_POINT ( 'NONE',  ( -35.50000000000000711, -112.8655373925166572, 1.864575885149403423 ) ) ;
#14993=CARTESIAN_POINT ( 'NONE',  ( -35.50000000000000711, -114.0998638248492085, 9.511920366020609308 ) ) ;
#14997=CARTESIAN_POINT ( 'NONE',  ( -34.50000000000000000, -113.4307644833805142, -2.624782352598442614 ) ) ;
#15001=CARTESIAN_POINT ( 'NONE',  ( -36.25098837183130485, -114.6652019342044184, 8.683975545821549957 ) ) ;
#15006=CARTESIAN_POINT ( 'NONE',  ( -35.50000000000000000, -115.0140978167138712, -0.3747823525984422255 ) ) ;
#15014=CARTESIAN_POINT ( 'NONE',  ( -35.50040135968785648, -114.9929510916434339, 12.63896776382214071 ) ) ;
#15019=CARTESIAN_POINT ( 'NONE',  ( -34.51922597003733273, -114.9929510916434339, 12.86289566494349224 ) ) ;
#15023=CARTESIAN_POINT ( 'NONE',  ( -35.50000000000000000, -114.2067765580549832, 8.517583185305328541 ) ) ;
#15034=CARTESIAN_POINT ( 'NONE',  ( -36.33479806579560289, -113.2509883718313262, 8.308975545821549957 ) ) ;
#15042=CARTESIAN_POINT ( 'NONE',  ( -38.18337828418796676, -117.0245472910329738, 5.965225545821550845 ) ) ;
#15057=CARTESIAN_POINT ( 'NONE',  ( -34.50000000000000000, -112.5103839485166333, -1.498529437127682495 ) ) ;
#15060=CARTESIAN_POINT ( 'NONE',  ( -36.07812499999994316, -115.9929510916434481, 14.11852480586265024 ) ) ;
#15063=CARTESIAN_POINT ( 'NONE',  ( -37.98325232167028531, -114.9929510916434339, 14.04194344061727406 ) ) ;
#15070=CARTESIAN_POINT ( 'NONE',  ( -34.00000000000000000, -113.9407375970686758, 3.996475545821551734 ) ) ;
#15072=CARTESIAN_POINT ( 'NONE',  ( -35.50000000000000000, -113.0140978167138712, -0.6247823525979733228 ) ) ;
#15084=CARTESIAN_POINT ( 'NONE',  ( -34.97545270896703329, -114.7691647218148745, 5.590225545821551734 ) ) ;
#15089=CARTESIAN_POINT ( 'NONE',  ( -35.50000000000000000, -115.5324766040685631, -2.560864217809699195 ) ) ;
#15095=CARTESIAN_POINT ( 'NONE',  ( -37.53269373325071712, -114.9929510916434339, 13.11752178341324360 ) ) ;
#15097=CARTESIAN_POINT ( 'NONE',  ( -34.50000000000000000, -114.1414532730574507, 9.517316564499758158 ) ) ;
#15100=CARTESIAN_POINT ( 'NONE',  ( -36.99999999999989342, -114.9929510916434339, 13.11852480586264669 ) ) ;
#15103=CARTESIAN_POINT ( 'NONE',  ( -37.42187499999996447, -113.9929510916434339, 14.11852480586265024 ) ) ;
#15105=CARTESIAN_POINT ( 'NONE',  ( -35.50000000000000711, -114.9929510916434339, 12.57451923796416082 ) ) ;
#15111=CARTESIAN_POINT ( 'NONE',  ( -35.50000000000000711, -114.9929517792218689, 10.50900788599415314 ) ) ;
#15113=CARTESIAN_POINT ( 'NONE',  ( -35.00000000000000000, -114.0592624029313242, 3.003524454178448710 ) ) ;
#15117=CARTESIAN_POINT ( 'NONE',  ( -34.50000000000000000, -113.0140978167138712, -0.1247823525984260717 ) ) ;
#15121=CARTESIAN_POINT ( 'NONE',  ( -38.45611840935523418, -115.3723087153909432, 6.566024454178448266 ) ) ;
#15125=CARTESIAN_POINT ( 'NONE',  ( -35.50000000000000711, -112.5103839485166333, -1.498529437127682495 ) ) ;
#15132=FILL_AREA_STYLE ('',( #20544 ) ) ;
#15136=CARTESIAN_POINT ( 'NONE',  ( -34.50000000000000000, -113.8474311500459777, -1.624782352598427959 ) ) ;
#15137=CARTESIAN_POINT ( 'NONE',  ( -35.50000000000000711, -112.0250551866464548, 1.025914454044489332 ) ) ;
#15145=CARTESIAN_POINT ( 'NONE',  ( -37.66108410722335265, -113.9929510916434339, 13.09299768411426612 ) ) ;
#15147=CARTESIAN_POINT ( 'NONE',  ( -37.34375000000001421, -113.9929510916434339, 13.11852480586264846 ) ) ;
#15148=CARTESIAN_POINT ( 'NONE',  ( -35.50000000000000000, -115.9929510916434481, 10.56126450660895699 ) ) ;
#15160=CARTESIAN_POINT ( 'NONE',  ( -35.50000000000000711, -112.0140978167138712, -0.4685323525984295134 ) ) ;
#15162=CARTESIAN_POINT ( 'NONE',  ( -35.50000000000000711, -114.0743172650041686, 9.508870970061893857 ) ) ;
#15166=ADVANCED_FACE ( 'NONE', ( #8139 ), #12828, .T. ) ;
#15167=CARTESIAN_POINT ( 'NONE',  ( -34.50000000000000000, -117.0140978167138854, -0.5622823525984408377 ) ) ;
#15172=CARTESIAN_POINT ( 'NONE',  ( -35.99999999999999289, -114.0592624029313242, 3.003524454178448710 ) ) ;
#15176=CARTESIAN_POINT ( 'NONE',  ( -35.50000000000000000, -115.0140978167137860, -0.6247823525984403936 ) ) ;
#15182=CARTESIAN_POINT ( 'NONE',  ( -35.50025087934803736, -114.9929510916434339, 12.63488142334835196 ) ) ;
#15184=CARTESIAN_POINT ( 'NONE',  ( -37.56132887387857267, -114.9929510916434339, 14.11732072679899197 ) ) ;
#15188=CARTESIAN_POINT ( 'NONE',  ( -35.50000000000000000, -115.9929510916434481, 12.60752341388803721 ) ) ;
#15189=CARTESIAN_POINT ( 'NONE',  ( -35.50000000000000711, -114.8474311500471572, -1.624782352598427959 ) ) ;
#15202=CARTESIAN_POINT ( 'NONE',  ( -37.35495115944176803, -115.0245472910329880, 7.465225545821552622 ) ) ;
#15212=CARTESIAN_POINT ( 'NONE',  ( -35.81662171581203324, -110.9754527089670546, 9.715225545821551734 ) ) ;
#15233=CARTESIAN_POINT ( 'NONE',  ( -34.50000000000000000, -115.9929510916434481, 12.53051367006571581 ) ) ;
#15236=CARTESIAN_POINT ( 'NONE',  ( -34.68937937320795584, -115.9929510916434481, 13.37409560816408671 ) ) ;
#15248=CARTESIAN_POINT ( 'NONE',  ( -38.18337828418796676, -117.0245472910329738, 2.965225545821551734 ) ) ;
#15250=CARTESIAN_POINT ( 'NONE',  ( -35.50000000000000000, -112.9977353549762000, -0.6247823525983134951 ) ) ;
#15265=CARTESIAN_POINT ( 'NONE',  ( -35.62769128460905677, -112.5438815906447729, 8.308975545821549957 ) ) ;
#15270=CARTESIAN_POINT ( 'NONE',  ( -35.50000000000000000, -111.0140978167138570, -0.4997823525984338988 ) ) ;
#15274=CARTESIAN_POINT ( 'NONE',  ( -38.00000000000000711, -114.9929510916434339, 10.50625754673587231 ) ) ;
#15275=CARTESIAN_POINT ( 'NONE',  ( -34.50000000000000000, -114.9929510916434339, 12.60752341388803544 ) ) ;
#15278=CARTESIAN_POINT ( 'NONE',  ( -37.93687354226506869, -114.9929510916434339, 12.87038173996323565 ) ) ;
#15280=CARTESIAN_POINT ( 'NONE',  ( -35.24442919769867899, -113.9929510916434339, 13.92914543265605509 ) ) ;
#15291=CARTESIAN_POINT ( 'NONE',  ( -35.50000000000000711, -114.9929510916434339, 10.51175824272318415 ) ) ;
#15293=CARTESIAN_POINT ( 'NONE',  ( -35.62769128460905677, -115.4561184093552413, 1.691024454178448710 ) ) ;
#15299=CARTESIAN_POINT ( 'NONE',  ( -34.50000000000000000, -113.0140978167138712, 0.2502176474015764263 ) ) ;
#15301=CARTESIAN_POINT ( 'NONE',  ( -35.62769128460905677, -115.4561184093552413, 7.691024454178449155 ) ) ;
#15303=CARTESIAN_POINT ( 'NONE',  ( -35.81662171581204746, -117.0245472910329738, 1.784774454178449155 ) ) ;
#15306=CARTESIAN_POINT ( 'NONE',  ( -35.50000000000000711, -116.0124910254613297, -0.6902086197697608894 ) ) ;
#15315=CARTESIAN_POINT ( 'NONE',  ( -34.50000000000000000, -116.0140978167138712, -0.5622823525984409487 ) ) ;
#15317=CARTESIAN_POINT ( 'NONE',  ( -35.50000000000000711, -112.0140978167138712, 0.6252176474015680441 ) ) ;
#15323=CARTESIAN_POINT ( 'NONE',  ( -34.50000000000000000, -113.9697269463297431, 10.50348536859153370 ) ) ;
#15325=CARTESIAN_POINT ( 'NONE',  ( -35.49999931242378182, -113.9929510916434339, 12.61439929482945743 ) ) ;
#15326=CARTESIAN_POINT ( 'NONE',  ( -35.87040530316090070, -115.9929510916434481, 13.10254527216545917 ) ) ;
#15339=CARTESIAN_POINT ( 'NONE',  ( -35.50000000000000711, -115.0468226098135744, -1.624774171496087716 ) ) ;
#15344=CARTESIAN_POINT ( 'NONE',  ( -35.50000000000000711, -114.1189822439768449, 9.514224058074130852 ) ) ;
#15348=CARTESIAN_POINT ( 'NONE',  ( -35.50000000000000000, -113.1451905347060460, 2.905063584339864668 ) ) ;
#15352=CARTESIAN_POINT ( 'NONE',  ( -37.05926240293133134, -115.0000000000000000, 4.878524454178448266 ) ) ;
#15356=CARTESIAN_POINT ( 'NONE',  ( -35.50000000000000000, -115.0140978167137860, -0.6411448143358557950 ) ) ;
#15362=CARTESIAN_POINT ( 'NONE',  ( -35.50000000000000000, -113.9917898843777522, 10.50611893782865813 ) ) ;
#15365=CARTESIAN_POINT ( 'NONE',  ( -36.03906250000000000, -114.9929510916434339, 14.11852480586264846 ) ) ;
#15371=CARTESIAN_POINT ( 'NONE',  ( -35.99181955245763476, -115.9929510916434481, 13.11847460610632510 ) ) ;
#15372=CARTESIAN_POINT ( 'NONE',  ( -35.50000000000000711, -116.0140978167138712, 0.3752176474015736507 ) ) ;
#15384=CARTESIAN_POINT ( 'NONE',  ( -36.64504884055823908, -115.0245472910329880, 7.784774454178449155 ) ) ;
#15395=CARTESIAN_POINT ( 'NONE',  ( -36.94073759706868287, -115.9999999999999858, 2.871475545821551290 ) ) ;
#15415=CARTESIAN_POINT ( 'NONE',  ( -34.54793860109200665, -115.9929510916434481, 13.00730889637958221 ) ) ;
#15419=CARTESIAN_POINT ( 'NONE',  ( -38.99999999999999289, -113.9407375970686900, 6.753524454178448266 ) ) ;
#15421=CARTESIAN_POINT ( 'NONE',  ( -34.50000000000000000, -115.9929510916434481, 12.59102132592610346 ) ) ;
#15428=CARTESIAN_POINT ( 'NONE',  ( -38.45611840935523418, -112.6276912846090568, 3.433975545821551290 ) ) ;
#15430=CARTESIAN_POINT ( 'NONE',  ( -35.50000000000000000, -113.0140978167143260, -0.6247823525984285142 ) ) ;
#15448=CARTESIAN_POINT ( 'NONE',  ( -35.50000000000000711, -112.0140978167138712, -0.3747823525984256832 ) ) ;
#15454=CARTESIAN_POINT ( 'NONE',  ( -34.50000000000000000, -112.4434344552011282, 1.705278471174987986 ) ) ;
#15455=CARTESIAN_POINT ( 'NONE',  ( -34.50000000000000000, -114.9929517792218689, 10.50900788599415314 ) ) ;
#15459=CARTESIAN_POINT ( 'NONE',  ( -36.62499999999902656, -114.9929510916434339, 13.11852480586264669 ) ) ;
#15462=CARTESIAN_POINT ( 'NONE',  ( -34.50000000000000000, -114.5636144531578680, 9.676196722963288366 ) ) ;
#15464=CARTESIAN_POINT ( 'NONE',  ( -37.58145695302688694, -114.9929510916434339, 13.11211614918362756 ) ) ;
#15470=CARTESIAN_POINT ( 'NONE',  ( -36.50000000000011369, -114.9929510916434339, 13.11852480586264669 ) ) ;
#15473=CARTESIAN_POINT ( 'NONE',  ( -38.45611840935523418, -115.3723087153909432, 3.566024454178448710 ) ) ;
#15479=CARTESIAN_POINT ( 'NONE',  ( -34.50000000000000000, -113.0140978167136581, -0.6247823525984261828 ) ) ;
#15483=CARTESIAN_POINT ( 'NONE',  ( -39.02454729103295961, -114.7691647218148745, 8.159774454178448266 ) ) ;
#15485=CARTESIAN_POINT ( 'NONE',  ( -35.50000000000000711, -116.0140978167138712, -0.1247823525984439463 ) ) ;
#15495=CARTESIAN_POINT ( 'NONE',  ( -34.50000000000000000, -115.8878449012421754, -1.128496220799388494 ) ) ;
#15498=PRODUCT_DEFINITION_FORMATION_WITH_SPECIFIED_SOURCE ( 'ANY', '', #31947, .NOT_KNOWN. ) ;
#15503=CARTESIAN_POINT ( 'NONE',  ( -38.00000000000000711, -113.9929510916434339, 12.53051367006571937 ) ) ;
#15505=CARTESIAN_POINT ( 'NONE',  ( -34.50000000000000000, -113.8814751941377352, 10.49295109164313722 ) ) ;
#15506=CARTESIAN_POINT ( 'NONE',  ( -37.97447287825094264, -115.9929510916434481, 12.77960891308616809 ) ) ;
#15517=CARTESIAN_POINT ( 'NONE',  ( -35.50000000000000711, -112.0250551866464548, 1.025914454044489332 ) ) ;
#15521=CARTESIAN_POINT ( 'NONE',  ( -35.50000000000000711, -114.1861579685891712, 9.524983039397698192 ) ) ;
#15525=CARTESIAN_POINT ( 'NONE',  ( -34.50000000000000000, -113.8474311500459777, -2.624782352598442614 ) ) ;
#15529=CARTESIAN_POINT ( 'NONE',  ( -37.66520193420439000, -113.2509883718312977, 6.941024454178450043 ) ) ;
#15533=CARTESIAN_POINT ( 'NONE',  ( -34.50000000000000000, -112.9990795116828650, 0.8734249692896993711 ) ) ;
#15539=CARTESIAN_POINT ( 'NONE',  ( -37.80727372874345349, -114.9929510916434339, 13.01835785830664527 ) ) ;
#15543=CARTESIAN_POINT ( 'NONE',  ( -35.75562914091914024, -114.9929510916434339, 14.09929883582542409 ) ) ;
#15548=CARTESIAN_POINT ( 'NONE',  ( -35.87040530316090070, -115.9929510916434481, 13.10254527216545917 ) ) ;
#15559=CARTESIAN_POINT ( 'NONE',  ( -37.05926240293133134, -115.0000000000000000, 3.378524454178448710 ) ) ;
#15567=CARTESIAN_POINT ( 'NONE',  ( -35.00000000000000000, -113.9407375970686900, 2.496475545821551290 ) ) ;
#15584=CARTESIAN_POINT ( 'NONE',  ( -38.50000000000000711, -114.9929510916434339, 10.50625754673587231 ) ) ;
#15586=CARTESIAN_POINT ( 'NONE',  ( -34.50000000000000000, -115.9929510916434481, 11.73841344789270202 ) ) ;
#15588=CARTESIAN_POINT ( 'NONE',  ( -37.05926240293131713, -115.9999999999999858, 7.878524454178450043 ) ) ;
#15590=CARTESIAN_POINT ( 'NONE',  ( -34.50000000000000000, -115.9710363517788068, 10.20486393345008835 ) ) ;
#15599=CARTESIAN_POINT ( 'NONE',  ( -35.54388159064475872, -115.3723087153909432, 2.683975545821551290 ) ) ;
#15602=CARTESIAN_POINT ( 'NONE',  ( -35.50000000000000000, -113.2441867727860227, 0.9026824934337903672 ) ) ;
#15621=CARTESIAN_POINT ( 'NONE',  ( -35.50000000000000711, -112.0269151300720409, -0.7876962586524208776 ) ) ;
#15631=CARTESIAN_POINT ( 'NONE',  ( -34.50000000000000000, -114.8847986568751907, 10.03799953695244618 ) ) ;
#15633=CARTESIAN_POINT ( 'NONE',  ( -36.01562499999996447, -114.9929510916434339, 13.11852480586264669 ) ) ;
#15635=CARTESIAN_POINT ( 'NONE',  ( -34.50000000000000000, -114.6604609523327838, 9.751889438017201428 ) ) ;
#15637=CARTESIAN_POINT ( 'NONE',  ( -37.99999897736218202, -114.9929510916434339, 12.62466071271732915 ) ) ;
#15638=DIRECTION ( 'NONE',  ( 0.000000000000000000, -0.9929510916431035783, 0.1185248058626076212 ) ) ;
#15644=CARTESIAN_POINT ( 'NONE',  ( -37.99959864031215773, -114.9929510916434339, 12.63896776382213538 ) ) ;
#15648=CARTESIAN_POINT ( 'NONE',  ( -36.11231047232249125, -112.0245472910329880, 7.222274454178451819 ) ) ;
#15657=CARTESIAN_POINT ( 'NONE',  ( -37.05926240293133134, -116.9999999999999858, 1.878524454178448710 ) ) ;
#15666=EDGE_CURVE ( 'NONE', #19761, #24733, #16482, .T. ) ;
#15671=CARTESIAN_POINT ( 'NONE',  ( -34.50000000000000000, -113.0974311500471714, -2.624782352598442614 ) ) ;
#15677=CARTESIAN_POINT ( 'NONE',  ( -35.50000000000000711, -114.4026847875275337, 9.592046023459676718 ) ) ;
#15679=CARTESIAN_POINT ( 'NONE',  ( -34.50000000000000000, -113.9743717753924699, 10.50403980422039396 ) ) ;
#15682=CARTESIAN_POINT ( 'NONE',  ( -38.00000000000000711, -113.9929510916434339, 12.53051367006571937 ) ) ;
#15683=CARTESIAN_POINT ( 'NONE',  ( -37.89983305244309264, -115.9929510916434481, 12.92579853460519423 ) ) ;
#15698=CARTESIAN_POINT ( 'NONE',  ( -35.50000000000000711, -112.0140978167138712, -0.4997823525984337878 ) ) ;
#15705=CARTESIAN_POINT ( 'NONE',  ( -35.50000000000000000, -113.1807644833805426, -2.624782352598442614 ) ) ;
#15708=ORIENTED_EDGE ( 'NONE', *, *, #23890, .T. ) ;
#15710=CARTESIAN_POINT ( 'NONE',  ( -37.74901162816869515, -114.6652019342044042, 6.566024454178448266 ) ) ;
#15716=CARTESIAN_POINT ( 'NONE',  ( -34.50000000000000000, -113.2224311500466030, -0.6247823525984269599 ) ) ;
#15720=CARTESIAN_POINT ( 'NONE',  ( -37.50613590685470911, -114.9929510916434339, 13.11852378322482515 ) ) ;
#15724=CARTESIAN_POINT ( 'NONE',  ( -34.50000000000000000, -112.0140978167138712, 0.7189676474015718188 ) ) ;
#15725=CARTESIAN_POINT ( 'NONE',  ( -34.49999793727135255, -114.9929510916434339, 12.61164896875036590 ) ) ;
#15729=CARTESIAN_POINT ( 'NONE',  ( -37.24999999999992184, -115.9929510916434481, 13.11852480586264846 ) ) ;
#15730=CARTESIAN_POINT ( 'NONE',  ( -35.50000000000000711, -115.5178116849130276, -1.498529437126731034 ) ) ;
#15739=CARTESIAN_POINT ( 'NONE',  ( -36.33479806579561000, -114.7490116281687165, 7.691024454178450043 ) ) ;
#15745=CARTESIAN_POINT ( 'NONE',  ( -35.00000000000000000, -114.0592624029313953, 1.503524454178449599 ) ) ;
#15750=CARTESIAN_POINT ( 'NONE',  ( -36.94073759706868287, -115.9999999999999858, 8.871475545821551734 ) ) ;
#15767=CARTESIAN_POINT ( 'NONE',  ( -34.97545270896703329, -113.2308352781851397, 8.909774454178448266 ) ) ;
#15768=CARTESIAN_POINT ( 'NONE',  ( -34.50000000000000000, -115.9929510916434481, 12.50851088611648265 ) ) ;
#15778=CARTESIAN_POINT ( 'NONE',  ( -39.99999999999999289, -114.0592624029313242, 9.246475545821549957 ) ) ;
#15798=CARTESIAN_POINT ( 'NONE',  ( -35.50000000000000711, -113.1256619669233885, 1.895633585076891947 ) ) ;
#15806=CARTESIAN_POINT ( 'NONE',  ( -34.50000000000000000, -112.0154707866092707, 0.9357013553229778235 ) ) ;
#15807=CARTESIAN_POINT ( 'NONE',  ( -34.54793860109200665, -114.9929510916434339, 13.00730889637958221 ) ) ;
#15809=CARTESIAN_POINT ( 'NONE',  ( -37.99839555572501837, -114.9929510916434339, 12.65937477241748965 ) ) ;
#15811=CARTESIAN_POINT ( 'NONE',  ( -34.50000000000000000, -114.3464919575557843, 9.568884482464163455 ) ) ;
#15821=CARTESIAN_POINT ( 'NONE',  ( -37.99999897736218202, -114.9929510916434339, 12.62466071271732915 ) ) ;
#15824=CARTESIAN_POINT ( 'NONE',  ( -39.16322519054179452, -116.0794154965774823, 2.066024454178448710 ) ) ;
#15832=CARTESIAN_POINT ( 'NONE',  ( -34.83677480945819838, -111.9205845034225462, 4.316024454178448266 ) ) ;
#15845=CARTESIAN_POINT ( 'NONE',  ( -34.50000000000000000, -112.0066700803175763, -2.372276521656937920 ) ) ;
#15849=CARTESIAN_POINT ( 'NONE',  ( -35.50000000000000711, -114.9922651054798308, 10.46846006712531008 ) ) ;
#15854=CARTESIAN_POINT ( 'NONE',  ( -34.50000000000000000, -113.9929510916434339, 10.51175824272318415 ) ) ;
#15858=CARTESIAN_POINT ( 'NONE',  ( -37.75185693410092824, -113.9929510916434339, 13.05539834812634759 ) ) ;
#15860=CARTESIAN_POINT ( 'NONE',  ( -36.07812499999994316, -115.9929510916434481, 13.11852480586264846 ) ) ;
#15874=CARTESIAN_POINT ( 'NONE',  ( -35.50000000000000711, -112.0577668799241309, 1.173706424699810569 ) ) ;
#15876=CARTESIAN_POINT ( 'NONE',  ( -35.50000000000000711, -114.9929510916434339, 10.55026311463432087 ) ) ;
#15884=CARTESIAN_POINT ( 'NONE',  ( -35.50000000000000000, -114.1807644833817648, -2.624782352598442614 ) ) ;
#15888=CARTESIAN_POINT ( 'NONE',  ( -38.97545270896704039, -113.1123104723225197, 2.347274454178448710 ) ) ;
#15894=CARTESIAN_POINT ( 'NONE',  ( -34.50000000000000000, -114.8057644833805853, -0.6247823525984269599 ) ) ;
#15900=CARTESIAN_POINT ( 'NONE',  ( -38.00000000000000711, -114.9929510916434339, 12.17846912687782179 ) ) ;
#15904=CARTESIAN_POINT ( 'NONE',  ( -34.50000000000000000, -112.8511839106603247, -1.611965039240275122 ) ) ;
#15905=COLOUR_RGB ( '', 0.08235294, 0.09019608, 0.10196078) ;
#15914=CARTESIAN_POINT ( 'NONE',  ( -37.49414064056232831, -115.9929510916434481, 13.11852578240983291 ) ) ;
#15934=CARTESIAN_POINT ( 'NONE',  ( -35.02454729103298803, -113.1123104723225197, 8.402725545821549957 ) ) ;
#15955=CARTESIAN_POINT ( 'NONE',  ( -38.37230871539094323, -112.5438815906447729, 6.941024454178449155 ) ) ;
#15956=CARTESIAN_POINT ( 'NONE',  ( -35.07817881376918479, -115.9929510916434481, 13.81802396319203474 ) ) ;
#15966=CARTESIAN_POINT ( 'NONE',  ( -38.30190309005061522, -111.0245472910330022, 9.527725545821551734 ) ) ;
#15983=CARTESIAN_POINT ( 'NONE',  ( -35.50000000000000711, -112.0140978167138712, 0.6252176474015680441 ) ) ;
#15990=CARTESIAN_POINT ( 'NONE',  ( -34.50000000000000000, -115.9630435732166518, -0.9469505670456015434 ) ) ;
#15991=CARTESIAN_POINT ( 'NONE',  ( -38.81062062679291103, -114.9929510916434339, 13.37409560816442067 ) ) ;
#15993=CARTESIAN_POINT ( 'NONE',  ( -35.50000000000000000, -113.9929510916434339, 10.52826033068511435 ) ) ;
#15996=CARTESIAN_POINT ( 'NONE',  ( -34.50000000000000000, -114.9929510916434339, 10.55026311463432087 ) ) ;
#15998=CARTESIAN_POINT ( 'NONE',  ( -38.00000000000000711, -114.9929510916434339, 12.50851088611646311 ) ) ;
#15999=SURFACE_STYLE_FILL_AREA ( #10271 ) ;
#16004=CARTESIAN_POINT ( 'NONE',  ( -38.00000000000000711, -114.9929510916434339, 12.44250253426874941 ) ) ;
#16006=CARTESIAN_POINT ( 'NONE',  ( -35.00000000000000000, -114.0592624029313242, 7.503524454178449155 ) ) ;
#16014=CARTESIAN_POINT ( 'NONE',  ( -36.23083527818512550, -116.0245472910329880, 7.784774454178451819 ) ) ;
#16017=ORIENTED_EDGE ( 'NONE', *, *, #10831, .T. ) ;
#16024=CARTESIAN_POINT ( 'NONE',  ( -34.50000000000000000, -111.1014359431343905, 1.472195201997948510 ) ) ;
#16030=CARTESIAN_POINT ( 'NONE',  ( -35.50000000000000711, -114.9929501463477663, 10.50247632894551231 ) ) ;
#16032=CARTESIAN_POINT ( 'NONE',  ( -34.50000000000000000, -113.9186338266397058, 10.49738657667399266 ) ) ;
#16036=CARTESIAN_POINT ( 'NONE',  ( -34.50000000000000000, -113.9929510916434339, 10.50625754673586876 ) ) ;
#16037=CARTESIAN_POINT ( 'NONE',  ( -36.99999999999988631, -115.9929510916434481, 13.11852480586264846 ) ) ;
#16047=CARTESIAN_POINT ( 'NONE',  ( -35.50000000000000711, -115.3362660311619692, -1.573728109101206085 ) ) ;
#16050=CARTESIAN_POINT ( 'NONE',  ( -35.50000000000000711, -114.9902084924877954, 10.43071793783961176 ) ) ;
#16056=CARTESIAN_POINT ( 'NONE',  ( -35.50000000000000000, -111.0140978167138570, 0.2502176474015764263 ) ) ;
#16059=CARTESIAN_POINT ( 'NONE',  ( -37.99999999999998579, -113.9407375970686758, 8.253524454178448266 ) ) ;
#16064=CARTESIAN_POINT ( 'NONE',  ( -34.50000000000000000, -113.0140978167137860, -0.6247823525984055326 ) ) ;
#16071=CARTESIAN_POINT ( 'NONE',  ( -37.99599240977853754, -114.9929510916434339, 12.68378527132499478 ) ) ;
#16075=CARTESIAN_POINT ( 'NONE',  ( -34.50000000000000000, -112.0140978167138712, 0.6252176474015680441 ) ) ;
#16082=CARTESIAN_POINT ( 'NONE',  ( -38.00000000000000711, -114.9929510916434339, 12.57451923796417503 ) ) ;
#16083=CARTESIAN_POINT ( 'NONE',  ( -37.52044295795950291, -115.9929510916434481, 13.11812344617477422 ) ) ;
#16105=CARTESIAN_POINT ( 'NONE',  ( -35.62769128460905677, -112.5438815906447729, 6.808975545821550845 ) ) ;
#16125=CARTESIAN_POINT ( 'NONE',  ( -37.76916472181487450, -111.9754527089670404, 5.534774454178449155 ) ) ;
#16126=CARTESIAN_POINT ( 'NONE',  ( -37.69578139638701941, -115.9929510916434481, 14.10650203519847778 ) ) ;
#16135=CARTESIAN_POINT ( 'NONE',  ( -35.62769128460905677, -112.5438815906447729, 3.808975545821551290 ) ) ;
#16156=CARTESIAN_POINT ( 'NONE',  ( -35.50000000000000711, -112.0221129971568104, -0.7553032835231431319 ) ) ;
#16164=CARTESIAN_POINT ( 'NONE',  ( -34.50000000000000000, -112.0140978167138712, 0.5627176474015717078 ) ) ;
#16165=CARTESIAN_POINT ( 'NONE',  ( -37.48437500000004263, -114.9929510916434339, 14.11852480586264846 ) ) ;
#16167=CARTESIAN_POINT ( 'NONE',  ( -35.50000000000000000, -113.9929510916434197, 10.50625754673586876 ) ) ;
#16169=CARTESIAN_POINT ( 'NONE',  ( -34.50000000000000000, -114.9929510916434339, 10.72628538622835670 ) ) ;
#16172=SURFACE_STYLE_USAGE ( .BOTH. , #21234 ) ;
#16177=CARTESIAN_POINT ( 'NONE',  ( -36.12500000000014211, -114.9929510916434339, 13.11852480586264669 ) ) ;
#16178=ORIENTED_EDGE ( 'NONE', *, *, #4206, .F. ) ;
#16179=CARTESIAN_POINT ( 'NONE',  ( -36.94073759706868287, -112.0000000000000142, 8.628524454178448266 ) ) ;
#16188=CARTESIAN_POINT ( 'NONE',  ( -36.94073759706868287, -116.9999999999999858, 2.871475545821551290 ) ) ;
#16199=CARTESIAN_POINT ( 'NONE',  ( -34.50000000000000000, -112.8832452823708792, -2.621568770093253953 ) ) ;
#16202=CARTESIAN_POINT ( 'NONE',  ( -35.50000000000000711, -114.9929510916434339, 10.85830208992344303 ) ) ;
#16203=CARTESIAN_POINT ( 'NONE',  ( -34.50000000000000000, -113.9929510916434339, 12.39849696637031684 ) ) ;
#16208=CARTESIAN_POINT ( 'NONE',  ( -37.99839555572501837, -113.9929510916434339, 12.65937477241749143 ) ) ;
#16209=CARTESIAN_POINT ( 'NONE',  ( -36.24999999999983658, -115.9929510916434481, 13.11852480586264846 ) ) ;
#16221=CARTESIAN_POINT ( 'NONE',  ( -35.50000000000000000, -113.4742757288593964, 0.9301473394660054739 ) ) ;
#16225=CARTESIAN_POINT ( 'NONE',  ( -35.50000000000000711, -114.9929510916434339, 10.51175824272318415 ) ) ;
#16230=CARTESIAN_POINT ( 'NONE',  ( -35.50000000000000000, -111.0360125565790383, 1.176611260687384419 ) ) ;
#16233=CARTESIAN_POINT ( 'NONE',  ( -37.88768952767750164, -115.9754527089670262, 1.972274454178448710 ) ) ;
#16240=CARTESIAN_POINT ( 'NONE',  ( -34.50000000000000000, -113.0140978167139991, -0.6247823525984269599 ) ) ;
#16245=CARTESIAN_POINT ( 'NONE',  ( -35.50000000000000000, -113.9929510916434339, 10.85830208992344303 ) ) ;
#16249=CARTESIAN_POINT ( 'NONE',  ( -34.50000000000000000, -112.0154707866092707, 0.9357013553229778235 ) ) ;
#16251=CARTESIAN_POINT ( 'NONE',  ( -36.31249999999994316, -115.9929510916434481, 14.11852480586265024 ) ) ;
#16256=CARTESIAN_POINT ( 'NONE',  ( -38.00000000000000711, -115.9929510916434481, 10.50625754673587053 ) ) ;
#16279=CARTESIAN_POINT ( 'NONE',  ( -39.02454729103295961, -113.2308352781851539, 7.840225545821551734 ) ) ;
#16301=CARTESIAN_POINT ( 'NONE',  ( -35.61121590948313553, -115.9929510916434481, 14.07058620477040733 ) ) ;
#16302=DIRECTION ( 'NONE',  ( -1.000000000000000000, 0.000000000000000000, 0.000000000000000000 ) ) ;
#16314=CARTESIAN_POINT ( 'NONE',  ( -35.99999999999999289, -113.9407375970686758, 3.996475545821551734 ) ) ;
#16339=CARTESIAN_POINT ( 'NONE',  ( -34.50000000000000000, -112.0269151300720409, -0.7876962586524208776 ) ) ;
#16341=CARTESIAN_POINT ( 'NONE',  ( -38.69949915733018742, -114.9929510916434339, 13.54034599209165712 ) ) ;
#16344=CARTESIAN_POINT ( 'NONE',  ( -37.99999897736218202, -114.9929510916434339, 12.62466071271732915 ) ) ;
#16346=CARTESIAN_POINT ( 'NONE',  ( -34.50000000000000000, -114.9929510916434339, 12.57451923796416082 ) ) ;
#16357=CARTESIAN_POINT ( 'NONE',  ( -34.97545270896703329, -113.2308352781851539, 7.409774454178451819 ) ) ;
#16367=CARTESIAN_POINT ( 'NONE',  ( -37.05926240293131713, -111.0000000000000284, 3.621475545821551734 ) ) ;
#16378=CARTESIAN_POINT ( 'NONE',  ( -34.50000000000000000, -114.5974311500472567, -2.624782352598442614 ) ) ;
#16381=CARTESIAN_POINT ( 'NONE',  ( -35.50000000000000711, -114.6604609523327838, 9.751889438017201428 ) ) ;
#16385=CARTESIAN_POINT ( 'NONE',  ( -35.98977351030467986, -113.9929510916434339, 14.11852173794918563 ) ) ;
#16389=CARTESIAN_POINT ( 'NONE',  ( -34.50000000000000000, -113.9929510916436470, 10.50625754673586876 ) ) ;
#16392=CARTESIAN_POINT ( 'NONE',  ( -35.50000000000000711, -114.1302255537607095, 9.515717283514957714 ) ) ;
#16404=CARTESIAN_POINT ( 'NONE',  ( -35.50000000000000000, -113.0140978167138712, 0.8752176474013583229 ) ) ;
#16406=CARTESIAN_POINT ( 'NONE',  ( -37.74901162816869515, -114.6652019342044042, 5.066024454178449155 ) ) ;
#16407=CARTESIAN_POINT ( 'NONE',  ( -35.50025087934803736, -114.9929510916434339, 12.63488142334835196 ) ) ;
#16412=CARTESIAN_POINT ( 'NONE',  ( -35.50000000000000000, -111.0278007905855588, 1.116632271043183078 ) ) ;
#16415=CARTESIAN_POINT ( 'NONE',  ( -36.94073759706868287, -112.0000000000000142, 7.128524454178449155 ) ) ;
#16421=CARTESIAN_POINT ( 'NONE',  ( -34.50000000000000000, -113.0140978167139991, -0.6091573525984278481 ) ) ;
#16428=CARTESIAN_POINT ( 'NONE',  ( -35.50000000000000000, -113.9929510916434339, 10.50625754673609258 ) ) ;
#16431=CARTESIAN_POINT ( 'NONE',  ( -34.50000000000000000, -111.0141129414446652, 0.9205922128478062350 ) ) ;
#16432=CARTESIAN_POINT ( 'NONE',  ( -35.50000000000000000, -114.2600084737790809, 8.524153227862690585 ) ) ;
#16440=CARTESIAN_POINT ( 'NONE',  ( -38.00000000000000711, -115.9929510916434481, 12.57451923796417681 ) ) ;
#16463=CARTESIAN_POINT ( 'NONE',  ( -36.11231047232249125, -115.9754527089670262, 5.777725545821551734 ) ) ;
#16482=( BOUNDED_CURVE ( )  B_SPLINE_CURVE ( 2, ( #17613, #1248, #31138, #20304, #12231, #11687, #6640, #6292, #23022, #3604, #31312, #28971, #34022, #28622, #23385, #6466, #33649, #25568, #12047, #8982, #17435, #28793, #19948, #17792, #14737, #4319, #4142, #28438, #3782, #704, #25749, #17258, #31661, #15084, #25921, #30959, #3972, #1079, #22844, #9348, #23205, #885, #26096, #34197, #9524, #28262, #20486, #11867, #34384, #14552, #1427, #12405, #33841, #9166, #20130, #31499, #22658, #6822, #9705, #20663, #6993, #17968, #15265, #32549, #34558, #1969, #18152, #7883, #35104, #21383, #34925, #4849, #21551, #34735, #24286, #29514, #2164, #2339, #26637, #12944, #23744 ),
 .UNSPECIFIED., .F., .T. ) 
 B_SPLINE_CURVE_WITH_KNOTS ( ( 3, 2, 2, 2, 2, 2, 2, 2, 2, 2, 2, 2, 2, 2, 2, 2, 2, 2, 2, 2, 2, 2, 2, 2, 2, 2, 2, 2, 2, 2, 2, 2, 2, 2, 2, 2, 2, 2, 2, 2, 3 ),
 ( 0.000000000000000000, 0.02500000000000000139, 0.05000000000000000278, 0.07499999999999999722, 0.1000000000000000056, 0.1250000000000000000, 0.1499999999999999944, 0.1749999999999999889, 0.2000000000000000111, 0.2250000000000000056, 0.2500000000000000000, 0.2750000000000000222, 0.2999999999999999889, 0.3250000000000000111, 0.3499999999999999778, 0.3750000000000000000, 0.4000000000000000222, 0.4249999999999999889, 0.4500000000000000111, 0.4749999999999999778, 0.5000000000000000000, 0.5250000000000000222, 0.5500000000000000444, 0.5749999999999999556, 0.5999999999999999778, 0.6250000000000000000, 0.6500000000000000222, 0.6750000000000000444, 0.6999999999999999556, 0.7249999999999999778, 0.7500000000000000000, 0.7750000000000000222, 0.8000000000000000444, 0.8249999999999999556, 0.8499999999999999778, 0.8750000000000000000, 0.9000000000000000222, 0.9250000000000000444, 0.9499999999999999556, 0.9749999999999999778, 1.000000000000000000 ),
 .UNSPECIFIED. ) 
 CURVE ( )  GEOMETRIC_REPRESENTATION_ITEM ( )  RATIONAL_B_SPLINE_CURVE ( ( 1.000000000000000000, 0.9238795325112867385, 1.000000000000000000, 0.9238795325112867385, 1.000000000000000000, 0.9238795325112867385, 1.000000000000000000, 0.9238795325112867385, 1.000000000000000000, 0.9238795325112867385, 1.000000000000000000, 0.9238795325112867385, 1.000000000000000000, 0.9238795325112867385, 1.000000000000000000, 0.9238795325112867385, 1.000000000000000000, 0.9238795325112867385, 1.000000000000000000, 0.9238795325112867385, 1.000000000000000000, 0.9238795325112867385, 1.000000000000000000, 0.9238795325112867385, 1.000000000000000000, 0.9238795325112867385, 1.000000000000000000, 0.9238795325112867385, 1.000000000000000000, 0.9238795325112867385, 1.000000000000000000, 0.9238795325112867385, 1.000000000000000000, 0.9238795325112867385, 1.000000000000000000, 0.9238795325112867385, 1.000000000000000000, 0.9238795325112867385, 1.000000000000000000, 0.9238795325112867385, 1.000000000000000000, 0.9238795325112867385, 1.000000000000000000, 0.9238795325112867385, 1.000000000000000000, 0.9238795325112867385, 1.000000000000000000, 0.9238795325112867385, 1.000000000000000000, 0.9238795325112867385, 1.000000000000000000, 0.9238795325112867385, 1.000000000000000000, 0.9238795325112867385, 1.000000000000000000, 0.9238795325112867385, 1.000000000000000000, 0.9238795325112867385, 1.000000000000000000, 0.9238795325112867385, 1.000000000000000000, 0.9238795325112867385, 1.000000000000000000, 0.9238795325112867385, 1.000000000000000000, 0.9238795325112867385, 1.000000000000000000, 0.9238795325112867385, 1.000000000000000000, 0.9238795325112867385, 1.000000000000000000, 0.9238795325112867385, 1.000000000000000000, 0.9238795325112867385, 1.000000000000000000, 0.9238795325112867385, 1.000000000000000000, 0.9238795325112867385, 1.000000000000000000, 0.9238795325112867385, 1.000000000000000000 ) ) 
 REPRESENTATION_ITEM ( '' )  );
#16485=CARTESIAN_POINT ( 'NONE',  ( -38.99879592093640213, -115.9929510916434481, 12.67985367974111277 ) ) ;
#16496=CARTESIAN_POINT ( 'NONE',  ( -35.99999999999999289, -113.9407375970686758, 2.496475545821551290 ) ) ;
#16529=CARTESIAN_POINT ( 'NONE',  ( -34.50000000000000000, -112.0140978167138712, 0.3752176474015640473 ) ) ;
#16531=CARTESIAN_POINT ( 'NONE',  ( -37.51022648969539119, -114.9929510916434339, 14.11852173794918386 ) ) ;
#16532=CARTESIAN_POINT ( 'NONE',  ( -35.50000000000000000, -113.9929510916433912, 10.50625754673588474 ) ) ;
#16534=ADVANCED_FACE ( 'NONE', ( #9396 ), #20154, .F. ) ;
#16535=CARTESIAN_POINT ( 'NONE',  ( -35.75562914091914024, -114.9929510916434339, 14.09929883582542409 ) ) ;
#16547=CARTESIAN_POINT ( 'NONE',  ( -34.00000000000000000, -114.0592624029313242, 4.503524454178447378 ) ) ;
#16555=CARTESIAN_POINT ( 'NONE',  ( -36.94073759706866156, -111.0000000000000284, 8.628524454178448266 ) ) ;
#16570=CARTESIAN_POINT ( 'NONE',  ( -35.50000000000000000, -112.1946304249441795, 2.703640693953100804 ) ) ;
#16575=CARTESIAN_POINT ( 'NONE',  ( -37.46093750000000711, -114.9929510916434339, 13.11852480586264669 ) ) ;
#16576=CARTESIAN_POINT ( 'NONE',  ( -35.51674767832922441, -113.9929510916434339, 14.04194344061634325 ) ) ;
#16580=CARTESIAN_POINT ( 'NONE',  ( -34.50000000000000000, -113.9929510916433344, 10.50625754673586876 ) ) ;
#16582=CARTESIAN_POINT ( 'NONE',  ( -38.00000000000000711, -115.9929510916434481, 10.85830208992306822 ) ) ;
#16593=CARTESIAN_POINT ( 'NONE',  ( -35.50000000000000711, -115.1770117227680998, -1.611965039240062181 ) ) ;
#16595=CARTESIAN_POINT ( 'NONE',  ( -37.35495115944176092, -112.9754527089670688, 5.534774454178449155 ) ) ;
#16601=CARTESIAN_POINT ( 'NONE',  ( -35.50000000000000000, -117.0140978167138854, -0.5622823525984408377 ) ) ;
#16604=CARTESIAN_POINT ( 'NONE',  ( -36.23083527818512550, -116.0245472910329880, 7.784774454178451819 ) ) ;
#16611=CARTESIAN_POINT ( 'NONE',  ( -34.50000000000000000, -112.0140978167138712, 0.3752176474015640473 ) ) ;
#16614=CARTESIAN_POINT ( 'NONE',  ( -35.50000000000000000, -113.9929510916434339, 12.57451923796416260 ) ) ;
#16618=CARTESIAN_POINT ( 'NONE',  ( -34.50000000000000000, -111.0140978167138570, 0.2502176474015764263 ) ) ;
#16619=CARTESIAN_POINT ( 'NONE',  ( -37.62254989966453422, -115.9929510916434481, 14.11371147303758278 ) ) ;
#16625=CARTESIAN_POINT ( 'NONE',  ( -35.50000000000000711, -114.1489256397697289, 9.518467544735724317 ) ) ;
#16644=CARTESIAN_POINT ( 'NONE',  ( -36.33479806579560289, -113.2509883718313262, 5.308975545821551734 ) ) ;
#16652=CARTESIAN_POINT ( 'NONE',  ( -35.50000000000000711, -114.0743172650041686, 9.508870970061893857 ) ) ;
#16655=CARTESIAN_POINT ( 'NONE',  ( -35.51674767832921731, -114.9929510916434339, 14.04194344061634503 ) ) ;
#16661=CARTESIAN_POINT ( 'NONE',  ( -39.00000000000000000, -115.9929510916434481, 12.57451923796417681 ) ) ;
#16670=CARTESIAN_POINT ( 'NONE',  ( -36.94073759706868287, -115.9999999999999858, 8.871475545821551734 ) ) ;
#16674=EDGE_LOOP ( 'NONE', ( #33476, #34884, #1326, #25946, #24066 ) ) ;
#16697=CARTESIAN_POINT ( 'NONE',  ( -34.50000000000000000, -112.0140978167138712, 0.0002176474015661141945 ) ) ;
#16698=CARTESIAN_POINT ( 'NONE',  ( -37.88878409051687868, -114.9929510916434339, 14.07058620477052102 ) ) ;
#16699=CARTESIAN_POINT ( 'NONE',  ( -35.50000000000000000, -113.9929510916434339, 10.50763272073269405 ) ) ;
#16702=CARTESIAN_POINT ( 'NONE',  ( -34.50000000000000000, -114.9929510916434339, 12.59102132592610523 ) ) ;
#16714=CARTESIAN_POINT ( 'NONE',  ( -40.02454729103296671, -115.1833782841879525, 3.659774454178448710 ) ) ;
#16716=CARTESIAN_POINT ( 'NONE',  ( -35.50000000000000711, -113.1807644833805426, -1.624782352598427959 ) ) ;
#16725=CARTESIAN_POINT ( 'NONE',  ( -35.00000000000000000, -114.0592624029316369, 9.003524454178483793 ) ) ;
#16737=CARTESIAN_POINT ( 'NONE',  ( -34.50000000000000000, -117.0140978167138854, 0.8752176474015623819 ) ) ;
#16741=CARTESIAN_POINT ( 'NONE',  ( -35.51597953369718397, -114.9929510916434339, 12.74811950270164473 ) ) ;
#16742=CARTESIAN_POINT ( 'NONE',  ( -37.24999999999992184, -113.9929510916434339, 14.11852480586265024 ) ) ;
#16745=CARTESIAN_POINT ( 'NONE',  ( -34.50000000000000000, -113.9929510916434339, 10.85830208992344303 ) ) ;
#16746=CARTESIAN_POINT ( 'NONE',  ( -38.92341863475394348, -114.9929510916434339, 13.10177712753322155 ) ) ;
#16748=CARTESIAN_POINT ( 'NONE',  ( -38.00000000000000711, -115.9929510916434481, 11.91443571948719615 ) ) ;
#16762=CARTESIAN_POINT ( 'NONE',  ( -35.50000000000000711, -115.8878449012421754, -1.128496220799388494 ) ) ;
#16764=CARTESIAN_POINT ( 'NONE',  ( -37.97545270896701908, -113.5265240346955977, 8.347274454178448266 ) ) ;
#16770=CARTESIAN_POINT ( 'NONE',  ( -35.50000000000000711, -113.0106174888879877, 1.881901162060937827 ) ) ;
#16773=CARTESIAN_POINT ( 'NONE',  ( -38.45611840935523418, -115.3723087153909432, 5.066024454178449155 ) ) ;
#16779=CARTESIAN_POINT ( 'NONE',  ( -34.50000000000000000, -115.0140978167137860, -0.6411448143358557950 ) ) ;
#16785=CARTESIAN_POINT ( 'NONE',  ( -35.50000000000000000, -113.9929510916434339, 10.56126450660895699 ) ) ;
#16788=CARTESIAN_POINT ( 'NONE',  ( -34.50000000000000000, -111.8727710936879589, 2.535339294948415922 ) ) ;
#16790=CARTESIAN_POINT ( 'NONE',  ( -35.50000000000000000, -114.2114213871176958, 8.518137620934190579 ) ) ;
#16816=CARTESIAN_POINT ( 'NONE',  ( -36.94073759706868287, -115.0000000000000000, 2.871475545821551290 ) ) ;
#16832=CARTESIAN_POINT ( 'NONE',  ( -34.50000000000000000, -114.9922651054798308, 10.46846006712531008 ) ) ;
#16835=UNCERTAINTY_MEASURE_WITH_UNIT (LENGTH_MEASURE( 1.000000000000000082E-05 ), #29362, 'distance_accuracy_value', 'NONE');
#16837=CARTESIAN_POINT ( 'NONE',  ( -35.90191880024782023, -115.9929510916434481, 14.11551573851449071 ) ) ;
#16846=CARTESIAN_POINT ( 'NONE',  ( -38.97545270896704039, -114.8876895276775087, 9.152725545821555286 ) ) ;
#16864=AXIS2_PLACEMENT_3D ( 'NONE', #7505, #28945, #24093 ) ;
#16873=CARTESIAN_POINT ( 'NONE',  ( -39.00000000000000711, -114.9929510916434339, 11.21034663311206181 ) ) ;
#16877=CARTESIAN_POINT ( 'NONE',  ( -34.50000000000000000, -114.9929510916434339, 12.39849696637031506 ) ) ;
#16887=CARTESIAN_POINT ( 'NONE',  ( -39.16322519054179452, -116.0794154965774823, 8.066024454178448266 ) ) ;
#16889=CARTESIAN_POINT ( 'NONE',  ( -35.50000000000000711, -114.6807644833805000, -1.624782352598427959 ) ) ;
#16906=CARTESIAN_POINT ( 'NONE',  ( -35.50000000000000000, -111.1014359431343905, 1.472195201997948510 ) ) ;
#16908=CARTESIAN_POINT ( 'NONE',  ( -36.99999999999989342, -114.9929510916434339, 13.11852480586264669 ) ) ;
#16910=CARTESIAN_POINT ( 'NONE',  ( -36.07812499999994316, -113.9929510916434339, 14.11852480586265024 ) ) ;
#16915=CARTESIAN_POINT ( 'NONE',  ( -34.50120407906360498, -113.9929510916434339, 12.67985367974112343 ) ) ;
#16917=CARTESIAN_POINT ( 'NONE',  ( -35.50000000000000711, -114.0650276068786582, 9.507762098804159123 ) ) ;
#16931=CARTESIAN_POINT ( 'NONE',  ( -35.50000000000000000, -115.0140978167138712, -0.6247823525983134951 ) ) ;
#16933=CARTESIAN_POINT ( 'NONE',  ( -38.37230871539094323, -112.5438815906447729, 2.441024454178448710 ) ) ;
#16939=CARTESIAN_POINT ( 'NONE',  ( -35.50000000000000000, -117.0140978167138854, -0.1247823525984438492 ) ) ;
#16942=CARTESIAN_POINT ( 'NONE',  ( -35.02454729103298803, -114.8876895276775087, 6.097274454178449155 ) ) ;
#16947=CARTESIAN_POINT ( 'NONE',  ( -34.50000000000000000, -112.9876085932806262, 1.879154677457530065 ) ) ;
#16957=CARTESIAN_POINT ( 'NONE',  ( -35.51597953369717686, -113.9929510916434339, 12.74811950270164473 ) ) ;
#16962=CARTESIAN_POINT ( 'NONE',  ( -34.50000000000000000, -111.2304026862503719, 1.811733666967775713 ) ) ;
#16963=CARTESIAN_POINT ( 'NONE',  ( -35.50000000000000000, -114.3049001878960240, 8.530677542735578101 ) ) ;
#16976=CARTESIAN_POINT ( 'NONE',  ( -35.50000000000000711, -113.1256619669233885, 1.895633585076891947 ) ) ;
#16988=CARTESIAN_POINT ( 'NONE',  ( -37.74901162816868805, -113.3347980657955958, 3.433975545821550845 ) ) ;
#17000=CARTESIAN_POINT ( 'NONE',  ( -35.50000000000000711, -114.4026847875275337, 9.592046023459676718 ) ) ;
#17006=CARTESIAN_POINT ( 'NONE',  ( -34.50000000000000000, -114.1414532730574507, 9.517316564499758158 ) ) ;
#17009=CARTESIAN_POINT ( 'NONE',  ( -35.50000000000000000, -114.2356323198232673, 8.521029492159460261 ) ) ;
#17010=CARTESIAN_POINT ( 'NONE',  ( -35.50000000000000711, -113.8159288351371714, 1.978028123174813802 ) ) ;
#17020=CARTESIAN_POINT ( 'NONE',  ( -37.74901162816868805, -113.3347980657955958, 3.433975545821550845 ) ) ;
#17031=CIRCLE ( 'NONE', #10735, 0.5000000000000004441 ) ;
#17050=CARTESIAN_POINT ( 'NONE',  ( -34.50000000000000000, -115.0140978167138428, -0.6247823525986679893 ) ) ;
#17053=CARTESIAN_POINT ( 'NONE',  ( -34.50000000000000000, -115.9929492010520846, 10.50058572605509966 ) ) ;
#17056=CARTESIAN_POINT ( 'NONE',  ( -34.50000000000000000, -114.2114213871176958, 8.518137620934190579 ) ) ;
#17069=CARTESIAN_POINT ( 'NONE',  ( -40.02454729103296671, -115.1833782841879525, 8.159774454178448266 ) ) ;
#17071=CARTESIAN_POINT ( 'NONE',  ( -35.50000000000000711, -112.0140978167138712, -0.5622823525984296245 ) ) ;
#17087=CARTESIAN_POINT ( 'NONE',  ( -34.50000000000000000, -117.0140978167138854, -0.3122823525984416704 ) ) ;
#17093=CARTESIAN_POINT ( 'NONE',  ( -36.31249999999995026, -114.9929510916434339, 13.11852480586264669 ) ) ;
#17094=CARTESIAN_POINT ( 'NONE',  ( -38.25557080230232998, -113.9929510916434339, 13.92914543265419525 ) ) ;
#17097=CARTESIAN_POINT ( 'NONE',  ( -34.50000306791346816, -113.9929510916434339, 12.62875129555796150 ) ) ;
#17098=CARTESIAN_POINT ( 'NONE',  ( -39.00000000000000711, -114.9929510916434339, 10.85830208992306822 ) ) ;
#17099=CARTESIAN_POINT ( 'NONE',  ( -35.83891589277640577, -114.9929510916434339, 13.09299768411358222 ) ) ;
#17103=AXIS2_PLACEMENT_3D ( 'NONE', #18171, #4869, #10269 ) ;
#17109=CIRCLE ( 'NONE', #9082, 0.5000000000000004441 ) ;
#17114=CARTESIAN_POINT ( 'NONE',  ( -35.50000000000000000, -115.0140978167139707, -0.6247823525984387283 ) ) ;
#17116=CARTESIAN_POINT ( 'NONE',  ( -36.94073759706866156, -113.0000000000000000, 8.628524454178448266 ) ) ;
#17122=CARTESIAN_POINT ( 'NONE',  ( -35.50000000000000000, -117.0140978167138854, -0.4997823525984417259 ) ) ;
#17126=CARTESIAN_POINT ( 'NONE',  ( -35.62769128460905677, -115.4561184093552413, 6.191024454178448266 ) ) ;
#17131=CARTESIAN_POINT ( 'NONE',  ( -34.50000000000000000, -115.0140978167137860, -0.6247823525984395054 ) ) ;
#17139=CARTESIAN_POINT ( 'NONE',  ( -38.00000068757622529, -113.9929510916434339, 12.61439929482944855 ) ) ;
#17143=CARTESIAN_POINT ( 'NONE',  ( -34.50000000000000000, -111.0140978167138570, 0.8127176474015720409 ) ) ;
#17144=CARTESIAN_POINT ( 'NONE',  ( -39.00000000000000000, -115.9929510916434481, 12.50851088611646311 ) ) ;
#17167=CARTESIAN_POINT ( 'NONE',  ( -37.05926240293131713, -113.0000000000000000, 6.621475545821551734 ) ) ;
#17175=CARTESIAN_POINT ( 'NONE',  ( -35.50000000000000711, -115.0795240838853886, -1.623175561345890472 ) ) ;
#17178=CARTESIAN_POINT ( 'NONE',  ( -35.50000000000000711, -114.9912366357066986, 10.44580456020104720 ) ) ;
#17182=CARTESIAN_POINT ( 'NONE',  ( -34.50000000000000000, -114.9927795562974069, 10.48735431211914815 ) ) ;
#17187=CARTESIAN_POINT ( 'NONE',  ( -35.50000000000000000, -114.2675000158779710, 8.525177020294046670 ) ) ;
#17188=CARTESIAN_POINT ( 'NONE',  ( -35.50000000000000711, -112.5103839485166333, -1.498529437127682495 ) ) ;
#17198=CARTESIAN_POINT ( 'NONE',  ( -38.02454729103295961, -113.6450488405582462, 9.340225545821551734 ) ) ;
#17208=CARTESIAN_POINT ( 'NONE',  ( -39.97545270896702618, -115.3019030900506152, 4.652725545821551734 ) ) ;
#17215=CARTESIAN_POINT ( 'NONE',  ( -34.50000000000000000, -112.0157046079661995, -0.6902086197697556713 ) ) ;
#17225=CARTESIAN_POINT ( 'NONE',  ( -34.50000000000000000, -114.9932644833805426, -0.6247823525982824089 ) ) ;
#17228=CARTESIAN_POINT ( 'NONE',  ( -34.50000000000000000, -114.2207110452431635, 8.519246492191951958 ) ) ;
#17232=CARTESIAN_POINT ( 'NONE',  ( -34.50000000000000000, -114.2899554544714960, 8.528375582263644006 ) ) ;
#17244=CARTESIAN_POINT ( 'NONE',  ( -39.97545270896702618, -112.6980969099493990, 8.347274454178448266 ) ) ;
#17246=CARTESIAN_POINT ( 'NONE',  ( -35.50000000000000711, -112.3995503592287690, -1.424448457485529618 ) ) ;
#17258=CARTESIAN_POINT ( 'NONE',  ( -35.02454729103298092, -113.1123104723225055, 5.402725545821551734 ) ) ;
#17265=CARTESIAN_POINT ( 'NONE',  ( -35.50000000000000000, -111.0140978167138570, 0.0002176474015660057743 ) ) ;
#17270=CARTESIAN_POINT ( 'NONE',  ( -35.50000000000000711, -114.9929510916434339, 12.53051367006571581 ) ) ;
#17271=CARTESIAN_POINT ( 'NONE',  ( -38.99999693208653895, -113.9929510916434339, 12.62875129555797749 ) ) ;
#17274=CARTESIAN_POINT ( 'NONE',  ( -35.97545865737298953, -113.9929510916434339, 14.11837420659365527 ) ) ;
#17276=CARTESIAN_POINT ( 'NONE',  ( -35.49999931242378892, -114.9929510916434339, 12.61439929482945566 ) ) ;
#17283=CARTESIAN_POINT ( 'NONE',  ( -35.50000000000000711, -114.9492820284331742, 10.20776876943783940 ) ) ;
#17291=CARTESIAN_POINT ( 'NONE',  ( -35.50000000000000000, -113.0140978167139991, -0.6091573525984278481 ) ) ;
#17293=CARTESIAN_POINT ( 'NONE',  ( -35.62769128460905677, -115.4561184093552413, 1.691024454178448710 ) ) ;
#17298=CARTESIAN_POINT ( 'NONE',  ( -37.76916472181487450, -111.9754527089670404, 5.534774454178449155 ) ) ;
#17300=CARTESIAN_POINT ( 'NONE',  ( -35.50000000000000000, -114.8474311500471572, -2.624782352598442614 ) ) ;
#17307=CARTESIAN_POINT ( 'NONE',  ( -34.50000000000000000, -112.0157046079661995, -0.6902086197697556713 ) ) ;
#17312=CARTESIAN_POINT ( 'NONE',  ( -36.01562499999997158, -113.9929510916434339, 13.11852480586264846 ) ) ;
#17316=CARTESIAN_POINT ( 'NONE',  ( -35.74814306589956203, -113.9929510916434339, 13.05539834812772781 ) ) ;
#17317=CARTESIAN_POINT ( 'NONE',  ( -35.50000000000000000, -115.9929510916434481, 11.73841344789270202 ) ) ;
#17320=EDGE_CURVE ( 'NONE', #31629, #17346, #20363, .T. ) ;
#17328=CARTESIAN_POINT ( 'NONE',  ( -35.50000000000000711, -113.3557509229967764, 1.923098431109107054 ) ) ;
#17341=CARTESIAN_POINT ( 'NONE',  ( -37.47347596530441649, -113.0245472910329880, 6.527725545821552622 ) ) ;
#17346=VERTEX_POINT ( 'NONE', #15274 ) ;
#17349=CARTESIAN_POINT ( 'NONE',  ( -35.50000000000000711, -116.0140978167138712, -0.1247823525984439463 ) ) ;
#17353=CARTESIAN_POINT ( 'NONE',  ( -35.50000102263782509, -114.9929510916434339, 12.62466071271731316 ) ) ;
#17356=CARTESIAN_POINT ( 'NONE',  ( -34.50000000000000000, -114.1091535596544873, 9.513028657562415447 ) ) ;
#17364=CARTESIAN_POINT ( 'NONE',  ( -35.50000000000000000, -115.9926080209513657, 10.46845107750242398 ) ) ;
#17375=CARTESIAN_POINT ( 'NONE',  ( -37.47347596530441649, -113.0245472910329880, 5.027725545821551734 ) ) ;
#17383=DIRECTION ( 'NONE',  ( -1.000000000000000000, 0.000000000000000000, 0.000000000000000000 ) ) ;
#17385=CARTESIAN_POINT ( 'NONE',  ( -33.97545270896702618, -112.8166217158120475, 8.909774454178450043 ) ) ;
#17401=CARTESIAN_POINT ( 'NONE',  ( -34.50000000000000000, -113.0106174888879877, 1.881901162060937827 ) ) ;
#17405=CARTESIAN_POINT ( 'NONE',  ( -34.50000000000000000, -115.6492853190479337, 9.359470924297957239 ) ) ;
#17410=CARTESIAN_POINT ( 'NONE',  ( -39.00000000000000711, -114.9929510916434339, 12.26648026267477043 ) ) ;
#17421=CARTESIAN_POINT ( 'NONE',  ( -34.92058450342249643, -111.8367748094582197, 3.808975545821551734 ) ) ;
#17423=CARTESIAN_POINT ( 'NONE',  ( -35.50000000000000711, -115.9821387493194891, -0.8839717462762166633 ) ) ;
#17435=CARTESIAN_POINT ( 'NONE',  ( -36.94073759706868287, -115.9999999999999858, 4.371475545821550845 ) ) ;
#17441=CARTESIAN_POINT ( 'NONE',  ( -35.50000000000000000, -111.4147656069378058, -1.853877267569947529 ) ) ;
#17450=CARTESIAN_POINT ( 'NONE',  ( -39.00000000000000000, -113.9929510916434339, 12.56351784598954779 ) ) ;
#17455=CARTESIAN_POINT ( 'NONE',  ( -37.49023442168701337, -113.9929510916434339, 14.11852773550420359 ) ) ;
#17457=CARTESIAN_POINT ( 'NONE',  ( -35.98364338251434447, -114.9929510916434339, 13.11827392651456314 ) ) ;
#17464=CARTESIAN_POINT ( 'NONE',  ( -35.93473953453761283, -114.9929510916434339, 13.11451721564123574 ) ) ;
#17472=CARTESIAN_POINT ( 'NONE',  ( -35.50000000000000000, -115.0140978167138712, -0.6247823525984403936 ) ) ;
#17474=CARTESIAN_POINT ( 'NONE',  ( -38.45611840935523418, -115.3723087153909432, 5.066024454178449155 ) ) ;
#17476=CARTESIAN_POINT ( 'NONE',  ( -39.02454729103295961, -114.7691647218148745, 3.659774454178448710 ) ) ;
#17478=CARTESIAN_POINT ( 'NONE',  ( -35.50000000000000711, -112.0140978167138712, 0.6252176474015680441 ) ) ;
#17482=SHAPE_REPRESENTATION_RELATIONSHIP ( 'NONE' , 'NONE' ,  #31216, #30145 ) ;
#17488=CARTESIAN_POINT ( 'NONE',  ( -34.50000000000000000, -115.2732872103912030, -1.592823285204062911 ) ) ;
#17494=CARTESIAN_POINT ( 'NONE',  ( -37.43749999999998579, -113.9929510916434339, 13.11852480586264846 ) ) ;
#17498=CARTESIAN_POINT ( 'NONE',  ( -36.15625000000007816, -113.9929510916434339, 13.11852480586264846 ) ) ;
#17500=CARTESIAN_POINT ( 'NONE',  ( -35.50000000000000000, -115.9920935318519923, 10.44577481630138749 ) ) ;
#17518=CARTESIAN_POINT ( 'NONE',  ( -34.50000000000000000, -117.0140978167138854, -0.4997823525984417259 ) ) ;
#17522=CARTESIAN_POINT ( 'NONE',  ( -37.99999999999998579, -113.9407375970686758, 2.253524454178448710 ) ) ;
#17527=CARTESIAN_POINT ( 'NONE',  ( -35.50000000000000000, -114.5974311500472567, -0.6247823525984269599 ) ) ;
#17529=CARTESIAN_POINT ( 'NONE',  ( -35.50000000000000711, -114.8474311500471572, -1.624782352598427959 ) ) ;
#17531=CARTESIAN_POINT ( 'NONE',  ( -36.06250000000002132, -114.9929510916434339, 13.11852480586264669 ) ) ;
#17535=CARTESIAN_POINT ( 'NONE',  ( -34.50000000000000000, -114.9492820284331742, 10.20776876943783940 ) ) ;
#17541=CARTESIAN_POINT ( 'NONE',  ( -35.50000000000000000, -114.2450133963102843, 8.522190569412378736 ) ) ;
#17542=CARTESIAN_POINT ( 'NONE',  ( -35.50000000000000711, -112.7765286249690035, 1.847058736912741583 ) ) ;
#17552=CARTESIAN_POINT ( 'NONE',  ( -36.25098837183130485, -114.6652019342044184, 5.683975545821551734 ) ) ;
#17560=CARTESIAN_POINT ( 'NONE',  ( -36.94073759706868287, -116.9999999999999858, 5.871475545821551734 ) ) ;
#17581=CARTESIAN_POINT ( 'NONE',  ( -34.50000000000000000, -115.0140978167138712, -0.6247823525984418369 ) ) ;
#17583=CARTESIAN_POINT ( 'NONE',  ( -34.50000000000000000, -115.7766462221073454, 9.569741527169023598 ) ) ;
#17586=CARTESIAN_POINT ( 'NONE',  ( -39.00000000000000711, -114.9929510916434339, 12.59102132592608925 ) ) ;
#17594=CARTESIAN_POINT ( 'NONE',  ( -35.69809690994941320, -116.9754527089670546, 4.277725545821552622 ) ) ;
#17598=CARTESIAN_POINT ( 'NONE',  ( -35.50000000000000000, -113.0140978167138712, -0.3122823525984338988 ) ) ;
#17613=CARTESIAN_POINT ( 'NONE',  ( -35.00000000000000000, -113.9407375970687895, 2.496475545821554398 ) ) ;
#17620=CARTESIAN_POINT ( 'NONE',  ( -35.50000000000000000, -112.7530559548648341, -2.608751991713152307 ) ) ;
#17626=CARTESIAN_POINT ( 'NONE',  ( -37.93687354226506869, -114.9929510916434339, 12.87038173996323565 ) ) ;
#17631=CARTESIAN_POINT ( 'NONE',  ( -34.50000000000000000, -114.0998638248492085, 9.511920366020609308 ) ) ;
#17635=CARTESIAN_POINT ( 'NONE',  ( -37.59808119975203766, -113.9929510916434339, 14.11551573851449071 ) ) ;
#17638=CARTESIAN_POINT ( 'NONE',  ( -35.50005019975638021, -114.9929510916434339, 12.62670525340498529 ) ) ;
#17644=CARTESIAN_POINT ( 'NONE',  ( -35.50000000000000711, -114.9929510916434339, 12.17846912687782712 ) ) ;
#17653=CARTESIAN_POINT ( 'NONE',  ( -35.50000000000000000, -113.0140978167138712, -0.6247823525983134951 ) ) ;
#17656=CARTESIAN_POINT ( 'NONE',  ( -35.54388159064475872, -112.6276912846090568, 7.316024454178449155 ) ) ;
#17659=CARTESIAN_POINT ( 'NONE',  ( -35.02454729103298803, -114.8876895276775087, 4.597274454178448266 ) ) ;
#17664=CARTESIAN_POINT ( 'NONE',  ( -35.50000000000000711, -112.0269151300720409, -0.7876962586524208776 ) ) ;
#17675=CARTESIAN_POINT ( 'NONE',  ( -34.50000000000000000, -113.8814751941374652, 2.992951091643117678 ) ) ;
#17676=CARTESIAN_POINT ( 'NONE',  ( -35.50000000000000711, -113.0796441757086939, 1.890140615870383956 ) ) ;
#17678=PRODUCT_DEFINITION_CONTEXT ( 'detailed design', #34261, 'design' ) ;
#17683=CARTESIAN_POINT ( 'NONE',  ( -35.60016694755736211, -113.9929510916434339, 12.92579853460621386 ) ) ;
#17685=CARTESIAN_POINT ( 'NONE',  ( -35.50640865667917723, -113.9929510916434339, 12.69998175888958691 ) ) ;
#17687=CARTESIAN_POINT ( 'NONE',  ( -35.50000000000000000, -115.9929510916434481, 12.59102132592610346 ) ) ;
#17698=CARTESIAN_POINT ( 'NONE',  ( -35.50000000000000711, -112.9876085932806262, 1.879154677457530065 ) ) ;
#17700=CARTESIAN_POINT ( 'NONE',  ( -35.50000000000000711, -114.0928965812550757, 9.511088712577292270 ) ) ;
#17704=CARTESIAN_POINT ( 'NONE',  ( -34.50000000000000000, -116.9980674558286040, -0.8858242144478970514 ) ) ;
#17708=CARTESIAN_POINT ( 'NONE',  ( -36.52652403469559061, -114.9754527089670262, 8.777725545821549957 ) ) ;
#17715=CARTESIAN_POINT ( 'NONE',  ( -34.50000000000000000, -113.9344536409997630, 0.9850770315317123327 ) ) ;
#17719=CARTESIAN_POINT ( 'NONE',  ( -35.50000000000000711, -114.9929510916434339, 12.53051367006571581 ) ) ;
#17722=CARTESIAN_POINT ( 'NONE',  ( -35.51674767832921731, -114.9929510916434339, 14.04194344061634503 ) ) ;
#17727=CARTESIAN_POINT ( 'NONE',  ( -35.50000000000000000, -115.9929510916434481, 10.94631322572069365 ) ) ;
#17728=CARTESIAN_POINT ( 'NONE',  ( -35.50000000000000711, -112.0140978167138712, -0.4997823525984337878 ) ) ;
#17739=CARTESIAN_POINT ( 'NONE',  ( -35.97545270896705460, -114.3549511594417680, 7.090225545821551734 ) ) ;
#17747=CARTESIAN_POINT ( 'NONE',  ( -33.97545270896703329, -115.1833782841879810, 8.590225545821549957 ) ) ;
#17762=CARTESIAN_POINT ( 'NONE',  ( -34.50000000000000000, -113.0140978167138712, -0.6247823525983134951 ) ) ;
#17765=CARTESIAN_POINT ( 'NONE',  ( -36.62499999999902656, -115.9929510916434481, 14.11852480586265024 ) ) ;
#17768=CARTESIAN_POINT ( 'NONE',  ( -38.81062062679291103, -114.9929510916434339, 13.37409560816442067 ) ) ;
#17777=CARTESIAN_POINT ( 'NONE',  ( -39.16322519054178741, -111.9205845034225177, 6.433975545821551734 ) ) ;
#17779=CARTESIAN_POINT ( 'NONE',  ( -35.50000000000000000, -113.0140978167138712, 0.8752176474015154195 ) ) ;
#17792=CARTESIAN_POINT ( 'NONE',  ( -38.97545270896704039, -114.8876895276775087, 4.652725545821550845 ) ) ;
#17797=CARTESIAN_POINT ( 'NONE',  ( -35.50000000000000000, -111.0301281775997353, -0.8858242144478579716 ) ) ;
#17805=CARTESIAN_POINT ( 'NONE',  ( -34.50000000000000000, -114.1189822439768449, 9.514224058074130852 ) ) ;
#17810=CARTESIAN_POINT ( 'NONE',  ( -37.24999999999992184, -113.9929510916434339, 14.11852480586265024 ) ) ;
#17813=CARTESIAN_POINT ( 'NONE',  ( -36.87500000000098055, -114.9929510916434339, 13.11852480586264669 ) ) ;
#17820=CARTESIAN_POINT ( 'NONE',  ( -35.49999931242378892, -114.9929510916434339, 12.61439929482945566 ) ) ;
#17823=CARTESIAN_POINT ( 'NONE',  ( -35.62769128460905677, -115.4561184093552413, 3.191024454178449155 ) ) ;
#17827=CARTESIAN_POINT ( 'NONE',  ( -34.50000000000000000, -113.0140978167138712, 0.8127176474015720409 ) ) ;
#17829=CARTESIAN_POINT ( 'NONE',  ( -39.02454729103295961, -114.7691647218148745, 6.659774454178450043 ) ) ;
#17832=CARTESIAN_POINT ( 'NONE',  ( -38.97545270896704039, -113.1123104723225197, 5.347274454178449155 ) ) ;
#17836=CARTESIAN_POINT ( 'NONE',  ( -35.50000000000000711, -112.7549084230351752, -1.592823285203595285 ) ) ;
#17842=( LENGTH_UNIT ( ) NAMED_UNIT ( * ) SI_UNIT ( .MILLI., .METRE. ) );
#17846=CARTESIAN_POINT ( 'NONE',  ( -34.50000000000000000, -112.5103839485166333, -1.498529437127682495 ) ) ;
#17853=CARTESIAN_POINT ( 'NONE',  ( -37.99999897736217491, -113.9929510916434339, 12.62466071271733092 ) ) ;
#17858=CARTESIAN_POINT ( 'NONE',  ( -35.50000000000000000, -113.9929510916434339, 12.50851088611648265 ) ) ;
#17859=CARTESIAN_POINT ( 'NONE',  ( -35.50400759022158326, -115.9929510916434481, 12.68378527132497524 ) ) ;
#17871=CARTESIAN_POINT ( 'NONE',  ( -35.50000000000000711, -113.4307644833805000, -1.624782352598427959 ) ) ;
#17879=CARTESIAN_POINT ( 'NONE',  ( -34.50000000000000000, -116.6134300264884445, -1.853877267570539944 ) ) ;
#17884=CARTESIAN_POINT ( 'NONE',  ( -37.35495115944176803, -115.0245472910329880, 8.965225545821551734 ) ) ;
#17888=CARTESIAN_POINT ( 'NONE',  ( -35.50000000000000000, -115.0140978167143402, -0.6247823525984417259 ) ) ;
#17896=CARTESIAN_POINT ( 'NONE',  ( -35.50000000000000711, -114.9929510916434339, 12.39849696637031506 ) ) ;
#17899=CARTESIAN_POINT ( 'NONE',  ( -36.15625000000007816, -114.9929510916434339, 14.11852480586264846 ) ) ;
#17905=CARTESIAN_POINT ( 'NONE',  ( -35.50000000000000000, -115.9929510916434481, 12.17846912687782712 ) ) ;
#17906=CARTESIAN_POINT ( 'NONE',  ( -35.50000000000000711, -116.0140896356112989, -0.6575071456984549201 ) ) ;
#17918=CARTESIAN_POINT ( 'NONE',  ( -37.99999999999998579, -114.0592624029313242, 4.746475545821549957 ) ) ;
#17925=ORIENTED_EDGE ( 'NONE', *, *, #20497, .T. ) ;
#17926=CARTESIAN_POINT ( 'NONE',  ( -34.02454729103297382, -112.6980969099494132, 9.902725545821553510 ) ) ;
#17943=CARTESIAN_POINT ( 'NONE',  ( -34.50000000000000000, -115.9929510916434481, 12.59652202191340464 ) ) ;
#17945=CARTESIAN_POINT ( 'NONE',  ( -37.76916472181487450, -111.9754527089670404, 2.534774454178448710 ) ) ;
#17946=CARTESIAN_POINT ( 'NONE',  ( -34.50000000000000000, -115.9874658933321001, 10.35517832894335832 ) ) ;
#17955=CARTESIAN_POINT ( 'NONE',  ( -40.02454729103296671, -112.8166217158120332, 4.840225545821551734 ) ) ;
#17957=CARTESIAN_POINT ( 'NONE',  ( -35.50000000000000000, -113.0140978167138712, 0.2502176474015764263 ) ) ;
#17963=ORIENTED_EDGE ( 'NONE', *, *, #8111, .F. ) ;
#17968=CARTESIAN_POINT ( 'NONE',  ( -36.23083527818513261, -111.9754527089670404, 8.215225545821549957 ) ) ;
#17974=CARTESIAN_POINT ( 'NONE',  ( -35.50000000000000000, -117.0140978167138854, -0.4997823525984417259 ) ) ;
#17981=CARTESIAN_POINT ( 'NONE',  ( -38.00000000000000711, -114.9929510916434339, 12.39849696637031151 ) ) ;
#17983=CARTESIAN_POINT ( 'NONE',  ( -34.50000000000000000, -114.9929296450195721, 10.49869535309826674 ) ) ;
#17986=CARTESIAN_POINT ( 'NONE',  ( -37.62959469683911351, -114.9929510916434339, 13.10254527216511633 ) ) ;
#17989=CARTESIAN_POINT ( 'NONE',  ( -37.52454134262689678, -113.9929510916434339, 14.11837420659362152 ) ) ;
#17997=CARTESIAN_POINT ( 'NONE',  ( -35.83891589277640577, -114.9929510916434339, 13.09299768411358222 ) ) ;
#18005=CARTESIAN_POINT ( 'NONE',  ( -34.50000000000000000, -113.0140978167139991, -0.6091573525984278481 ) ) ;
#18009=CARTESIAN_POINT ( 'NONE',  ( -38.37230871539094323, -112.5438815906447729, 5.441024454178449155 ) ) ;
#18013=CARTESIAN_POINT ( 'NONE',  ( -35.50000000000000711, -114.5974311500472425, -1.624782352598427959 ) ) ;
#18022=CARTESIAN_POINT ( 'NONE',  ( -34.50000000000000000, -113.5133328644208746, 2.949007337991939259 ) ) ;
#18023=CARTESIAN_POINT ( 'NONE',  ( -35.50000000000000711, -112.0140900043112282, 0.8439677466545482121 ) ) ;
#18031=CARTESIAN_POINT ( 'NONE',  ( -38.00000000000000711, -113.9929510916434339, 12.50851088611646311 ) ) ;
#18034=CARTESIAN_POINT ( 'NONE',  ( -35.50000000000000000, -113.9929510916434339, 11.21034663311132107 ) ) ;
#18036=CARTESIAN_POINT ( 'NONE',  ( -35.50000000000000000, -115.9710363517788068, 10.20486393345008835 ) ) ;
#18047=CARTESIAN_POINT ( 'NONE',  ( -35.50000000000000711, -113.1807644833805426, -1.624782352598427959 ) ) ;
#18055=CARTESIAN_POINT ( 'NONE',  ( -35.50000000000000000, -113.5133328644208746, 2.949007337991939259 ) ) ;
#18059=CARTESIAN_POINT ( 'NONE',  ( -37.99999999999998579, -113.9407375970686758, 5.253524454178449155 ) ) ;
#18062=CARTESIAN_POINT ( 'NONE',  ( -35.50000000000000000, -114.3474311500471572, -0.6247823525984269599 ) ) ;
#18071=CARTESIAN_POINT ( 'NONE',  ( -36.00585935943767169, -114.9929510916434339, 13.11852578240983291 ) ) ;
#18074=CARTESIAN_POINT ( 'NONE',  ( -34.80050084267117683, -114.9929510916434339, 13.54034599209289169 ) ) ;
#18078=CARTESIAN_POINT ( 'NONE',  ( -35.51597953369717686, -115.9929510916434481, 12.74811950270164473 ) ) ;
#18079=CARTESIAN_POINT ( 'NONE',  ( -35.50000000000000711, -115.3362660311619692, -1.573728109101206085 ) ) ;
#18091=CARTESIAN_POINT ( 'NONE',  ( -36.52652403469556930, -113.0245472910329880, 4.222274454178449155 ) ) ;
#18102=CARTESIAN_POINT ( 'NONE',  ( -36.11231047232249125, -115.9754527089670262, 2.777725545821550845 ) ) ;
#18123=CARTESIAN_POINT ( 'NONE',  ( -34.50000000000000000, -115.9929510916434481, 12.50851088611648265 ) ) ;
#18125=CARTESIAN_POINT ( 'NONE',  ( -34.97545270896703329, -113.2308352781851397, 7.409774454178450043 ) ) ;
#18126=CARTESIAN_POINT ( 'NONE',  ( -34.50000000000000000, -115.9929510916434481, 12.57451923796416260 ) ) ;
#18135=CARTESIAN_POINT ( 'NONE',  ( -36.94073759706868287, -116.9999999999999858, 7.371475545821551734 ) ) ;
#18137=CARTESIAN_POINT ( 'NONE',  ( -35.50000000000000000, -113.0140978167137860, -0.6247823525984055326 ) ) ;
#18152=CARTESIAN_POINT ( 'NONE',  ( -35.54388159064475872, -115.3723087153909432, 8.683975545821551734 ) ) ;
#18157=VERTEX_POINT ( 'NONE', #8726 ) ;
#18158=CARTESIAN_POINT ( 'NONE',  ( -35.50000000000000711, -112.0209493036498287, 0.9959249592223760050 ) ) ;
#18164=CARTESIAN_POINT ( 'NONE',  ( -38.00000000000000711, -114.9929510916434339, 12.50851088611646311 ) ) ;
#18166=CARTESIAN_POINT ( 'NONE',  ( -34.50000000000000000, -114.9929510916434339, 10.51175824272318415 ) ) ;
#18168=CARTESIAN_POINT ( 'NONE',  ( -37.46874999999996447, -114.9929510916434339, 13.11852480586264669 ) ) ;
#18170=CARTESIAN_POINT ( 'NONE',  ( -34.50000000000000000, -114.9929510916434339, 10.68227981832981044 ) ) ;
#18171=CARTESIAN_POINT ( 'NONE',  ( -35.00000000000000000, -114.0000000000003411, 9.500000000000035527 ) ) ;
#18173=CARTESIAN_POINT ( 'NONE',  ( -37.89983305244309975, -114.9929510916434339, 12.92579853460519246 ) ) ;
#18179=CARTESIAN_POINT ( 'NONE',  ( -37.24999999999992895, -114.9929510916434339, 13.11852480586264669 ) ) ;
#18189=CARTESIAN_POINT ( 'NONE',  ( -34.50000000000000000, -113.0140978167138712, 0.5627176474015715968 ) ) ;
#18191=CARTESIAN_POINT ( 'NONE',  ( -36.11231047232249125, -112.0245472910329880, 8.722274454178448266 ) ) ;
#18193=CARTESIAN_POINT ( 'NONE',  ( -39.99999999999999289, -113.9407375970686758, 2.253524454178448710 ) ) ;
#18197=CARTESIAN_POINT ( 'NONE',  ( -35.50000000000000711, -113.2224311500466030, -1.624782352598427959 ) ) ;
#18206=CARTESIAN_POINT ( 'NONE',  ( -34.50000000000000000, -112.7549084230351752, -1.592823285203595285 ) ) ;
#18215=CARTESIAN_POINT ( 'NONE',  ( -34.50000000000000000, -113.9929510916436470, 10.50625754673581724 ) ) ;
#18217=CARTESIAN_POINT ( 'NONE',  ( -37.54084996655477369, -113.9929510916434339, 13.11692036158760466 ) ) ;
#18218=CARTESIAN_POINT ( 'NONE',  ( -37.43749999999998579, -115.9929510916434481, 13.11852480586264846 ) ) ;
#18230=CARTESIAN_POINT ( 'NONE',  ( -35.50000000000000711, -112.0140978167138712, -0.5622823525984296245 ) ) ;
#18239=CARTESIAN_POINT ( 'NONE',  ( -34.50000000000000000, -111.0301281775997353, -0.8858242144478579716 ) ) ;
#18243=CARTESIAN_POINT ( 'NONE',  ( -35.99999999999999289, -113.9407375970686758, 9.996475545821549957 ) ) ;
#18249=CARTESIAN_POINT ( 'NONE',  ( -35.50000000000000000, -115.0140978167138712, 0.3752176474015736507 ) ) ;
#18253=CARTESIAN_POINT ( 'NONE',  ( -35.50000000000000000, -113.9929510916434339, 10.50625754673586876 ) ) ;
#18257=CARTESIAN_POINT ( 'NONE',  ( -37.59808119975203766, -114.9929510916434339, 14.11551573851448893 ) ) ;
#18261=CARTESIAN_POINT ( 'NONE',  ( -36.24999999999983658, -115.9929510916434481, 13.11852480586264846 ) ) ;
#18262=CARTESIAN_POINT ( 'NONE',  ( -35.50000000000000711, -113.0557643173828524, -1.624792769101735868 ) ) ;
#18277=CARTESIAN_POINT ( 'NONE',  ( -36.33479806579561000, -114.7490116281687165, 3.191024454178448710 ) ) ;
#18287=CARTESIAN_POINT ( 'NONE',  ( -34.83677480945821259, -116.0794154965774965, 5.683975545821551734 ) ) ;
#18292=DIRECTION ( 'NONE',  ( 1.000000000000000000, 0.000000000000000000, 0.000000000000000000 ) ) ;
#18308=CARTESIAN_POINT ( 'NONE',  ( -34.50000000000000000, -115.9929510916434481, 10.94631322572069365 ) ) ;
#18311=CARTESIAN_POINT ( 'NONE',  ( -35.54388159064475872, -112.6276912846090568, 5.816024454178449155 ) ) ;
#18313=CARTESIAN_POINT ( 'NONE',  ( -34.50000000000000000, -115.9929510916434481, 10.55026311463432087 ) ) ;
#18322=CARTESIAN_POINT ( 'NONE',  ( -39.16322519054178741, -111.9205845034225177, 7.933975545821553510 ) ) ;
#18325=CARTESIAN_POINT ( 'NONE',  ( -35.50000000000000711, -116.0140978167138712, 0.3752176474015736507 ) ) ;
#18343=CARTESIAN_POINT ( 'NONE',  ( -35.50000000000000711, -112.0140900043366088, -0.5935324770972457697 ) ) ;
#18349=CARTESIAN_POINT ( 'NONE',  ( -34.50000000000000000, -112.1222502514821144, 1.343475657184566296 ) ) ;
#18351=CARTESIAN_POINT ( 'NONE',  ( -34.50000000000000000, -114.9925223117477202, 10.47601618151863079 ) ) ;
#18354=CARTESIAN_POINT ( 'NONE',  ( -35.51597953369718397, -114.9929510916434339, 12.74811950270164473 ) ) ;
#18356=CARTESIAN_POINT ( 'NONE',  ( -39.00000000000000000, -113.9929510916434339, 11.73841344789285657 ) ) ;
#18365=CARTESIAN_POINT ( 'NONE',  ( -37.53269373325071712, -114.9929510916434339, 13.11752178341324360 ) ) ;
#18368=CARTESIAN_POINT ( 'NONE',  ( -35.00000000000000000, -114.0592624029313242, 6.003524454178450043 ) ) ;
#18375=CARTESIAN_POINT ( 'NONE',  ( -37.05926240293133134, -116.9999999999999858, 3.378524454178448710 ) ) ;
#18380=VERTEX_POINT ( 'NONE', #29749 ) ;
#18386=CARTESIAN_POINT ( 'NONE',  ( -34.50000000000000000, -111.2304026862503719, 1.811733666967775713 ) ) ;
#18393=CARTESIAN_POINT ( 'NONE',  ( -35.50000000000000711, -114.0928965812550757, 9.511088712577292270 ) ) ;
#18395=CARTESIAN_POINT ( 'NONE',  ( -34.50000000000000000, -113.9917898843777522, 10.50611893782865813 ) ) ;
#18398=CARTESIAN_POINT ( 'NONE',  ( -38.00000000000000711, -113.9929510916434339, 12.59652202191340820 ) ) ;
#18399=CARTESIAN_POINT ( 'NONE',  ( -37.50818044754229419, -115.9929510916434481, 13.11847460610629845 ) ) ;
#18410=CARTESIAN_POINT ( 'NONE',  ( -35.50000000000000711, -113.3474311500483935, -1.624782352598427959 ) ) ;
#18414=CARTESIAN_POINT ( 'NONE',  ( -35.50000000000000711, -114.1414532730574507, 9.517316564499758158 ) ) ;
#18418=CARTESIAN_POINT ( 'NONE',  ( -35.50000000000000000, -112.9650106922503170, -2.624765990393421955 ) ) ;
#18422=CARTESIAN_POINT ( 'NONE',  ( -38.97545270896704039, -113.1123104723225197, 3.847274454178449599 ) ) ;
#18426=CARTESIAN_POINT ( 'NONE',  ( -34.50000000000000000, -114.8474311500471572, -0.6247823525984269599 ) ) ;
#18432=CARTESIAN_POINT ( 'NONE',  ( -38.00000000000000711, -114.9929510916434339, 12.59102132592608925 ) ) ;
#18436=CARTESIAN_POINT ( 'NONE',  ( -34.50000000000000000, -112.0140978167138712, 0.8127176474015721519 ) ) ;
#18438=CARTESIAN_POINT ( 'NONE',  ( -35.07817881376918479, -114.9929510916434339, 13.81802396319203297 ) ) ;
#18444=CARTESIAN_POINT ( 'NONE',  ( -36.99999999999988631, -115.9929510916434481, 13.11852480586264846 ) ) ;
#18445=CARTESIAN_POINT ( 'NONE',  ( -35.50000000000000711, -115.0468226098135744, -1.624774171496087716 ) ) ;
#18455=CARTESIAN_POINT ( 'NONE',  ( -36.25098837183129774, -113.3347980657956242, 7.316024454178450043 ) ) ;
#18463=CARTESIAN_POINT ( 'NONE',  ( -38.99999999999999289, -114.0592624029313242, 9.246475545821551734 ) ) ;
#18486=CARTESIAN_POINT ( 'NONE',  ( -35.62769128460905677, -115.4561184093552413, 3.191024454178449155 ) ) ;
#18489=CARTESIAN_POINT ( 'NONE',  ( -34.50000000000000000, -115.9929510916434481, 10.53376102667243508 ) ) ;
#18498=CARTESIAN_POINT ( 'NONE',  ( -35.54388159064475872, -115.3723087153909432, 5.683975545821551734 ) ) ;
#18518=CARTESIAN_POINT ( 'NONE',  ( -35.50000000000000711, -112.0140978167138712, -0.3122823525984337878 ) ) ;
#18526=CARTESIAN_POINT ( 'NONE',  ( -34.50000000000000000, -112.9185811467682754, 1.870920967077121411 ) ) ;
#18527=CARTESIAN_POINT ( 'NONE',  ( -34.50000306791346816, -114.9929510916434339, 12.62875129555796150 ) ) ;
#18529=CARTESIAN_POINT ( 'NONE',  ( -37.49414064056234253, -114.9929510916434339, 13.11852578240983291 ) ) ;
#18531=CARTESIAN_POINT ( 'NONE',  ( -34.50000000000000000, -114.1189822439768449, 9.514224058074130852 ) ) ;
#18534=CARTESIAN_POINT ( 'NONE',  ( -38.00000000000000711, -114.9929510916434339, 12.39849696637031151 ) ) ;
#18541=CARTESIAN_POINT ( 'NONE',  ( -36.03125000000004263, -114.9929510916434339, 13.11852480586264669 ) ) ;
#18545=CARTESIAN_POINT ( 'NONE',  ( -38.45611840935523418, -115.3723087153909432, 8.066024454178448266 ) ) ;
#18551=CARTESIAN_POINT ( 'NONE',  ( -35.00000000000000000, -114.0592624029313242, 7.503524454178449155 ) ) ;
#18565=CARTESIAN_POINT ( 'NONE',  ( -34.50000000000000000, -111.0141129414446652, 0.9205922128478062350 ) ) ;
#18573=CARTESIAN_POINT ( 'NONE',  ( -35.50000000000000711, -114.9902084924877954, 10.43071793783961176 ) ) ;
#18574=CARTESIAN_POINT ( 'NONE',  ( -34.50000000000000000, -113.9929510916434339, 10.51725893871049067 ) ) ;
#18577=CARTESIAN_POINT ( 'NONE',  ( -38.00000000000000711, -113.9929510916434339, 12.60752341388803721 ) ) ;
#18578=CARTESIAN_POINT ( 'NONE',  ( -35.96730626674924025, -115.9929510916434481, 13.11752178341330222 ) ) ;
#18591=CARTESIAN_POINT ( 'NONE',  ( -35.50000000000000711, -112.1403507321855528, -1.128496220798856253 ) ) ;
#18593=CARTESIAN_POINT ( 'NONE',  ( -35.50000000000000711, -114.9929510916434339, 10.59426868253284226 ) ) ;
#18599=CARTESIAN_POINT ( 'NONE',  ( -35.50000000000000000, -111.0397324434303101, -0.9506101647064429949 ) ) ;
#18602=CARTESIAN_POINT ( 'NONE',  ( -35.62769128460905677, -115.4561184093552413, 1.691024454178448710 ) ) ;
#18608=CARTESIAN_POINT ( 'NONE',  ( -34.50000000000000000, -113.0140978167136581, 0.8752176474015690433 ) ) ;
#18613=CARTESIAN_POINT ( 'NONE',  ( -37.46874999999996447, -114.9929510916434339, 13.11852480586264669 ) ) ;
#18617=CARTESIAN_POINT ( 'NONE',  ( -34.50000000000000000, -112.0651520602111191, -0.9469505670458575608 ) ) ;
#18622=CARTESIAN_POINT ( 'NONE',  ( -37.46093750000000711, -115.9929510916434481, 13.11852480586264846 ) ) ;
#18643=CARTESIAN_POINT ( 'NONE',  ( -35.02454729103298803, -113.1123104723225197, 5.402725545821551734 ) ) ;
#18651=VERTEX_POINT ( 'NONE', #8648 ) ;
#18660=CARTESIAN_POINT ( 'NONE',  ( -36.94073759706868287, -112.0000000000000142, 5.628524454178449155 ) ) ;
#18661=CARTESIAN_POINT ( 'NONE',  ( -34.50000000000000000, -115.9927366631908825, 10.47601115720670073 ) ) ;
#18669=CARTESIAN_POINT ( 'NONE',  ( -39.07941549657749647, -116.1632251905417803, 9.058975545821549957 ) ) ;
#18692=CARTESIAN_POINT ( 'NONE',  ( -35.50000000000000711, -112.1222502514821144, 1.343475657184566296 ) ) ;
#18698=CARTESIAN_POINT ( 'NONE',  ( -34.50000000000000000, -112.7549084230351752, -1.592823285203595285 ) ) ;
#18699=CARTESIAN_POINT ( 'NONE',  ( -34.50000000000000000, -114.9860996047076895, 10.38555023491505835 ) ) ;
#18701=CARTESIAN_POINT ( 'NONE',  ( -36.12500000000014211, -114.9929510916434339, 13.11852480586264669 ) ) ;
#18703=CARTESIAN_POINT ( 'NONE',  ( -39.00000000000000000, -113.9929510916434339, 12.57451923796417681 ) ) ;
#18707=FILL_AREA_STYLE_COLOUR ( '', #15905 ) ;
#18713=CARTESIAN_POINT ( 'NONE',  ( -37.99994980024369085, -114.9929510916434339, 12.62670525340494621 ) ) ;
#18715=CARTESIAN_POINT ( 'NONE',  ( -37.76916472181487450, -111.9754527089670404, 7.034774454178450931 ) ) ;
#18725=CARTESIAN_POINT ( 'NONE',  ( -39.16322519054179452, -116.0794154965774823, 3.566024454178448710 ) ) ;
#18737=CARTESIAN_POINT ( 'NONE',  ( -34.50000000000000000, -112.6572589393539516, 2.844055607295835397 ) ) ;
#18741=CARTESIAN_POINT ( 'NONE',  ( -35.50000000000000711, -114.2598117360253696, 9.542047897280109936 ) ) ;
#18744=CARTESIAN_POINT ( 'NONE',  ( -34.50000000000000000, -113.9929510916434339, 10.55026311463432087 ) ) ;
#18747=CARTESIAN_POINT ( 'NONE',  ( -38.00000000000000711, -113.9929510916434339, 12.59102132592609102 ) ) ;
#18750=CARTESIAN_POINT ( 'NONE',  ( -36.50000000000010658, -115.9929510916434481, 13.11852480586264846 ) ) ;
#18764=CARTESIAN_POINT ( 'NONE',  ( -35.50000000000000711, -116.0012805033554883, -0.7876962586524312027 ) ) ;
#18768=CARTESIAN_POINT ( 'NONE',  ( -35.50000000000000711, -114.9929517792218689, 10.50900788599415314 ) ) ;
#18773=CARTESIAN_POINT ( 'NONE',  ( -35.50000000000000000, -112.9611193698460738, 2.883091707513499635 ) ) ;
#18777=CARTESIAN_POINT ( 'NONE',  ( -38.99999999999999289, -113.9407375970686900, 2.253524454178449155 ) ) ;
#18784=CARTESIAN_POINT ( 'NONE',  ( -34.50000000000000000, -113.0140978167138712, 0.0002176474015659786963 ) ) ;
#18791=CARTESIAN_POINT ( 'NONE',  ( -38.00000000000000711, -114.9929510916434339, 10.50625754673587231 ) ) ;
#18794=CARTESIAN_POINT ( 'NONE',  ( -34.50000000000000000, -112.0140978167138712, -0.4685323525984295134 ) ) ;
#18804=CARTESIAN_POINT ( 'NONE',  ( -35.50000000000000711, -114.1861579685891712, 9.524983039397698192 ) ) ;
#18818=ORIENTED_EDGE ( 'NONE', *, *, #8362, .T. ) ;
#18824=CARTESIAN_POINT ( 'NONE',  ( -35.02454729103298803, -113.1123104723225197, 6.902725545821550845 ) ) ;
#18844=CARTESIAN_POINT ( 'NONE',  ( -37.76916472181487450, -111.9754527089670404, 7.034774454178450043 ) ) ;
#18846=CARTESIAN_POINT ( 'NONE',  ( -37.46874999999995737, -115.9929510916434481, 14.11852480586265024 ) ) ;
#18855=CARTESIAN_POINT ( 'NONE',  ( -34.92058450342249643, -111.8367748094582197, 9.808975545821553510 ) ) ;
#18861=CARTESIAN_POINT ( 'NONE',  ( -34.50000000000000000, -113.0140978167138712, 0.0002176474015659786963 ) ) ;
#18874=CARTESIAN_POINT ( 'NONE',  ( -35.50000000000000711, -112.6919296022648638, -1.573728109100751116 ) ) ;
#18881=CARTESIAN_POINT ( 'NONE',  ( -34.50000000000000000, -114.8474311500471572, -1.624782352598427959 ) ) ;
#18883=CARTESIAN_POINT ( 'NONE',  ( -35.24442919769869320, -114.9929510916434339, 13.92914543265605509 ) ) ;
#18886=CARTESIAN_POINT ( 'NONE',  ( -35.50000000000000000, -113.9929510916434339, 10.50625754673586876 ) ) ;
#18888=CARTESIAN_POINT ( 'NONE',  ( -34.50000000000000000, -114.0371586325023117, 9.504435485030890973 ) ) ;
#18896=CARTESIAN_POINT ( 'NONE',  ( -37.18750000000006395, -114.9929510916434339, 13.11852480586264669 ) ) ;
#18899=CARTESIAN_POINT ( 'NONE',  ( -37.88768952767750164, -115.9754527089670262, 6.472274454178450043 ) ) ;
#18908=CARTESIAN_POINT ( 'NONE',  ( -36.94073759706868287, -112.0000000000000142, 8.628524454178448266 ) ) ;
#18918=CARTESIAN_POINT ( 'NONE',  ( -34.50000000000000000, -111.0780159515033034, -1.143161139953928762 ) ) ;
#18921=CARTESIAN_POINT ( 'NONE',  ( -35.50000000000000711, -114.9928438774171582, 10.49113435197128652 ) ) ;
#18923=CARTESIAN_POINT ( 'NONE',  ( -34.50015059926905536, -113.9929510916434339, 12.64306614848962518 ) ) ;
#18929=CARTESIAN_POINT ( 'NONE',  ( -37.99959864031216483, -113.9929510916434339, 12.63896776382213538 ) ) ;
#18930=CARTESIAN_POINT ( 'NONE',  ( -38.00000000000000711, -115.9929510916434481, 12.59652202191340820 ) ) ;
#18942=CARTESIAN_POINT ( 'NONE',  ( -35.50000000000000711, -116.0140978167138712, -0.3122823525984417259 ) ) ;
#18945=CARTESIAN_POINT ( 'NONE',  ( -35.50000000000000711, -114.9929510916434339, 12.26648026267477221 ) ) ;
#18950=CARTESIAN_POINT ( 'NONE',  ( -35.50000000000000000, -111.1162063037085801, -1.269118781493287607 ) ) ;
#18953=CARTESIAN_POINT ( 'NONE',  ( -36.94073759706866156, -113.0000000000000000, 5.628524454178450043 ) ) ;
#18962=CARTESIAN_POINT ( 'NONE',  ( -34.50000000000000000, -113.0140978167138996, -0.6247823525984302906 ) ) ;
#18968=CARTESIAN_POINT ( 'NONE',  ( -35.50000000000000000, -113.9883062625807071, 10.50570311110699961 ) ) ;
#18973=CARTESIAN_POINT ( 'NONE',  ( -34.50000000000000000, -114.3474311500471430, -1.624782352598427959 ) ) ;
#18974=CARTESIAN_POINT ( 'NONE',  ( -36.15625000000007816, -115.9929510916434481, 14.11852480586265024 ) ) ;
#18980=CARTESIAN_POINT ( 'NONE',  ( -37.97447287825094264, -115.9929510916434481, 12.77960891308616809 ) ) ;
#19000=CARTESIAN_POINT ( 'NONE',  ( -37.76916472181486739, -116.0245472910329880, 7.465225545821551734 ) ) ;
#19022=CARTESIAN_POINT ( 'NONE',  ( -36.03906250000000000, -115.9929510916434481, 14.11852480586265024 ) ) ;
#19030=CARTESIAN_POINT ( 'NONE',  ( -36.33479806579560289, -113.2509883718313262, 3.808975545821551734 ) ) ;
#19055=CARTESIAN_POINT ( 'NONE',  ( -34.50000000000000000, -114.9724313160460696, -1.624792769101446765 ) ) ;
#19056=CARTESIAN_POINT ( 'NONE',  ( -38.99518666717493431, -114.9929510916434339, 12.74107470552714716 ) ) ;
#19058=CARTESIAN_POINT ( 'NONE',  ( -38.00000000000000711, -114.9929510916434339, 12.26648026267477043 ) ) ;
#19060=CARTESIAN_POINT ( 'NONE',  ( -34.50000000000000000, -114.9929510916434339, 12.53051367006571581 ) ) ;
#19070=CARTESIAN_POINT ( 'NONE',  ( -38.97545270896704039, -113.1123104723225197, 5.347274454178449155 ) ) ;
#19080=CARTESIAN_POINT ( 'NONE',  ( -39.16322519054179452, -116.0794154965774823, 6.566024454178448266 ) ) ;
#19091=CARTESIAN_POINT ( 'NONE',  ( -34.50000000000000000, -112.9650106922503170, -2.624765990393421955 ) ) ;
#19095=CARTESIAN_POINT ( 'NONE',  ( -35.50000000000000711, -114.9860996047076895, 10.38555023491505835 ) ) ;
#19096=CARTESIAN_POINT ( 'NONE',  ( -36.87500000000098765, -113.9929510916434339, 14.11852480586265024 ) ) ;
#19102=CARTESIAN_POINT ( 'NONE',  ( -34.50000000000000000, -113.9929510916434339, 10.50763272073269405 ) ) ;
#19103=CARTESIAN_POINT ( 'NONE',  ( -39.00000000000000711, -114.9929510916434339, 12.53051367006571937 ) ) ;
#19104=CARTESIAN_POINT ( 'NONE',  ( -35.50000000000000711, -114.1189822439768449, 9.514224058074130852 ) ) ;
#19115=CARTESIAN_POINT ( 'NONE',  ( -35.50000000000000000, -113.1981689815712997, 0.8971895242272823756 ) ) ;
#19117=CARTESIAN_POINT ( 'NONE',  ( -36.52652403469556930, -113.0245472910329880, 2.722274454178449155 ) ) ;
#19118=CARTESIAN_POINT ( 'NONE',  ( -35.50000000000000711, -114.9929510916434339, 12.53051367006571581 ) ) ;
#19122=CARTESIAN_POINT ( 'NONE',  ( -35.50000000000000000, -111.0780159515033034, -1.143161139953928762 ) ) ;
#19127=CARTESIAN_POINT ( 'NONE',  ( -35.97545270896702618, -113.6450488405582604, 7.409774454178449155 ) ) ;
#19131=CARTESIAN_POINT ( 'NONE',  ( -34.50000000000000000, -113.0140978167138712, -0.6247823525985405357 ) ) ;
#19139=CARTESIAN_POINT ( 'NONE',  ( -35.50000000000000000, -113.9929510916434339, 11.73841344789270202 ) ) ;
#19143=CARTESIAN_POINT ( 'NONE',  ( -34.50000000000000000, -113.6807644833805995, -1.624782352598427959 ) ) ;
#19144=CARTESIAN_POINT ( 'NONE',  ( -38.99699093265172678, -115.9929510916434481, 12.71660600561481402 ) ) ;
#19150=CARTESIAN_POINT ( 'NONE',  ( -38.00000000000000711, -115.9929510916434481, 12.60752341388803721 ) ) ;
#19172=CARTESIAN_POINT ( 'NONE',  ( -35.00000000000000000, -113.9407375970686900, 3.996475545821551290 ) ) ;
#19181=AXIS2_PLACEMENT_3D ( 'NONE', #34470, #14831, #1159 ) ;
#19185=CARTESIAN_POINT ( 'NONE',  ( -35.50000000000000711, -114.9929510916434339, 10.52000928670414126 ) ) ;
#19191=CARTESIAN_POINT ( 'NONE',  ( -38.42182118622945808, -115.9929510916434481, 13.81802396319329773 ) ) ;
#19201=CARTESIAN_POINT ( 'NONE',  ( -38.97545270896704039, -114.8876895276775087, 7.652725545821552622 ) ) ;
#19224=CARTESIAN_POINT ( 'NONE',  ( -34.50000000000000000, -113.0557643173828524, -1.624792769101735868 ) ) ;
#19225=CARTESIAN_POINT ( 'NONE',  ( -37.34375000000001421, -114.9929510916434339, 14.11852480586264846 ) ) ;
#19226=CARTESIAN_POINT ( 'NONE',  ( -38.00000000000000711, -114.9929510916434339, 12.53051367006571937 ) ) ;
#19228=CARTESIAN_POINT ( 'NONE',  ( -35.24442919769869320, -114.9929510916434339, 13.92914543265605509 ) ) ;
#19240=CARTESIAN_POINT ( 'NONE',  ( -34.02454729103298092, -115.3019030900506294, 4.597274454178449155 ) ) ;
#19249=CARTESIAN_POINT ( 'NONE',  ( -39.97545270896702618, -112.6980969099493990, 6.847274454178448266 ) ) ;
#19262=CARTESIAN_POINT ( 'NONE',  ( -34.50000000000000000, -115.2751396785629510, -2.608751991713152307 ) ) ;
#19265=CARTESIAN_POINT ( 'NONE',  ( -35.50000000000000711, -114.9929510916434339, 12.50851088611648088 ) ) ;
#19267=CARTESIAN_POINT ( 'NONE',  ( -35.75562914091914024, -113.9929510916434339, 14.09929883582542409 ) ) ;
#19271=CARTESIAN_POINT ( 'NONE',  ( -34.50000000000000000, -113.9929510916433060, 10.50625754673589540 ) ) ;
#19272=CARTESIAN_POINT ( 'NONE',  ( -39.00000000000000711, -114.9929510916434339, 12.60752341388803721 ) ) ;
#19274=CARTESIAN_POINT ( 'NONE',  ( -35.50000000000000711, -114.9929510916434339, 10.56126450660895699 ) ) ;
#19286=CARTESIAN_POINT ( 'NONE',  ( -35.50000000000000000, -113.0140978167138712, -0.3747823525984258497 ) ) ;
#19288=CARTESIAN_POINT ( 'NONE',  ( -38.02454729103296671, -114.3549511594417396, 3.659774454178448710 ) ) ;
#19293=CARTESIAN_POINT ( 'NONE',  ( -35.50000000000000711, -113.3557509229967764, 1.923098431109107054 ) ) ;
#19296=CARTESIAN_POINT ( 'NONE',  ( -39.02454729103295961, -114.7691647218148745, 5.159774454178448266 ) ) ;
#19301=CARTESIAN_POINT ( 'NONE',  ( -34.50000000000000000, -115.0140978167138712, -0.3747823525984421145 ) ) ;
#19309=CARTESIAN_POINT ( 'NONE',  ( -35.50160444427493189, -113.9929510916434339, 12.65937477241749853 ) ) ;
#19312=CARTESIAN_POINT ( 'NONE',  ( -34.50000000000000000, -111.0140821919592327, -0.5779076015960634694 ) ) ;
#19313=CARTESIAN_POINT ( 'NONE',  ( -35.50000000000000000, -114.1835524127412924, 8.514811007161055656 ) ) ;
#19321=CARTESIAN_POINT ( 'NONE',  ( -35.50000000000000711, -114.0185793162512908, 9.502217742515812304 ) ) ;
#19342=CARTESIAN_POINT ( 'NONE',  ( -35.97545270896705460, -114.3549511594417680, 7.090225545821551734 ) ) ;
#19355=CARTESIAN_POINT ( 'NONE',  ( -35.50000000000000711, -114.1861579685891712, 9.524983039397698192 ) ) ;
#19367=CARTESIAN_POINT ( 'NONE',  ( -36.06250000000000711, -115.9929510916434481, 14.11852480586265024 ) ) ;
#19378=CARTESIAN_POINT ( 'NONE',  ( -36.23083527818512550, -111.9754527089670404, 8.215225545821549957 ) ) ;
#19411=CARTESIAN_POINT ( 'NONE',  ( -34.50000000000000000, -115.1770117227680998, -1.611965039240062181 ) ) ;
#19413=CARTESIAN_POINT ( 'NONE',  ( -36.12500000000014211, -114.9929510916434339, 14.11852480586264846 ) ) ;
#19415=CARTESIAN_POINT ( 'NONE',  ( -35.50000000000000000, -113.9929510916434339, 10.50625754673587409 ) ) ;
#19418=CARTESIAN_POINT ( 'NONE',  ( -34.50300906734827322, -114.9929510916434339, 12.71660600561482468 ) ) ;
#19429=CARTESIAN_POINT ( 'NONE',  ( -34.00000000000000000, -114.0592624029313242, 6.003524454178450043 ) ) ;
#19431=CARTESIAN_POINT ( 'NONE',  ( -35.50000000000000711, -114.8057644833805568, -1.624782352598427959 ) ) ;
#19450=CARTESIAN_POINT ( 'NONE',  ( -35.50000000000000000, -113.1451905347060460, 2.905063584339864668 ) ) ;
#19454=CARTESIAN_POINT ( 'NONE',  ( -35.50000102263782509, -114.9929510916434339, 12.62466071271731316 ) ) ;
#19455=CARTESIAN_POINT ( 'NONE',  ( -36.12500000000014211, -113.9929510916434339, 14.11852480586265024 ) ) ;
#19461=CARTESIAN_POINT ( 'NONE',  ( -34.50000000000000000, -113.9929510916434339, 11.73841344789270202 ) ) ;
#19462=CARTESIAN_POINT ( 'NONE',  ( -39.00000000000000711, -114.9929510916434339, 12.17846912687782179 ) ) ;
#19464=CARTESIAN_POINT ( 'NONE',  ( -35.50000000000000711, -114.9928438774171582, 10.49113435197128652 ) ) ;
#19474=CARTESIAN_POINT ( 'NONE',  ( -35.50000000000000711, -116.0140978167138712, 0.0002176474015577116276 ) ) ;
#19476=CARTESIAN_POINT ( 'NONE',  ( -38.37230871539094323, -112.5438815906447729, 3.941024454178448710 ) ) ;
#19480=CARTESIAN_POINT ( 'NONE',  ( -35.50000000000000000, -117.0108842342086888, -0.7556348869410856040 ) ) ;
#19483=CARTESIAN_POINT ( 'NONE',  ( -34.97545270896703329, -113.2308352781851539, 8.909774454178450043 ) ) ;
#19488=CARTESIAN_POINT ( 'NONE',  ( -34.50000000000000000, -114.0000000000000853, 2.000000000000001776 ) ) ;
#19492=CARTESIAN_POINT ( 'NONE',  ( -35.50000000000000000, -113.9929510916432207, 10.50625754673563250 ) ) ;
#19495=CARTESIAN_POINT ( 'NONE',  ( -34.50000000000000000, -116.0124910254613297, -0.6902086197697608894 ) ) ;
#19496=CARTESIAN_POINT ( 'NONE',  ( -37.98325232167028531, -115.9929510916434481, 14.04194344061727584 ) ) ;
#19509=CARTESIAN_POINT ( 'NONE',  ( -35.00000000000000000, -114.0000000000003411, 9.500000000000035527 ) ) ;
#19517=CARTESIAN_POINT ( 'NONE',  ( -36.52652403469559061, -114.9754527089670262, 4.277725545821552622 ) ) ;
#19520=ORIENTED_EDGE ( 'NONE', *, *, #23938, .T. ) ;
#19523=CARTESIAN_POINT ( 'NONE',  ( -35.50000000000000711, -113.1807644833805426, -1.624782352598427959 ) ) ;
#19525=CARTESIAN_POINT ( 'NONE',  ( -35.50000000000000711, -114.9656200615856818, 10.26631071845107179 ) ) ;
#19531=CARTESIAN_POINT ( 'NONE',  ( -34.50000000000000000, -114.1152303497977414, 9.513755561829650986 ) ) ;
#19534=CARTESIAN_POINT ( 'NONE',  ( -35.95093014754292682, -115.9929510916434481, 14.11777216781842625 ) ) ;
#19543=CARTESIAN_POINT ( 'NONE',  ( -38.45611840935523418, -112.6276912846090568, 6.433975545821550845 ) ) ;
#19571=CARTESIAN_POINT ( 'NONE',  ( -36.15625000000007816, -114.9929510916434339, 14.11852480586264846 ) ) ;
#19575=CARTESIAN_POINT ( 'NONE',  ( -36.50000000000011369, -114.9929510916434339, 14.11852480586264846 ) ) ;
#19586=CARTESIAN_POINT ( 'NONE',  ( -38.18337828418795965, -110.9754527089670546, 5.534774454178449155 ) ) ;
#19589=CARTESIAN_POINT ( 'NONE',  ( -35.50000000000000711, -115.0468226098135744, -1.624774171496087716 ) ) ;
#19609=CARTESIAN_POINT ( 'NONE',  ( -35.50000000000000000, -111.6790780953339066, 2.383953864837686343 ) ) ;
#19612=CARTESIAN_POINT ( 'NONE',  ( -35.50000000000000711, -114.9929510916434339, 12.44250253426871033 ) ) ;
#19614=CARTESIAN_POINT ( 'NONE',  ( -35.97545865737298953, -113.9929510916434339, 14.11837420659365527 ) ) ;
#19617=CARTESIAN_POINT ( 'NONE',  ( -34.49999793727135966, -113.9929510916434339, 12.61164896875036767 ) ) ;
#19619=CARTESIAN_POINT ( 'NONE',  ( -35.50000000000000711, -114.9929510916434339, 11.73841344789270202 ) ) ;
#19632=CARTESIAN_POINT ( 'NONE',  ( -35.50000000000000000, -113.6807644833805995, -0.6247823525984269599 ) ) ;
#19634=CARTESIAN_POINT ( 'NONE',  ( -35.00000000000000000, -114.0592624029313242, 6.003524454178450043 ) ) ;
#19640=CARTESIAN_POINT ( 'NONE',  ( -35.50000000000000000, -117.0140978167138854, -0.4685323525984309012 ) ) ;
#19644=CARTESIAN_POINT ( 'NONE',  ( -36.94073759706868287, -112.0000000000000142, 5.628524454178449155 ) ) ;
#19649=CARTESIAN_POINT ( 'NONE',  ( -34.50000000000000000, -115.0140978167138712, 0.8752176474015623819 ) ) ;
#19654=CARTESIAN_POINT ( 'NONE',  ( -35.50040135968784938, -113.9929510916434339, 12.63896776382214071 ) ) ;
#19657=CARTESIAN_POINT ( 'NONE',  ( -34.50000000000000000, -116.0140978167138712, 0.3752176474015736507 ) ) ;
#19658=CARTESIAN_POINT ( 'NONE',  ( -35.50000000000000000, -114.2183886307118428, 8.518969274377507617 ) ) ;
#19682=CARTESIAN_POINT ( 'NONE',  ( -37.47347596530441649, -113.0245472910329880, 3.527725545821551734 ) ) ;
#19689=CARTESIAN_POINT ( 'NONE',  ( -35.50000000000000711, -116.0140978167138712, 0.6252176474015648244 ) ) ;
#19691=CARTESIAN_POINT ( 'NONE',  ( -35.50000000000000711, -114.2305202833893816, 9.534416457224700991 ) ) ;
#19696=CARTESIAN_POINT ( 'NONE',  ( -34.50000000000000000, -114.9929510916434339, 10.51725893871048889 ) ) ;
#19699=CARTESIAN_POINT ( 'NONE',  ( -35.50000000000000000, -115.1342778146718473, 8.846135899190283425 ) ) ;
#19700=CARTESIAN_POINT ( 'NONE',  ( -35.50000000000000711, -112.1859307030124739, 1.448610958621386224 ) ) ;
#19710=CARTESIAN_POINT ( 'NONE',  ( -36.94073759706868287, -115.0000000000000000, 2.871475545821551290 ) ) ;
#19735=CARTESIAN_POINT ( 'NONE',  ( -34.50000000000000000, -115.0140978167138712, 0.8752176474015623819 ) ) ;
#19739=CARTESIAN_POINT ( 'NONE',  ( -34.50000000000000000, -115.9929081983957104, 10.49113315946066294 ) ) ;
#19743=CARTESIAN_POINT ( 'NONE',  ( -37.42187499999997158, -114.9929510916434339, 14.11852480586264846 ) ) ;
#19753=CARTESIAN_POINT ( 'NONE',  ( -34.02454729103298092, -115.3019030900506294, 6.097274454178449155 ) ) ;
#19755=CARTESIAN_POINT ( 'NONE',  ( -35.50000000000000711, -112.0157046079661995, -0.6902086197697556713 ) ) ;
#19761=VERTEX_POINT ( 'NONE', #10393 ) ;
#19773=CARTESIAN_POINT ( 'NONE',  ( -35.50000000000000000, -112.8115600290184801, 2.865251044451027074 ) ) ;
#19776=CARTESIAN_POINT ( 'NONE',  ( -35.50000000000000711, -114.9929510916434339, 12.17846912687782712 ) ) ;
#19778=CARTESIAN_POINT ( 'NONE',  ( -38.99699093265172678, -113.9929510916434339, 12.71660600561481402 ) ) ;
#19781=CARTESIAN_POINT ( 'NONE',  ( -34.50000000000000000, -113.9929510916434339, 10.72628538622835670 ) ) ;
#19783=CARTESIAN_POINT ( 'NONE',  ( -35.50000000000000711, -114.1152303497977414, 9.513755561829650986 ) ) ;
#19799=CARTESIAN_POINT ( 'NONE',  ( -35.50000000000000000, -115.0140978167137860, -0.6247823525984403936 ) ) ;
#19801=CARTESIAN_POINT ( 'NONE',  ( -37.88768952767750164, -115.9754527089670262, 4.972274454178448266 ) ) ;
#19809=CARTESIAN_POINT ( 'NONE',  ( -35.50000000000000711, -112.0209493036498287, 0.9959249592223760050 ) ) ;
#19817=CARTESIAN_POINT ( 'NONE',  ( -34.50000000000000000, -113.0796441757086939, 1.890140615870383956 ) ) ;
#19826=CARTESIAN_POINT ( 'NONE',  ( -35.50000000000000000, -113.9929510916434339, 10.50625754673588474 ) ) ;
#19831=CARTESIAN_POINT ( 'NONE',  ( -34.50000000000000000, -111.0360125565790383, 1.176611260687384419 ) ) ;
#19832=CARTESIAN_POINT ( 'NONE',  ( -38.99924736195577424, -115.9929510916434481, 12.66759465831984599 ) ) ;
#19856=CARTESIAN_POINT ( 'NONE',  ( -37.99999999999998579, -114.0592624029313242, 6.246475545821551734 ) ) ;
#19862=CARTESIAN_POINT ( 'NONE',  ( -35.50000000000000711, -113.6807644833805995, -1.624782352598427959 ) ) ;
#19872=CARTESIAN_POINT ( 'NONE',  ( -34.50000000000000000, -114.1264797827112574, 9.515205387299289441 ) ) ;
#19877=CARTESIAN_POINT ( 'NONE',  ( -35.50000000000000000, -114.2600084737790809, 8.524153227862690585 ) ) ;
#19878=CARTESIAN_POINT ( 'NONE',  ( -35.50000000000000711, -112.0140900043112282, 0.8439677466545482121 ) ) ;
#19888=CARTESIAN_POINT ( 'NONE',  ( -37.05926240293131713, -113.0000000000000000, 6.621475545821551734 ) ) ;
#19898=CARTESIAN_POINT ( 'NONE',  ( -39.07941549657749647, -116.1632251905417803, 4.558975545821549957 ) ) ;
#19914=CARTESIAN_POINT ( 'NONE',  ( -34.50000000000000000, -114.6807644833805000, -0.6247823525984269599 ) ) ;
#19917=CARTESIAN_POINT ( 'NONE',  ( -34.50000000000000000, -115.9929510916434481, 10.52826033068511435 ) ) ;
#19921=CARTESIAN_POINT ( 'NONE',  ( -37.88878409051687868, -114.9929510916434339, 14.07058620477052102 ) ) ;
#19934=CARTESIAN_POINT ( 'NONE',  ( -35.81662171581204746, -117.0245472910329738, 7.784774454178449155 ) ) ;
#19937=CARTESIAN_POINT ( 'NONE',  ( -35.50000000000000711, -115.1446187476384040, -1.616767172155725740 ) ) ;
#19944=AXIS2_PLACEMENT_3D ( 'NONE', #15584, #26782, #20993 ) ;
#19948=CARTESIAN_POINT ( 'NONE',  ( -38.37230871539094323, -115.4561184093552413, 4.558975545821550845 ) ) ;
#19954=CARTESIAN_POINT ( 'NONE',  ( -35.50000000000000000, -111.0140978167138570, 0.6252176474015680441 ) ) ;
#19961=CARTESIAN_POINT ( 'NONE',  ( -35.50000000000000711, -114.9929510916434339, 12.26648026267477221 ) ) ;
#19962=CARTESIAN_POINT ( 'NONE',  ( -39.00000000000000000, -113.9929510916434339, 11.21034663311206181 ) ) ;
#19966=CARTESIAN_POINT ( 'NONE',  ( -36.62499999999902656, -113.9929510916434339, 14.11852480586265024 ) ) ;
#19968=CARTESIAN_POINT ( 'NONE',  ( -35.91854304697313438, -114.9929510916434339, 13.11211614918345703 ) ) ;
#19974=CARTESIAN_POINT ( 'NONE',  ( -37.99839555572501837, -115.9929510916434481, 12.65937477241749143 ) ) ;
#19984=CARTESIAN_POINT ( 'NONE',  ( -35.50000000000000000, -115.0140978167138712, -0.4685323525984309012 ) ) ;
#19986=CARTESIAN_POINT ( 'NONE',  ( -36.25098837183129774, -113.3347980657956242, 8.816024454178446490 ) ) ;
#19988=CARTESIAN_POINT ( 'NONE',  ( -36.23083527818512550, -116.0245472910329880, 3.284774454178449155 ) ) ;
#19991=CARTESIAN_POINT ( 'NONE',  ( -35.50000000000000000, -115.3399256288223569, -2.599147725881697291 ) ) ;
#19994=CARTESIAN_POINT ( 'NONE',  ( -38.37230871539094323, -112.5438815906447729, 6.941024454178449155 ) ) ;
#19999=CARTESIAN_POINT ( 'NONE',  ( -34.50000000000000000, -115.0140978167137860, -0.6247823525984403936 ) ) ;
#20009=CARTESIAN_POINT ( 'NONE',  ( -36.62499999999902656, -113.9929510916434339, 13.11852480586264846 ) ) ;
#20013=CARTESIAN_POINT ( 'NONE',  ( -34.50000000000000000, -116.0140896356112989, -0.6575071456984549201 ) ) ;
#20015=CARTESIAN_POINT ( 'NONE',  ( -35.50000000000000000, -115.9929510916434481, 10.59426868253284226 ) ) ;
#20041=CARTESIAN_POINT ( 'NONE',  ( -35.00000000000000000, -113.9407375970686900, 9.996475545821549957 ) ) ;
#20048=CARTESIAN_POINT ( 'NONE',  ( -35.50000000000000711, -115.1446187476384040, -1.616767172155725740 ) ) ;
#20050=CARTESIAN_POINT ( 'NONE',  ( -35.50100302244946704, -114.9929510916434339, 12.65121853911337269 ) ) ;
#20055=CARTESIAN_POINT ( 'NONE',  ( -34.50000000000000000, -114.9929510916434339, 10.59426868253284226 ) ) ;
#20062=CARTESIAN_POINT ( 'NONE',  ( -35.50000000000000000, -115.3279708130221479, 8.997521329298534098 ) ) ;
#20063=CARTESIAN_POINT ( 'NONE',  ( -35.50000000000000711, -113.3557509229967764, 1.923098431109107054 ) ) ;
#20070=CARTESIAN_POINT ( 'NONE',  ( -37.74901162816868805, -113.3347980657955958, 6.433975545821551734 ) ) ;
#20081=CARTESIAN_POINT ( 'NONE',  ( -38.30190309005061522, -116.9754527089670546, 6.472274454178449155 ) ) ;
#20097=ORIENTED_EDGE ( 'NONE', *, *, #2381, .T. ) ;
#20099=CARTESIAN_POINT ( 'NONE',  ( -34.50000000000000000, -113.2637153405686519, 1.912112492696748989 ) ) ;
#20102=CARTESIAN_POINT ( 'NONE',  ( -34.50000000000000000, -114.5266723804073195, 8.577838247824468354 ) ) ;
#20105=CARTESIAN_POINT ( 'NONE',  ( -34.50000000000000000, -114.3793648455349654, 8.543708532059524074 ) ) ;
#20115=CARTESIAN_POINT ( 'NONE',  ( -40.02454729103296671, -112.8166217158120332, 7.840225545821554398 ) ) ;
#20117=CARTESIAN_POINT ( 'NONE',  ( -35.50000000000000711, -115.0795240838853886, -1.623175561345890472 ) ) ;
#20130=CARTESIAN_POINT ( 'NONE',  ( -38.37230871539094323, -115.4561184093552413, 7.558975545821551734 ) ) ;
#20136=CARTESIAN_POINT ( 'NONE',  ( -35.50000000000000000, -113.4307644833805142, -2.624782352598442614 ) ) ;
#20142=CARTESIAN_POINT ( 'NONE',  ( -37.46874999999995737, -113.9929510916434339, 14.11852480586265024 ) ) ;
#20145=CARTESIAN_POINT ( 'NONE',  ( -35.07817881376918479, -113.9929510916434339, 13.81802396319203474 ) ) ;
#20147=CARTESIAN_POINT ( 'NONE',  ( -36.12500000000014211, -114.9929510916434339, 13.11852480586264669 ) ) ;
#20153=CARTESIAN_POINT ( 'NONE',  ( -35.91854304697313438, -114.9929510916434339, 13.11211614918345703 ) ) ;
#20154=( BOUNDED_SURFACE ( )  B_SPLINE_SURFACE ( 3, 3, ( 
 ( #12459, #23073, #29020, #20352, #6694, #33889, #17676, #28844, #34247, #28675, #7046, #4021, #31550, #23253, #14965, #9580, #20549, #22896, #31184, #4195, #26330, #34439, #6513, #15137, #26144, #4369, #23445, #18023, #9757, #20718, #31715, #15317, #9220, #28424, #6102, #33829, #3423, #3067, #5927, #25204, #33465, #17071, #30767, #3766, #19755, #25379, #28080, #8789, #30945, #526, #14202, #17246, #14373, #3239, #27893, #867, #14023, #691, #5759, #33298, #11675, #16716, #11506, #14723, #22642, #25016, #28252, #22305, #6453, #8619, #16889, #19431, #22476, #33636, #8970, #19589, #20117, #19937, #6278, #3591, #14539, #30592, #341, #8450, #30429, #11339, #17423, #25554, #27727, #11852, #22833, #31126, #9153, #25737, #1067, #12036, #23011, #34188, #34546, #18325, #31651, #23733 ),
 ( #25913, #4673, #6626, #9693, #1240, #15602, #7163, #29146, #6985, #12578, #29323, #6808, #32014, #1600, #9863, #10044, #34371, #20649, #31486, #31828, #21009, #7354, #17779, #12933, #23370, #9335, #3959, #9511, #26624, #20294, #34724, #1957, #14902, #34011, #17957, #26261, #31300, #17598, #28608, #1778, #12217, #23194, #20472, #28783, #4133, #28960, #18137, #23550, #20825, #15430, #4306, #15072, #12755, #26084, #1415, #12392, #4498, #26443, #15250, #6737, #12500, #31585, #34291, #26554, #23482, #7089, #1340, #26184, #18062, #17527, #34477, #12142, #28886, #9434, #1519, #34830, #4236, #9796, #29254, #12319, #6916, #3879, #17888, #20757, #34113, #12865, #14839, #15176, #20392, #23841, #15356, #1702, #31757, #29064, #1892, #15006, #4599, #4414, #26370, #18249, #12687, #23664 ),
 ( #31404, #17715, #34653, #23291, #23116, #28714, #9973, #20933, #31933, #7271, #4063, #15533, #10153, #26011, #21123, #9621, #6551, #28531, #25844, #1168, #20588, #21299, #35362, #29425, #30131, #18608, #13045, #10691, #2424, #5127, #13393, #24734, #13226, #32656, #27442, #18784, #24031, #24375, #32295, #21655, #21472, #24200, #16421, #7981, #18962, #26914, #16064, #29958, #7450, #5299, #2070, #29786, #35022, #27083, #59, #16240, #27259, #19131, #2258, #4773, #7617, #7798, #15716, #35192, #2789, #32468, #10340, #2599, #29606, #5467, #4945, #15894, #18426, #10510, #13567, #24557, #35549, #8149, #10876, #21838, #32831, #13752, #11046, #32122, #26730, #8322, #2958, #19999, #17131, #33008, #16779, #33529, #9041, #8857, #22709, #19301, #24904, #33186, #22184, #22536, #6340, #19649 ),
 ( #19488, #11212, #228, #30492, #28138, #3306, #19817, #582, #16947, #27953, #942, #14431, #5650, #3481, #405, #25618, #25439, #3127, #27791, #22011, #14079, #27623, #757, #5821, #25075, #8513, #5991, #11399, #22360, #33356, #30313, #30829, #31006, #16611, #8681, #14605, #11737, #14260, #6166, #13916, #30659, #33703, #3657, #25260, #17307, #11568, #28310, #1474, #23624, #12282, #9219, #1295, #17846, #3836, #18206, #20177, #23252, #14795, #29215, #20717, #7045, #20548, #26143, #7224, #20351, #9928, #15136, #23444, #34612, #34246, #9578, #9395, #9756, #20891, #31890, #31362, #26514, #31549, #22895, #17488, #12098, #4562, #33888, #1663, #15495, #28485, #12644, #6874, #4194, #31183, #11923, #6512, #15315, #25801, #1127, #23072, #34069, #6692, #28843, #31714, #12457, #34438 ),
 ( #17675, #28674, #18022, #4020, #29019, #14964, #4368, #25969, #26329, #26867, #29569, #21790, #18737, #2388, #32260, #21434, #13356, #12821, #7755, #23982, #18386, #16024, #29740, #10474, #5084, #30090, #18565, #24337, #32786, #24159, #29390, #27044, #2024, #35328, #2217, #4904, #8109, #10649, #21605, #7581, #32432, #32608, #23802, #7939, #7412, #35154, #4735, #18918, #5430, #29916, #5261, #24510, #15845, #34785, #26692, #13185, #10105, #16199, #19091, #27220, #15671, #2563, #12996, #35502, #34978, #10300, #21075, #13529, #10835, #16378, #21261, #1848, #32082, #30614, #11356, #5779, #2915, #19262, #27393, #13710, #8284, #25397, #22496, #2746, #22146, #3258, #14389, #14220, #28097, #24688, #30266, #13875, #27577, #27911, #11692, #25037, #17087, #22323, #21967, #24861, #8469, #16737 ),
 ( #8639, #14038, #27745, #25222, #19450, #33140, #541, #3085, #30448, #11174, #19773, #32965, #33315, #16, #710, #358, #16570, #186, #19609, #5946, #5607, #16906, #11525, #33485, #8810, #30785, #6119, #3440, #22665, #33655, #8988, #19954, #30964, #6297, #11002, #17265, #14745, #6471, #20494, #14557, #15270, #3976, #9880, #20670, #9531, #17797, #11873, #31144, #31666, #34565, #17441, #26279, #23210, #25754, #6829, #28976, #17620, #25575, #6647, #34203, #9171, #23571, #893, #28629, #20136, #20842, #26101, #12410, #25927, #31504, #12597, #1083, #1618, #28799, #4149, #4325, #14918, #1253, #12052, #15089, #31845, #28270, #23027, #3611, #12237, #22850, #33846, #28444, #3788, #34029, #7001, #9353, #20309, #17974, #1432, #23393, #31319, #34391, #9711, #10601, #276, #10061 ),
 ( #5218, #29342, #23750, #21391, #13142, #15798, #24120, #11260, #23937, #7706, #2515, #29521, #34740, #35109, #7371, #10432, #32211, #34931, #27175, #32385, #18692, #1974, #26819, #29689, #18158, #5033, #12774, #4856, #21029, #2170, #22233, #15983, #26999, #29872, #12950, #4517, #32034, #18518, #15448, #10256, #13481, #7539, #18343, #2344, #4688, #16156, #15621, #26645, #29166, #21219, #13314, #24293, #35282, #18874, #21558, #32557, #7889, #24463, #7180, #26462, #1797, #19523, #14128, #33756, #28533, #19862, #25128, #3524, #33398, #14472, #22578, #25302, #17529, #25482, #9089, #28006, #17175, #20048, #8551, #801, #3171, #30878, #458, #28182, #25845, #6216, #11780, #20222, #3357, #30531, #22402, #8901, #5861, #14303, #3881, #33571, #11438, #17349, #8722, #31229, #19689, #6034 ) ),
 .UNSPECIFIED., .T., .F., .F. ) 
 B_SPLINE_SURFACE_WITH_KNOTS ( ( 4, 3, 4 ),
 ( 4, 2, 2, 2, 2, 2, 2, 2, 2, 2, 2, 2, 2, 2, 2, 2, 2, 2, 2, 2, 2, 2, 2, 2, 2, 2, 2, 2, 2, 2, 2, 2, 2, 2, 2, 2, 2, 2, 2, 2, 2, 2, 2, 2, 2, 2, 2, 2, 2, 2, 4 ),
 ( 0.000000000000000000, 0.5000000000000000000, 1.000000000000000000 ),
 ( 0.000000000000000000, 0.05194669433742771930, 0.07792004150614158242, 0.09090671509049851051, 0.09740005188267697456, 0.1038933886748554386, 0.1123700156520060500, 0.1208466426291566476, 0.1377998965834578704, 0.1717064044920602883, 0.2056129124006627062, 0.2225661663549639291, 0.2310427933321145266, 0.2395194203092651519, 0.2482763131408625423, 0.2570332059724599327, 0.2745469916356546580, 0.3095745629620442196, 0.3446021342884337813, 0.3621159199516285621, 0.3708728127832259247, 0.3796297056148233429, 0.3887999023441631730, 0.3979700990735030031, 0.4163104925321826633, 0.4529912794495420392, 0.4896720663669014151, 0.5080124598255810753, 0.5171826565549209054, 0.5263528532842607355, 0.5380287103930572190, 0.5497045675018538136, 0.5730562817194468916, 0.6197597101546329368, 0.6664631385898189819, 0.6898148528074120600, 0.7014907099162086546, 0.7131665670250051381, 0.7223367637543449682, 0.7315069604836847983, 0.7498473539423643475, 0.7865281408597235568, 0.8232089277770826552, 0.8415493212357623154, 0.8507195179651021455, 0.8598897146944418646, 0.8686466075260392827, 0.8774035003576365899, 0.8949172860208314262, 0.9299448573472208768, 1.000000000000000000 ),
 .UNSPECIFIED. ) 
 GEOMETRIC_REPRESENTATION_ITEM ( )  RATIONAL_B_SPLINE_SURFACE ( (
 ( 1.000000000000000000, 1.000000000000000000, 1.000000000000000000, 1.000000000000000000, 1.000000000000000000, 1.000000000000000000, 1.000000000000000000, 1.000000000000000000, 1.000000000000000000, 1.000000000000000000, 1.000000000000000000, 1.000000000000000000, 1.000000000000000000, 1.000000000000000000, 1.000000000000000000, 1.000000000000000000, 1.000000000000000000, 1.000000000000000000, 1.000000000000000000, 1.000000000000000000, 1.000000000000000000, 1.000000000000000000, 1.000000000000000000, 1.000000000000000000, 1.000000000000000000, 1.000000000000000000, 1.000000000000000000, 1.000000000000000000, 1.000000000000000000, 1.000000000000000000, 1.000000000000000000, 1.000000000000000000, 1.000000000000000000, 1.000000000000000000, 1.000000000000000000, 1.000000000000000000, 1.000000000000000000, 1.000000000000000000, 1.000000000000000000, 1.000000000000000000, 1.000000000000000000, 1.000000000000000000, 1.000000000000000000, 1.000000000000000000, 1.000000000000000000, 1.000000000000000000, 1.000000000000000000, 1.000000000000000000, 1.000000000000000000, 1.000000000000000000, 1.000000000000000000, 1.000000000000000000, 1.000000000000000000, 1.000000000000000000, 1.000000000000000000, 1.000000000000000000, 1.000000000000000000, 1.000000000000000000, 1.000000000000000000, 1.000000000000000000, 1.000000000000000000, 1.000000000000000000, 1.000000000000000000, 1.000000000000000000, 1.000000000000000000, 1.000000000000000000, 1.000000000000000000, 1.000000000000000000, 1.000000000000000000, 1.000000000000000000, 1.000000000000000000, 1.000000000000000000, 1.000000000000000000, 1.000000000000000000, 1.000000000000000000, 1.000000000000000000, 1.000000000000000000, 1.000000000000000000, 1.000000000000000000, 1.000000000000000000, 1.000000000000000000, 1.000000000000000000, 1.000000000000000000, 1.000000000000000000, 1.000000000000000000, 1.000000000000000000, 1.000000000000000000, 1.000000000000000000, 1.000000000000000000, 1.000000000000000000, 1.000000000000000000, 1.000000000000000000, 1.000000000000000000, 1.000000000000000000, 1.000000000000000000, 1.000000000000000000, 1.000000000000000000, 1.000000000000000000, 1.000000000000000000, 1.000000000000000000, 1.000000000000000000, 1.000000000000000000),
 ( 0.3333333333333333703, 0.3333333333333333703, 0.3333333333333333703, 0.3333333333333333703, 0.3333333333333333703, 0.3333333333333333703, 0.3333333333333333703, 0.3333333333333333703, 0.3333333333333333703, 0.3333333333333333703, 0.3333333333333333703, 0.3333333333333333703, 0.3333333333333333703, 0.3333333333333333703, 0.3333333333333333703, 0.3333333333333333703, 0.3333333333333333703, 0.3333333333333333703, 0.3333333333333333703, 0.3333333333333333703, 0.3333333333333333703, 0.3333333333333333703, 0.3333333333333333703, 0.3333333333333333703, 0.3333333333333333703, 0.3333333333333333703, 0.3333333333333333703, 0.3333333333333333703, 0.3333333333333333703, 0.3333333333333333703, 0.3333333333333333703, 0.3333333333333333703, 0.3333333333333333703, 0.3333333333333333703, 0.3333333333333333703, 0.3333333333333333703, 0.3333333333333333703, 0.3333333333333333703, 0.3333333333333333703, 0.3333333333333333703, 0.3333333333333333703, 0.3333333333333333703, 0.3333333333333333703, 0.3333333333333333703, 0.3333333333333333703, 0.3333333333333333703, 0.3333333333333333703, 0.3333333333333333703, 0.3333333333333333703, 0.3333333333333333703, 0.3333333333333333703, 0.3333333333333333703, 0.3333333333333333703, 0.3333333333333333703, 0.3333333333333333703, 0.3333333333333333703, 0.3333333333333333703, 0.3333333333333333703, 0.3333333333333333703, 0.3333333333333333703, 0.3333333333333333703, 0.3333333333333333703, 0.3333333333333333703, 0.3333333333333333703, 0.3333333333333333703, 0.3333333333333333703, 0.3333333333333333703, 0.3333333333333333703, 0.3333333333333333703, 0.3333333333333333703, 0.3333333333333333703, 0.3333333333333333703, 0.3333333333333333703, 0.3333333333333333703, 0.3333333333333333703, 0.3333333333333333703, 0.3333333333333333703, 0.3333333333333333703, 0.3333333333333333703, 0.3333333333333333703, 0.3333333333333333703, 0.3333333333333333703, 0.3333333333333333703, 0.3333333333333333703, 0.3333333333333333703, 0.3333333333333333703, 0.3333333333333333703, 0.3333333333333333703, 0.3333333333333333703, 0.3333333333333333703, 0.3333333333333333703, 0.3333333333333333703, 0.3333333333333333703, 0.3333333333333333703, 0.3333333333333333703, 0.3333333333333333703, 0.3333333333333333703, 0.3333333333333333703, 0.3333333333333333703, 0.3333333333333333703, 0.3333333333333333703, 0.3333333333333333703),
 ( 0.3333333333333333703, 0.3333333333333333703, 0.3333333333333333703, 0.3333333333333333703, 0.3333333333333333703, 0.3333333333333333703, 0.3333333333333333703, 0.3333333333333333703, 0.3333333333333333703, 0.3333333333333333703, 0.3333333333333333703, 0.3333333333333333703, 0.3333333333333333703, 0.3333333333333333703, 0.3333333333333333703, 0.3333333333333333703, 0.3333333333333333703, 0.3333333333333333703, 0.3333333333333333703, 0.3333333333333333703, 0.3333333333333333703, 0.3333333333333333703, 0.3333333333333333703, 0.3333333333333333703, 0.3333333333333333703, 0.3333333333333333703, 0.3333333333333333703, 0.3333333333333333703, 0.3333333333333333703, 0.3333333333333333703, 0.3333333333333333703, 0.3333333333333333703, 0.3333333333333333703, 0.3333333333333333703, 0.3333333333333333703, 0.3333333333333333703, 0.3333333333333333703, 0.3333333333333333703, 0.3333333333333333703, 0.3333333333333333703, 0.3333333333333333703, 0.3333333333333333703, 0.3333333333333333703, 0.3333333333333333703, 0.3333333333333333703, 0.3333333333333333703, 0.3333333333333333703, 0.3333333333333333703, 0.3333333333333333703, 0.3333333333333333703, 0.3333333333333333703, 0.3333333333333333703, 0.3333333333333333703, 0.3333333333333333703, 0.3333333333333333703, 0.3333333333333333703, 0.3333333333333333703, 0.3333333333333333703, 0.3333333333333333703, 0.3333333333333333703, 0.3333333333333333703, 0.3333333333333333703, 0.3333333333333333703, 0.3333333333333333703, 0.3333333333333333703, 0.3333333333333333703, 0.3333333333333333703, 0.3333333333333333703, 0.3333333333333333703, 0.3333333333333333703, 0.3333333333333333703, 0.3333333333333333703, 0.3333333333333333703, 0.3333333333333333703, 0.3333333333333333703, 0.3333333333333333703, 0.3333333333333333703, 0.3333333333333333703, 0.3333333333333333703, 0.3333333333333333703, 0.3333333333333333703, 0.3333333333333333703, 0.3333333333333333703, 0.3333333333333333703, 0.3333333333333333703, 0.3333333333333333703, 0.3333333333333333703, 0.3333333333333333703, 0.3333333333333333703, 0.3333333333333333703, 0.3333333333333333703, 0.3333333333333333703, 0.3333333333333333703, 0.3333333333333333703, 0.3333333333333333703, 0.3333333333333333703, 0.3333333333333333703, 0.3333333333333333703, 0.3333333333333333703, 0.3333333333333333703, 0.3333333333333333703, 0.3333333333333333703),
 ( 1.000000000000000000, 1.000000000000000000, 1.000000000000000000, 1.000000000000000000, 1.000000000000000000, 1.000000000000000000, 1.000000000000000000, 1.000000000000000000, 1.000000000000000000, 1.000000000000000000, 1.000000000000000000, 1.000000000000000000, 1.000000000000000000, 1.000000000000000000, 1.000000000000000000, 1.000000000000000000, 1.000000000000000000, 1.000000000000000000, 1.000000000000000000, 1.000000000000000000, 1.000000000000000000, 1.000000000000000000, 1.000000000000000000, 1.000000000000000000, 1.000000000000000000, 1.000000000000000000, 1.000000000000000000, 1.000000000000000000, 1.000000000000000000, 1.000000000000000000, 1.000000000000000000, 1.000000000000000000, 1.000000000000000000, 1.000000000000000000, 1.000000000000000000, 1.000000000000000000, 1.000000000000000000, 1.000000000000000000, 1.000000000000000000, 1.000000000000000000, 1.000000000000000000, 1.000000000000000000, 1.000000000000000000, 1.000000000000000000, 1.000000000000000000, 1.000000000000000000, 1.000000000000000000, 1.000000000000000000, 1.000000000000000000, 1.000000000000000000, 1.000000000000000000, 1.000000000000000000, 1.000000000000000000, 1.000000000000000000, 1.000000000000000000, 1.000000000000000000, 1.000000000000000000, 1.000000000000000000, 1.000000000000000000, 1.000000000000000000, 1.000000000000000000, 1.000000000000000000, 1.000000000000000000, 1.000000000000000000, 1.000000000000000000, 1.000000000000000000, 1.000000000000000000, 1.000000000000000000, 1.000000000000000000, 1.000000000000000000, 1.000000000000000000, 1.000000000000000000, 1.000000000000000000, 1.000000000000000000, 1.000000000000000000, 1.000000000000000000, 1.000000000000000000, 1.000000000000000000, 1.000000000000000000, 1.000000000000000000, 1.000000000000000000, 1.000000000000000000, 1.000000000000000000, 1.000000000000000000, 1.000000000000000000, 1.000000000000000000, 1.000000000000000000, 1.000000000000000000, 1.000000000000000000, 1.000000000000000000, 1.000000000000000000, 1.000000000000000000, 1.000000000000000000, 1.000000000000000000, 1.000000000000000000, 1.000000000000000000, 1.000000000000000000, 1.000000000000000000, 1.000000000000000000, 1.000000000000000000, 1.000000000000000000, 1.000000000000000000),
 ( 0.3333333333333333703, 0.3333333333333333703, 0.3333333333333333703, 0.3333333333333333703, 0.3333333333333333703, 0.3333333333333333703, 0.3333333333333333703, 0.3333333333333333703, 0.3333333333333333703, 0.3333333333333333703, 0.3333333333333333703, 0.3333333333333333703, 0.3333333333333333703, 0.3333333333333333703, 0.3333333333333333703, 0.3333333333333333703, 0.3333333333333333703, 0.3333333333333333703, 0.3333333333333333703, 0.3333333333333333703, 0.3333333333333333703, 0.3333333333333333703, 0.3333333333333333703, 0.3333333333333333703, 0.3333333333333333703, 0.3333333333333333703, 0.3333333333333333703, 0.3333333333333333703, 0.3333333333333333703, 0.3333333333333333703, 0.3333333333333333703, 0.3333333333333333703, 0.3333333333333333703, 0.3333333333333333703, 0.3333333333333333703, 0.3333333333333333703, 0.3333333333333333703, 0.3333333333333333703, 0.3333333333333333703, 0.3333333333333333703, 0.3333333333333333703, 0.3333333333333333703, 0.3333333333333333703, 0.3333333333333333703, 0.3333333333333333703, 0.3333333333333333703, 0.3333333333333333703, 0.3333333333333333703, 0.3333333333333333703, 0.3333333333333333703, 0.3333333333333333703, 0.3333333333333333703, 0.3333333333333333703, 0.3333333333333333703, 0.3333333333333333703, 0.3333333333333333703, 0.3333333333333333703, 0.3333333333333333703, 0.3333333333333333703, 0.3333333333333333703, 0.3333333333333333703, 0.3333333333333333703, 0.3333333333333333703, 0.3333333333333333703, 0.3333333333333333703, 0.3333333333333333703, 0.3333333333333333703, 0.3333333333333333703, 0.3333333333333333703, 0.3333333333333333703, 0.3333333333333333703, 0.3333333333333333703, 0.3333333333333333703, 0.3333333333333333703, 0.3333333333333333703, 0.3333333333333333703, 0.3333333333333333703, 0.3333333333333333703, 0.3333333333333333703, 0.3333333333333333703, 0.3333333333333333703, 0.3333333333333333703, 0.3333333333333333703, 0.3333333333333333703, 0.3333333333333333703, 0.3333333333333333703, 0.3333333333333333703, 0.3333333333333333703, 0.3333333333333333703, 0.3333333333333333703, 0.3333333333333333703, 0.3333333333333333703, 0.3333333333333333703, 0.3333333333333333703, 0.3333333333333333703, 0.3333333333333333703, 0.3333333333333333703, 0.3333333333333333703, 0.3333333333333333703, 0.3333333333333333703, 0.3333333333333333703, 0.3333333333333333703),
 ( 0.3333333333333333703, 0.3333333333333333703, 0.3333333333333333703, 0.3333333333333333703, 0.3333333333333333703, 0.3333333333333333703, 0.3333333333333333703, 0.3333333333333333703, 0.3333333333333333703, 0.3333333333333333703, 0.3333333333333333703, 0.3333333333333333703, 0.3333333333333333703, 0.3333333333333333703, 0.3333333333333333703, 0.3333333333333333703, 0.3333333333333333703, 0.3333333333333333703, 0.3333333333333333703, 0.3333333333333333703, 0.3333333333333333703, 0.3333333333333333703, 0.3333333333333333703, 0.3333333333333333703, 0.3333333333333333703, 0.3333333333333333703, 0.3333333333333333703, 0.3333333333333333703, 0.3333333333333333703, 0.3333333333333333703, 0.3333333333333333703, 0.3333333333333333703, 0.3333333333333333703, 0.3333333333333333703, 0.3333333333333333703, 0.3333333333333333703, 0.3333333333333333703, 0.3333333333333333703, 0.3333333333333333703, 0.3333333333333333703, 0.3333333333333333703, 0.3333333333333333703, 0.3333333333333333703, 0.3333333333333333703, 0.3333333333333333703, 0.3333333333333333703, 0.3333333333333333703, 0.3333333333333333703, 0.3333333333333333703, 0.3333333333333333703, 0.3333333333333333703, 0.3333333333333333703, 0.3333333333333333703, 0.3333333333333333703, 0.3333333333333333703, 0.3333333333333333703, 0.3333333333333333703, 0.3333333333333333703, 0.3333333333333333703, 0.3333333333333333703, 0.3333333333333333703, 0.3333333333333333703, 0.3333333333333333703, 0.3333333333333333703, 0.3333333333333333703, 0.3333333333333333703, 0.3333333333333333703, 0.3333333333333333703, 0.3333333333333333703, 0.3333333333333333703, 0.3333333333333333703, 0.3333333333333333703, 0.3333333333333333703, 0.3333333333333333703, 0.3333333333333333703, 0.3333333333333333703, 0.3333333333333333703, 0.3333333333333333703, 0.3333333333333333703, 0.3333333333333333703, 0.3333333333333333703, 0.3333333333333333703, 0.3333333333333333703, 0.3333333333333333703, 0.3333333333333333703, 0.3333333333333333703, 0.3333333333333333703, 0.3333333333333333703, 0.3333333333333333703, 0.3333333333333333703, 0.3333333333333333703, 0.3333333333333333703, 0.3333333333333333703, 0.3333333333333333703, 0.3333333333333333703, 0.3333333333333333703, 0.3333333333333333703, 0.3333333333333333703, 0.3333333333333333703, 0.3333333333333333703, 0.3333333333333333703, 0.3333333333333333703),
 ( 1.000000000000000000, 1.000000000000000000, 1.000000000000000000, 1.000000000000000000, 1.000000000000000000, 1.000000000000000000, 1.000000000000000000, 1.000000000000000000, 1.000000000000000000, 1.000000000000000000, 1.000000000000000000, 1.000000000000000000, 1.000000000000000000, 1.000000000000000000, 1.000000000000000000, 1.000000000000000000, 1.000000000000000000, 1.000000000000000000, 1.000000000000000000, 1.000000000000000000, 1.000000000000000000, 1.000000000000000000, 1.000000000000000000, 1.000000000000000000, 1.000000000000000000, 1.000000000000000000, 1.000000000000000000, 1.000000000000000000, 1.000000000000000000, 1.000000000000000000, 1.000000000000000000, 1.000000000000000000, 1.000000000000000000, 1.000000000000000000, 1.000000000000000000, 1.000000000000000000, 1.000000000000000000, 1.000000000000000000, 1.000000000000000000, 1.000000000000000000, 1.000000000000000000, 1.000000000000000000, 1.000000000000000000, 1.000000000000000000, 1.000000000000000000, 1.000000000000000000, 1.000000000000000000, 1.000000000000000000, 1.000000000000000000, 1.000000000000000000, 1.000000000000000000, 1.000000000000000000, 1.000000000000000000, 1.000000000000000000, 1.000000000000000000, 1.000000000000000000, 1.000000000000000000, 1.000000000000000000, 1.000000000000000000, 1.000000000000000000, 1.000000000000000000, 1.000000000000000000, 1.000000000000000000, 1.000000000000000000, 1.000000000000000000, 1.000000000000000000, 1.000000000000000000, 1.000000000000000000, 1.000000000000000000, 1.000000000000000000, 1.000000000000000000, 1.000000000000000000, 1.000000000000000000, 1.000000000000000000, 1.000000000000000000, 1.000000000000000000, 1.000000000000000000, 1.000000000000000000, 1.000000000000000000, 1.000000000000000000, 1.000000000000000000, 1.000000000000000000, 1.000000000000000000, 1.000000000000000000, 1.000000000000000000, 1.000000000000000000, 1.000000000000000000, 1.000000000000000000, 1.000000000000000000, 1.000000000000000000, 1.000000000000000000, 1.000000000000000000, 1.000000000000000000, 1.000000000000000000, 1.000000000000000000, 1.000000000000000000, 1.000000000000000000, 1.000000000000000000, 1.000000000000000000, 1.000000000000000000, 1.000000000000000000, 1.000000000000000000) ) ) 
 REPRESENTATION_ITEM ( '' )  SURFACE ( )  );
#20161=CARTESIAN_POINT ( 'NONE',  ( -35.50000000000000000, -115.0140978167143402, -0.6247823525984417259 ) ) ;
#20163=CARTESIAN_POINT ( 'NONE',  ( -35.62769128460905677, -115.4561184093552413, 3.191024454178449155 ) ) ;
#20167=CARTESIAN_POINT ( 'NONE',  ( -36.11231047232249125, -112.0245472910329880, 2.722274454178448266 ) ) ;
#20169=CARTESIAN_POINT ( 'NONE',  ( -35.50000000000000711, -114.9724313160460696, -1.624792769101446765 ) ) ;
#20177=CARTESIAN_POINT ( 'NONE',  ( -34.50000000000000000, -112.8511839106603247, -1.611965039240275122 ) ) ;
#20182=CARTESIAN_POINT ( 'NONE',  ( -36.31249999999994316, -113.9929510916434339, 13.11852480586264846 ) ) ;
#20183=CARTESIAN_POINT ( 'NONE',  ( -34.50000000000000000, -112.0140978167138712, 0.6252176474015680441 ) ) ;
#20186=COLOUR_RGB ( '', 0.08235294, 0.09019608, 0.10196078) ;
#20188=CARTESIAN_POINT ( 'NONE',  ( -35.50100302244945993, -113.9929510916434339, 12.65121853911337446 ) ) ;
#20189=CARTESIAN_POINT ( 'NONE',  ( -35.56312645773537895, -115.9929510916434481, 12.87038173996308998 ) ) ;
#20207=CARTESIAN_POINT ( 'NONE',  ( -34.50000000000000000, -112.4957190293567066, -2.560864217808777266 ) ) ;
#20211=CARTESIAN_POINT ( 'NONE',  ( -37.74901162816869515, -114.6652019342044042, 5.066024454178449155 ) ) ;
#20222=CARTESIAN_POINT ( 'NONE',  ( -35.50000000000000711, -116.0012805033554883, -0.7876962586524312027 ) ) ;
#20224=CARTESIAN_POINT ( 'NONE',  ( -35.87040530316090070, -114.9929510916434339, 13.10254527216545917 ) ) ;
#20228=CARTESIAN_POINT ( 'NONE',  ( -34.50000000000000000, -114.9929510916434339, 10.52000928670414126 ) ) ;
#20233=CARTESIAN_POINT ( 'NONE',  ( -35.50000000000000000, -115.9929510916434481, 10.61627146648203990 ) ) ;
#20235=CARTESIAN_POINT ( 'NONE',  ( -35.50000000000000711, -112.9185811467682754, 1.870920967077121411 ) ) ;
#20247=CARTESIAN_POINT ( 'NONE',  ( -37.35495115944176803, -115.0245472910329880, 8.965225545821551734 ) ) ;
#20256=CARTESIAN_POINT ( 'NONE',  ( -39.16322519054178741, -111.9205845034225177, 9.433975545821549957 ) ) ;
#20274=CARTESIAN_POINT ( 'NONE',  ( -34.50000000000000000, -115.0140978167137860, -0.6247823525984395054 ) ) ;
#20276=CARTESIAN_POINT ( 'NONE',  ( -34.50000000000000000, -116.0140978167138712, -0.3122823525984417259 ) ) ;
#20277=CARTESIAN_POINT ( 'NONE',  ( -34.50000000000000000, -115.9929510916434481, 10.85830208992344303 ) ) ;
#20280=CARTESIAN_POINT ( 'NONE',  ( -39.02454729103295961, -114.7691647218148745, 2.159774454178448710 ) ) ;
#20281=CARTESIAN_POINT ( 'NONE',  ( -37.59808119975203766, -114.9929510916434339, 14.11551573851448893 ) ) ;
#20291=CARTESIAN_POINT ( 'NONE',  ( -34.00000000000000000, -113.9407375970686758, 2.496475545821551290 ) ) ;
#20294=CARTESIAN_POINT ( 'NONE',  ( -35.50000000000000000, -113.0140978167138712, 0.7502176474015694874 ) ) ;
#20304=CARTESIAN_POINT ( 'NONE',  ( -36.11231047232249836, -115.9754527089670262, 2.777725545821551290 ) ) ;
#20309=CARTESIAN_POINT ( 'NONE',  ( -35.50000000000000000, -117.0140978167138854, -0.5622823525984408377 ) ) ;
#20315=CARTESIAN_POINT ( 'NONE',  ( -38.00000000000000711, -114.9929510916434339, 10.50625754673587231 ) ) ;
#20319=CARTESIAN_POINT ( 'NONE',  ( -39.00000000000000000, -113.9929510916434339, 12.17846912687782179 ) ) ;
#20322=CARTESIAN_POINT ( 'NONE',  ( -37.88878409051687157, -113.9929510916434339, 14.07058620477052280 ) ) ;
#20324=CARTESIAN_POINT ( 'NONE',  ( -35.50000000000000711, -114.9929510916434339, 12.53051367006571581 ) ) ;
#20330=CARTESIAN_POINT ( 'NONE',  ( -35.50040135968785648, -114.9929510916434339, 12.63896776382214071 ) ) ;
#20337=CARTESIAN_POINT ( 'NONE',  ( -35.50000000000000000, -113.0140978167138712, -0.5622823525984297355 ) ) ;
#20339=CARTESIAN_POINT ( 'NONE',  ( -35.00000000000000000, -114.0592624029313242, 9.003524454178448266 ) ) ;
#20342=CARTESIAN_POINT ( 'NONE',  ( -38.37230871539094323, -112.5438815906447729, 3.941024454178448710 ) ) ;
#20344=CARTESIAN_POINT ( 'NONE',  ( -35.50000000000000711, -114.8057644833805568, -1.624782352598427959 ) ) ;
#20351=CARTESIAN_POINT ( 'NONE',  ( -34.50000000000000000, -113.4307644833805000, -1.624782352598427959 ) ) ;
#20352=CARTESIAN_POINT ( 'NONE',  ( -35.50000000000000711, -113.3557509229967764, 1.923098431109107054 ) ) ;
#20358=CARTESIAN_POINT ( 'NONE',  ( -37.80727372874345349, -113.9929510916434339, 13.01835785830664705 ) ) ;
#20361=CARTESIAN_POINT ( 'NONE',  ( -35.50005019975638021, -113.9929510916434339, 12.62670525340498351 ) ) ;
#20363=B_SPLINE_CURVE_WITH_KNOTS ( 'NONE', 3,
 ( #13359, #32972, #10838, #2028, #21794, #32437, #18393, #32792, #35158, #13190, #29396, #10477, #23991, #13533, #26874, #24164, #7585, #24341, #7758, #4907, #18741, #4741, #15677, #10303, #16381, #24517, #13001, #21440, #35332, #21266, #19095, #18573, #29573, #15849, #2222, #29746, #18921, #2753, #16030, #8114, #10654, #21609, #32614, #7942, #30095, #29923, #5433, #5265, #24692, #27225, #27399, #16202, #2566, #13713, #20, #6300, #11532, #19776, #19961, #8646, #19612, #19265, #17270, #25040, #33145, #8475, #33319, #3089, #24864, #19454, #30787, #543, #33487, #25224, #193, #5951, #28273, #16741, #28100, #11361, #22500, #11698, #896, #361, #8815, #3262, #22149, #30968, #27748, #6126, #27915, #22325, #30454, #11178, #8287, #30270, #5783, #3616, #3444, #5613, #14043, #11876, #17093, #30616, #25402, #25578, #16908, #14565, #14224, #14394, #715, #22854, #22668, #16575, #33658, #8992, #27581, #2920, #13878, #26284, #3792, #15095, #20501, #23217, #20675, #14921, #3979, #7005, #34207, #28634, #17626, #1624, #28449, #28805, #9176, #7184, #25934, #23033, #34032, #9537, #1257, #9356, #31672, #26107, #23399, #1436, #25759, #31511, #18164, #6652, #17981, #12242, #12414, #4522, #28982, #33850, #31324, #20315 ),
 .UNSPECIFIED., .F., .F.,
 ( 4, 2, 2, 2, 2, 2, 2, 2, 2, 2, 2, 2, 2, 2, 2, 2, 2, 2, 2, 2, 2, 2, 2, 2, 2, 2, 2, 2, 2, 2, 2, 2, 2, 2, 2, 2, 2, 2, 2, 2, 2, 2, 2, 2, 2, 2, 2, 2, 2, 2, 2, 2, 2, 2, 2, 2, 2, 2, 2, 2, 2, 2, 2, 2, 2, 2, 2, 2, 2, 2, 2, 2, 2, 2, 2, 2, 2, 2, 4 ),
 ( 0.000000000000000000, 0.005381740036788157898, 0.008072610055182236413, 0.009418045064379276105, 0.01009076256897779508, 0.01076348007357631580, 0.01185104180586291078, 0.01293860353814950404, 0.01511372700272269054, 0.01946397393186906355, 0.02816446779016181304, 0.04556545550674730855, 0.08036743093991829956, 0.1151694063730892975, 0.1325703940896748034, 0.1412708879479675494, 0.1456211348771139225, 0.1477962583416871090, 0.1488838200739737161, 0.1499713818062602955, 0.1507624401091536004, 0.1515534984120469053, 0.1531356150178334874, 0.1562998482294066793, 0.1626283146525530909, 0.1752852474988458864, 0.2005991131914315051, 0.2512268445766027147, 0.3018545759617738966, 0.3271684416543594875, 0.3398253745006523108, 0.3461538409237986946, 0.3493180741353718588, 0.3509001907411584686, 0.3524823073469450785, 0.3548354025267266287, 0.3571884977065081790, 0.3618946880660712795, 0.3713070687851974805, 0.3901318302234498825, 0.4277813530999547420, 0.4654308759764596015, 0.4842556374147120035, 0.4936680181338382045, 0.4983742084934013050, 0.5007273036731828553, 0.5030803988529644055, 0.5053274392295320494, 0.5075744796060996933, 0.5120685603592350921, 0.5210567218655057786, 0.5390330448780472627, 0.5749856909031301200, 0.6109383369282129772, 0.6289146599407544613, 0.6379028214470251479, 0.6423969022001605467, 0.6446439425767281906, 0.6468909829532958344, 0.6492440781330773847, 0.6515971733128589349, 0.6563033636724220354, 0.6657157443915482364, 0.6845405058298006384, 0.7221900287063054424, 0.7598395515828102464, 0.7786643130210626484, 0.7880766937401888494, 0.7927828840997519499, 0.7951359792795336112, 0.7974890744593151615, 0.7990711910651018268, 0.8006533076708883812, 0.8038175408824614898, 0.8101460073056079292, 0.8228029401519008079, 0.8481168058444863433, 0.8987445372296576362, 1.000000000000000000 ),
 .UNSPECIFIED. ) ;
#20364=CARTESIAN_POINT ( 'NONE',  ( -35.50000000000000000, -115.9929510916434481, 12.57451923796416260 ) ) ;
#20382=CARTESIAN_POINT ( 'NONE',  ( -34.50000000000000000, -114.1807644833817648, -2.624782352598442614 ) ) ;
#20386=CARTESIAN_POINT ( 'NONE',  ( -37.97545270896702618, -114.4734759653044023, 9.152725545821551734 ) ) ;
#20392=CARTESIAN_POINT ( 'NONE',  ( -35.50000000000000000, -115.0140978167137860, -0.6247823525984395054 ) ) ;
#20397=CARTESIAN_POINT ( 'NONE',  ( -35.50000000000000711, -114.9929510916434339, 11.91443571948719971 ) ) ;
#20401=CARTESIAN_POINT ( 'NONE',  ( -36.87500000000098055, -114.9929510916434339, 14.11852480586264846 ) ) ;
#20409=CARTESIAN_POINT ( 'NONE',  ( -35.50000000000000000, -114.8124184834118324, 8.677834500183694288 ) ) ;
#20410=CARTESIAN_POINT ( 'NONE',  ( -35.50000000000000711, -112.0140978167138712, -0.3747823525984256832 ) ) ;
#20420=CARTESIAN_POINT ( 'NONE',  ( -37.35495115944176803, -115.0245472910329880, 5.965225545821550845 ) ) ;
#20428=CARTESIAN_POINT ( 'NONE',  ( -38.30190309005061522, -111.0245472910330022, 8.027725545821551734 ) ) ;
#20451=CARTESIAN_POINT ( 'NONE',  ( -34.50000000000000000, -113.0349311500474982, -0.6247823525985715110 ) ) ;
#20455=CARTESIAN_POINT ( 'NONE',  ( -34.50000000000000000, -115.9920935318519923, 10.44577481630138749 ) ) ;
#20459=CARTESIAN_POINT ( 'NONE',  ( -34.50000000000000000, -114.1556834383649459, 8.511484393387789282 ) ) ;
#20468=CARTESIAN_POINT ( 'NONE',  ( -39.07941549657749647, -116.1632251905417803, 6.058975545821550845 ) ) ;
#20472=CARTESIAN_POINT ( 'NONE',  ( -35.50000000000000000, -113.0140978167139991, -0.6091573525984278481 ) ) ;
#20486=CARTESIAN_POINT ( 'NONE',  ( -35.62769128460905677, -112.5438815906447729, 6.808975545821550845 ) ) ;
#20494=CARTESIAN_POINT ( 'NONE',  ( -35.50000000000000000, -111.0140978167138570, -0.3747823525984258497 ) ) ;
#20497=EDGE_CURVE ( 'NONE', #14462, #18380, #8684, .T. ) ;
#20501=CARTESIAN_POINT ( 'NONE',  ( -37.54084996655477369, -114.9929510916434339, 13.11692036158760466 ) ) ;
#20502=STYLED_ITEM ( 'NONE', ( #32574 ), #22365 ) ;
#20505=CARTESIAN_POINT ( 'NONE',  ( -39.00000000000000000, -113.9929510916434339, 12.59102132592609102 ) ) ;
#20510=CARTESIAN_POINT ( 'NONE',  ( -39.00000000000000000, -113.9929510916434339, 12.60752341388803721 ) ) ;
#20514=CARTESIAN_POINT ( 'NONE',  ( -35.52552712174884419, -114.9929510916434339, 12.77960891308624447 ) ) ;
#20520=CARTESIAN_POINT ( 'NONE',  ( -35.50000000000000711, -114.9929510916434339, 12.59652202191340642 ) ) ;
#20528=CARTESIAN_POINT ( 'NONE',  ( -34.50000000000000000, -112.9990795116828650, 0.8734249692896993711 ) ) ;
#20532=CARTESIAN_POINT ( 'NONE',  ( -35.62769128460905677, -115.4561184093552413, 6.191024454178448266 ) ) ;
#20537=CARTESIAN_POINT ( 'NONE',  ( -35.50000000000000711, -112.0140978167138712, -0.1247823525984259746 ) ) ;
#20544=FILL_AREA_STYLE_COLOUR ( '', #20186 ) ;
#20548=CARTESIAN_POINT ( 'NONE',  ( -34.50000000000000000, -113.1807644833805426, -1.624782352598427959 ) ) ;
#20549=CARTESIAN_POINT ( 'NONE',  ( -35.50000000000000711, -112.6043641208289188, 1.789429170677330649 ) ) ;
#20556=CARTESIAN_POINT ( 'NONE',  ( -36.06250000000000711, -113.9929510916434339, 13.11852480586264846 ) ) ;
#20558=CARTESIAN_POINT ( 'NONE',  ( -36.99999999999988631, -113.9929510916434339, 13.11852480586264846 ) ) ;
#20560=CARTESIAN_POINT ( 'NONE',  ( -35.50000000000000000, -115.9929510916434481, 10.51725893871049067 ) ) ;
#20570=CARTESIAN_POINT ( 'NONE',  ( -35.50000000000000711, -112.0140978167138712, -0.1247823525984259746 ) ) ;
#20578=CARTESIAN_POINT ( 'NONE',  ( -34.50000000000000000, -114.5974311500472567, -2.624782352598442614 ) ) ;
#20582=CARTESIAN_POINT ( 'NONE',  ( -36.02454729103297382, -113.5265240346956261, 9.902725545821553510 ) ) ;
#20588=CARTESIAN_POINT ( 'NONE',  ( -34.50000000000000000, -113.0140978167138712, 0.8752176474013583229 ) ) ;
#20592=CARTESIAN_POINT ( 'NONE',  ( -36.62499999999902656, -114.9929510916434339, 13.11852480586264669 ) ) ;
#20594=CARTESIAN_POINT ( 'NONE',  ( -36.24999999999983658, -114.9929510916434339, 14.11852480586264846 ) ) ;
#20599=CARTESIAN_POINT ( 'NONE',  ( -37.50613590685470911, -115.9929510916434481, 13.11852378322482515 ) ) ;
#20600=CARTESIAN_POINT ( 'NONE',  ( -35.50000000000000711, -114.9724313160460696, -1.624792769101446765 ) ) ;
#20608=CARTESIAN_POINT ( 'NONE',  ( -36.25098837183130485, -114.6652019342044184, 8.683975545821549957 ) ) ;
#20617=CARTESIAN_POINT ( 'NONE',  ( -40.02454729103296671, -112.8166217158120332, 9.340225545821551734 ) ) ;
#20634=CARTESIAN_POINT ( 'NONE',  ( -35.87745010033553683, -115.9929510916434481, 14.11371147303761475 ) ) ;
#20637=CARTESIAN_POINT ( 'NONE',  ( -39.00000000000000711, -114.9929510916434339, 10.85830208992306822 ) ) ;
#20647=CARTESIAN_POINT ( 'NONE',  ( -35.69809690994941320, -116.9754527089670546, 2.777725545821551734 ) ) ;
#20649=CARTESIAN_POINT ( 'NONE',  ( -35.50000000000000000, -113.0140978167142833, 0.8752176474015604946 ) ) ;
#20663=CARTESIAN_POINT ( 'NONE',  ( -37.88768952767750875, -112.0245472910329880, 8.027725545821549957 ) ) ;
#20670=CARTESIAN_POINT ( 'NONE',  ( -35.50000000000000000, -111.0141141789186605, -0.6738694770610589302 ) ) ;
#20675=CARTESIAN_POINT ( 'NONE',  ( -37.58145695302688694, -114.9929510916434339, 13.11211614918362756 ) ) ;
#20677=CARTESIAN_POINT ( 'NONE',  ( -34.50000000000000000, -114.9929510916434339, 12.57451923796416082 ) ) ;
#20679=CARTESIAN_POINT ( 'NONE',  ( -37.51635661748575501, -114.9929510916434339, 13.11827392651459157 ) ) ;
#20682=CARTESIAN_POINT ( 'NONE',  ( -37.74437085908086686, -113.9929510916434339, 14.09929883582536903 ) ) ;
#20686=CARTESIAN_POINT ( 'NONE',  ( -37.50613590685470911, -114.9929510916434339, 13.11852378322482515 ) ) ;
#20691=CARTESIAN_POINT ( 'NONE',  ( -35.50000000000000711, -114.6604609523327838, 9.751889438017201428 ) ) ;
#20698=CARTESIAN_POINT ( 'NONE',  ( -34.50000000000000000, -113.0140978167142833, 0.8752176474019800478 ) ) ;
#20704=CARTESIAN_POINT ( 'NONE',  ( -38.99999999999999289, -113.9407375970686900, 5.253524454178449155 ) ) ;
#20707=CARTESIAN_POINT ( 'NONE',  ( -35.50000000000000711, -112.0140978167138712, 0.5627176474015717078 ) ) ;
#20711=AXIS2_PLACEMENT_3D ( 'NONE', #19509, #21495, #32490 ) ;
#20717=CARTESIAN_POINT ( 'NONE',  ( -34.50000000000000000, -113.0557643173828524, -1.624792769101735868 ) ) ;
#20718=CARTESIAN_POINT ( 'NONE',  ( -35.50000000000000711, -112.0140978167138712, 0.7502176474015694874 ) ) ;
#20725=CARTESIAN_POINT ( 'NONE',  ( -34.50000000000000000, -113.9929510916434623, 10.50436693183592141 ) ) ;
#20728=CARTESIAN_POINT ( 'NONE',  ( -35.96730626674924025, -113.9929510916434339, 13.11752178341330222 ) ) ;
#20730=CARTESIAN_POINT ( 'NONE',  ( -35.51597953369717686, -115.9929510916434481, 12.74811950270164473 ) ) ;
#20743=CARTESIAN_POINT ( 'NONE',  ( -35.50000000000000711, -112.9486715495423681, -1.623175561345890472 ) ) ;
#20750=CARTESIAN_POINT ( 'NONE',  ( -34.50000000000000000, -117.0141134414687514, -0.5779076015960331603 ) ) ;
#20753=ORIENTED_EDGE ( 'NONE', *, *, #4206, .T. ) ;
#20754=CARTESIAN_POINT ( 'NONE',  ( -36.52652403469556930, -113.0245472910329880, 4.222274454178449155 ) ) ;
#20757=CARTESIAN_POINT ( 'NONE',  ( -35.50000000000000000, -115.0140978167134165, -0.6247823525984399495 ) ) ;
#20763=CARTESIAN_POINT ( 'NONE',  ( -35.50005019975638021, -114.9929510916434339, 12.62670525340498529 ) ) ;
#20766=CARTESIAN_POINT ( 'NONE',  ( -34.50000000000000000, -114.9929510916434339, 12.60752341388803544 ) ) ;
#20772=CARTESIAN_POINT ( 'NONE',  ( -35.83891589277641287, -115.9929510916434481, 13.09299768411358400 ) ) ;
#20773=CARTESIAN_POINT ( 'NONE',  ( -35.50000000000000711, -114.5974311500472425, -1.624782352598427959 ) ) ;
#20783=CARTESIAN_POINT ( 'NONE',  ( -37.99999999999998579, -113.9407375970686758, 3.753524454178448710 ) ) ;
#20792=CARTESIAN_POINT ( 'NONE',  ( -35.81662171581203324, -110.9754527089670546, 8.215225545821551734 ) ) ;
#20810=CARTESIAN_POINT ( 'NONE',  ( -35.61121590948313553, -115.9929510916434481, 14.07058620477040733 ) ) ;
#20812=CARTESIAN_POINT ( 'NONE',  ( -38.97545270896704039, -113.1123104723225055, 3.847274454178449599 ) ) ;
#20813=CARTESIAN_POINT ( 'NONE',  ( -34.50000000000000000, -115.9929510916434481, 10.85830208992344303 ) ) ;
#20823=CARTESIAN_POINT ( 'NONE',  ( -35.69809690994941320, -116.9754527089670546, 7.277725545821552622 ) ) ;
#20825=CARTESIAN_POINT ( 'NONE',  ( -35.50000000000000000, -113.0140978167136581, -0.6247823525984261828 ) ) ;
#20842=CARTESIAN_POINT ( 'NONE',  ( -35.50000000000000000, -113.6807644833805995, -2.624782352598442614 ) ) ;
#20851=CARTESIAN_POINT ( 'NONE',  ( -34.50120407906360498, -114.9929510916434339, 12.67985367974112343 ) ) ;
#20855=CARTESIAN_POINT ( 'NONE',  ( -35.74814306589956914, -114.9929510916434339, 13.05539834812772781 ) ) ;
#20857=CARTESIAN_POINT ( 'NONE',  ( -34.50000000000000000, -114.0882517521923489, 9.510534276948430232 ) ) ;
#20859=CARTESIAN_POINT ( 'NONE',  ( -38.00000000000000711, -114.9929510916434339, 12.44250253426874941 ) ) ;
#20865=CARTESIAN_POINT ( 'NONE',  ( -35.50000000000000711, -114.9929510916434339, 10.56126450660895699 ) ) ;
#20868=CARTESIAN_POINT ( 'NONE',  ( -37.05926240293131713, -115.9999999999999858, 1.878524454178448710 ) ) ;
#20875=CARTESIAN_POINT ( 'NONE',  ( -34.50000000000000000, -113.0140978167138712, -0.6247823525988807081 ) ) ;
#20879=CARTESIAN_POINT ( 'NONE',  ( -33.97545270896702618, -112.8166217158120475, 4.409774454178449155 ) ) ;
#20881=CARTESIAN_POINT ( 'NONE',  ( -35.50000000000000711, -114.8474311500471572, -1.624782352598427959 ) ) ;
#20891=CARTESIAN_POINT ( 'NONE',  ( -34.50000000000000000, -114.9307644833806137, -1.624782352598427959 ) ) ;
#20899=CARTESIAN_POINT ( 'NONE',  ( -34.50000000000000000, -113.9929510916434339, 10.50625754673586876 ) ) ;
#20903=CARTESIAN_POINT ( 'NONE',  ( -37.97447287825094264, -113.9929510916434339, 12.77960891308616809 ) ) ;
#20904=CARTESIAN_POINT ( 'NONE',  ( -38.00000068757622529, -115.9929510916434481, 12.61439929482944855 ) ) ;
#20917=CARTESIAN_POINT ( 'NONE',  ( -35.50000000000000711, -112.0141053790792114, 0.9054673897245171243 ) ) ;
#20924=CARTESIAN_POINT ( 'NONE',  ( -34.50000000000000000, -112.3697613878167658, -2.522673865603075605 ) ) ;
#20928=CARTESIAN_POINT ( 'NONE',  ( -37.05926240293131713, -113.0000000000000000, 8.121475545821549957 ) ) ;
#20933=CARTESIAN_POINT ( 'NONE',  ( -34.50000000000000000, -113.1291422947505936, 0.8889500704178361357 ) ) ;
#20942=CARTESIAN_POINT ( 'NONE',  ( -37.75185693410092824, -114.9929510916434339, 13.05539834812634581 ) ) ;
#20946=CARTESIAN_POINT ( 'NONE',  ( -36.50000000000011369, -114.9929510916434339, 14.11852480586264846 ) ) ;
#20950=CARTESIAN_POINT ( 'NONE',  ( -36.15625000000007816, -115.9929510916434481, 13.11852480586264846 ) ) ;
#20963=CARTESIAN_POINT ( 'NONE',  ( -37.66520193420439000, -113.2509883718312977, 2.441024454178448710 ) ) ;
#20971=CARTESIAN_POINT ( 'NONE',  ( -38.99999999999999289, -114.0592624029313242, 3.246475545821551734 ) ) ;
#20993=DIRECTION ( 'NONE',  ( 1.000000000000000000, 0.000000000000000000, -0.000000000000000000 ) ) ;
#20995=CARTESIAN_POINT ( 'NONE',  ( -34.50300906734826611, -115.9929510916434481, 12.71660600561482468 ) ) ;
#20997=CARTESIAN_POINT ( 'NONE',  ( -37.05926240293131713, -115.9999999999999858, 6.378524454178448266 ) ) ;
#20998=CARTESIAN_POINT ( 'NONE',  ( -34.50000000000000000, -115.9929510916434481, 10.94631322572069365 ) ) ;
#21007=CARTESIAN_POINT ( 'NONE',  ( -35.54388159064475872, -115.3723087153909432, 4.183975545821551734 ) ) ;
#21009=CARTESIAN_POINT ( 'NONE',  ( -35.50000000000000000, -113.0140978167138712, 0.8752176474013583229 ) ) ;
#21029=CARTESIAN_POINT ( 'NONE',  ( -35.50000000000000711, -112.0140978167138712, 0.8127176474015721519 ) ) ;
#21035=CARTESIAN_POINT ( 'NONE',  ( -34.51922597003733273, -114.9929510916434339, 12.86289566494349224 ) ) ;
#21038=CARTESIAN_POINT ( 'NONE',  ( -35.60016694755736921, -114.9929510916434339, 12.92579853460621209 ) ) ;
#21040=CARTESIAN_POINT ( 'NONE',  ( -39.00000000000000000, -113.9929510916434339, 12.17846912687782179 ) ) ;
#21045=( NAMED_UNIT ( * ) PLANE_ANGLE_UNIT ( ) SI_UNIT ( $, .RADIAN. ) );
#21051=CARTESIAN_POINT ( 'NONE',  ( -36.87500000000098055, -114.9929510916434339, 13.11852480586264669 ) ) ;
#21053=CARTESIAN_POINT ( 'NONE',  ( -35.54388159064475872, -112.6276912846090568, 5.816024454178449155 ) ) ;
#21059=CARTESIAN_POINT ( 'NONE',  ( -34.50000000000000000, -113.0140978167129617, -0.6247823525984270709 ) ) ;
#21060=CARTESIAN_POINT ( 'NONE',  ( -38.99999999999999289, -113.9407375970686900, 8.253524454178448266 ) ) ;
#21062=CARTESIAN_POINT ( 'NONE',  ( -35.62769128460905677, -115.4561184093552413, 7.691024454178449155 ) ) ;
#21067=CARTESIAN_POINT ( 'NONE',  ( -35.50000000000000711, -116.0140978167138712, 0.6252176474015648244 ) ) ;
#21075=CARTESIAN_POINT ( 'NONE',  ( -34.50000000000000000, -113.8474311500459777, -2.624782352598442614 ) ) ;
#21083=CARTESIAN_POINT ( 'NONE',  ( -34.50000000000000000, -113.9813390189866027, 10.50487145766371100 ) ) ;
#21086=CARTESIAN_POINT ( 'NONE',  ( -38.00000000000000711, -113.9929510916434339, 12.17846912687782179 ) ) ;
#21087=CARTESIAN_POINT ( 'NONE',  ( -36.87500000000098765, -115.9929510916434481, 13.11852480586264846 ) ) ;
#21101=CARTESIAN_POINT ( 'NONE',  ( -35.50000000000000711, -112.4434344552011282, 1.705278471174987986 ) ) ;
#21106=CARTESIAN_POINT ( 'NONE',  ( -35.50000000000000711, -114.3464919575557843, 9.568884482464163455 ) ) ;
#21111=CARTESIAN_POINT ( 'NONE',  ( -35.50000000000000000, -112.7530559548648341, -2.608751991713152307 ) ) ;
#21116=CARTESIAN_POINT ( 'NONE',  ( -36.23083527818512550, -116.0245472910329880, 1.784774454178448932 ) ) ;
#21123=CARTESIAN_POINT ( 'NONE',  ( -34.50000000000000000, -113.0140978167137717, 0.8752176474015607166 ) ) ;
#21132=CARTESIAN_POINT ( 'NONE',  ( -38.00000000000000711, -114.9929510916434339, 11.21034663311206181 ) ) ;
#21135=CARTESIAN_POINT ( 'NONE',  ( -34.50000000000000000, -114.5974311500472425, -1.624782352598427959 ) ) ;
#21136=CARTESIAN_POINT ( 'NONE',  ( -37.69578139638701941, -114.9929510916434339, 14.10650203519847778 ) ) ;
#21140=CARTESIAN_POINT ( 'NONE',  ( -35.56312645773537895, -115.9929510916434481, 12.87038173996308998 ) ) ;
#21153=CARTESIAN_POINT ( 'NONE',  ( -36.94073759706866156, -113.0000000000000000, 5.628524454178450043 ) ) ;
#21167=CARTESIAN_POINT ( 'NONE',  ( -35.02454729103298803, -113.1123104723225197, 3.902725545821551290 ) ) ;
#21187=CARTESIAN_POINT ( 'NONE',  ( -35.02454729103298092, -114.8876895276775087, 7.597274454178450043 ) ) ;
#21188=CARTESIAN_POINT ( 'NONE',  ( -34.50000000000000000, -115.9929510916434481, 10.59426868253284226 ) ) ;
#21199=CARTESIAN_POINT ( 'NONE',  ( -37.76916472181486739, -116.0245472910329880, 4.465225545821550845 ) ) ;
#21219=CARTESIAN_POINT ( 'NONE',  ( -35.50000000000000711, -112.1403507321855528, -1.128496220798856253 ) ) ;
#21225=CARTESIAN_POINT ( 'NONE',  ( -34.50000000000000000, -114.9929510916434339, 12.44250253426871033 ) ) ;
#21228=CARTESIAN_POINT ( 'NONE',  ( -37.46093750000000711, -114.9929510916434339, 13.11852480586264669 ) ) ;
#21230=CARTESIAN_POINT ( 'NONE',  ( -39.00000000000000000, -113.9929510916434339, 11.21034663311206181 ) ) ;
#21233=CARTESIAN_POINT ( 'NONE',  ( -37.99974912065192711, -114.9929510916434339, 12.63488142334838571 ) ) ;
#21234=SURFACE_SIDE_STYLE ('',( #15999 ) ) ;
#21241=CARTESIAN_POINT ( 'NONE',  ( -37.50613590685470911, -114.9929510916434339, 13.11852378322482515 ) ) ;
#21243=CARTESIAN_POINT ( 'NONE',  ( -36.94073759706868287, -112.0000000000000142, 5.628524454178449155 ) ) ;
#21250=CARTESIAN_POINT ( 'NONE',  ( -35.00000000000000000, -114.0592624029313242, 9.003524454178448266 ) ) ;
#21261=CARTESIAN_POINT ( 'NONE',  ( -34.50000000000000000, -114.6807644833805000, -2.624782352598442614 ) ) ;
#21266=CARTESIAN_POINT ( 'NONE',  ( -35.50000000000000711, -114.9819937217110635, 10.35556074009299188 ) ) ;
#21267=CARTESIAN_POINT ( 'NONE',  ( -34.50000000000000000, -113.9929510916435049, 10.50625754673586876 ) ) ;
#21270=CARTESIAN_POINT ( 'NONE',  ( -37.53269373325071712, -113.9929510916434339, 13.11752178341324360 ) ) ;
#21271=CARTESIAN_POINT ( 'NONE',  ( -37.52044295795950291, -115.9929510916434481, 13.11812344617477422 ) ) ;
#21283=CARTESIAN_POINT ( 'NONE',  ( -35.50000000000000711, -112.3465879560236687, 1.629585756119413364 ) ) ;
#21291=CARTESIAN_POINT ( 'NONE',  ( -35.50000000000000000, -112.8115600290184801, 2.865251044451027074 ) ) ;
#21294=CARTESIAN_POINT ( 'NONE',  ( -36.52652403469556930, -113.0245472910329880, 5.722274454178450043 ) ) ;
#21299=CARTESIAN_POINT ( 'NONE',  ( -34.50000000000000000, -113.0140978167138712, 0.8752176474016720720 ) ) ;
#21303=CARTESIAN_POINT ( 'NONE',  ( -38.00000000000000711, -114.9929510916434339, 12.26648026267477043 ) ) ;
#21307=AXIS2_PLACEMENT_3D ( 'NONE', #26589, #12725, #18292 ) ;
#21309=CARTESIAN_POINT ( 'NONE',  ( -34.50000000000000000, -113.0974311500471714, -1.624782352598427959 ) ) ;
#21316=CARTESIAN_POINT ( 'NONE',  ( -35.50025087934803736, -115.9929510916434481, 12.63488142334835196 ) ) ;
#21337=CARTESIAN_POINT ( 'NONE',  ( -38.97545270896704039, -114.8876895276775087, 4.652725545821551734 ) ) ;
#21347=ORIENTED_EDGE ( 'NONE', *, *, #29513, .T. ) ;
#21357=CARTESIAN_POINT ( 'NONE',  ( -35.62769128460905677, -115.4561184093552413, 4.691024454178448266 ) ) ;
#21361=CARTESIAN_POINT ( 'NONE',  ( -34.51922597003733273, -115.9929510916434481, 12.86289566494349224 ) ) ;
#21371=CARTESIAN_POINT ( 'NONE',  ( -38.18337828418796676, -117.0245472910329738, 8.965225545821551734 ) ) ;
#21383=CARTESIAN_POINT ( 'NONE',  ( -37.76916472181486739, -116.0245472910329880, 8.965225545821551734 ) ) ;
#21391=CARTESIAN_POINT ( 'NONE',  ( -35.50000000000000711, -113.3557509229967764, 1.923098431109107054 ) ) ;
#21398=CARTESIAN_POINT ( 'NONE',  ( -34.50000000000000000, -112.0140900043112282, 0.8439677466545482121 ) ) ;
#21399=CARTESIAN_POINT ( 'NONE',  ( -34.50000000000000000, -114.9922651054798308, 10.46846006712531008 ) ) ;
#21402=CARTESIAN_POINT ( 'NONE',  ( -37.99994980024369085, -114.9929510916434339, 12.62670525340494621 ) ) ;
#21405=CARTESIAN_POINT ( 'NONE',  ( -34.50000000000000000, -114.9929510916434339, 10.51725893871048889 ) ) ;
#21414=CARTESIAN_POINT ( 'NONE',  ( -38.00000000000000711, -114.9929510916434339, 12.59102132592608925 ) ) ;
#21417=CARTESIAN_POINT ( 'NONE',  ( -36.23083527818512550, -116.0245472910329880, 6.284774454178450043 ) ) ;
#21423=CARTESIAN_POINT ( 'NONE',  ( -38.45611840935523418, -115.3723087153909432, 8.066024454178448266 ) ) ;
#21434=CARTESIAN_POINT ( 'NONE',  ( -34.50000000000000000, -112.3070160848889429, 2.749963775944984867 ) ) ;
#21440=CARTESIAN_POINT ( 'NONE',  ( -35.50000000000000711, -114.9492820284331742, 10.20776876943783940 ) ) ;
#21441=CARTESIAN_POINT ( 'NONE',  ( -34.50000000000000000, -113.9929510916436470, 10.50625754673586876 ) ) ;
#21444=CARTESIAN_POINT ( 'NONE',  ( -37.99599240977853754, -113.9929510916434339, 12.68378527132499656 ) ) ;
#21445=CARTESIAN_POINT ( 'NONE',  ( -36.00585935943765747, -115.9929510916434481, 13.11852578240983291 ) ) ;
#21458=CARTESIAN_POINT ( 'NONE',  ( -35.50000000000000000, -113.0140978167139991, 0.8752176474014555785 ) ) ;
#21461=CARTESIAN_POINT ( 'NONE',  ( -35.50000000000000711, -114.9929510916434339, 12.56351784598954424 ) ) ;
#21465=CARTESIAN_POINT ( 'NONE',  ( -35.50000000000000000, -112.1946304249441795, 2.703640693953100804 ) ) ;
#21468=CARTESIAN_POINT ( 'NONE',  ( -37.35495115944176092, -112.9754527089670688, 8.534774454178448266 ) ) ;
#21472=CARTESIAN_POINT ( 'NONE',  ( -34.50000000000000000, -113.0140978167138712, -0.4997823525984338988 ) ) ;
#21477=CARTESIAN_POINT ( 'NONE',  ( -38.00000000000000711, -114.9929510916434339, 12.53051367006571937 ) ) ;
#21482=CARTESIAN_POINT ( 'NONE',  ( -34.50000000000000000, -114.8474311500471572, -1.624782352598427959 ) ) ;
#21487=CARTESIAN_POINT ( 'NONE',  ( -37.99974912065192001, -115.9929510916434481, 12.63488142334838749 ) ) ;
#21495=DIRECTION ( 'NONE',  ( 0.000000000000000000, 0.9929510916431029122, -0.1185248058626136303 ) ) ;
#21497=CARTESIAN_POINT ( 'NONE',  ( -34.50000000000000000, -114.0000000000000853, 2.000000000000001776 ) ) ;
#21505=CARTESIAN_POINT ( 'NONE',  ( -38.37230871539094323, -115.4561184093552413, 9.058975545821551734 ) ) ;
#21523=CARTESIAN_POINT ( 'NONE',  ( -39.02454729103295961, -114.7691647218148745, 3.659774454178448710 ) ) ;
#21524=CARTESIAN_POINT ( 'NONE',  ( -37.52454134262689678, -115.9929510916434481, 14.11837420659362152 ) ) ;
#21533=CARTESIAN_POINT ( 'NONE',  ( -34.92058450342249643, -111.8367748094582197, 8.308975545821549957 ) ) ;
#21538=ORIENTED_EDGE ( 'NONE', *, *, #23938, .F. ) ;
#21551=CARTESIAN_POINT ( 'NONE',  ( -38.99999999999999289, -114.0592624029313242, 9.246475545821551734 ) ) ;
#21558=CARTESIAN_POINT ( 'NONE',  ( -35.50000000000000711, -112.7549084230351752, -1.592823285203595285 ) ) ;
#21567=CARTESIAN_POINT ( 'NONE',  ( -34.50000000000000000, -116.0140896356112989, -0.6575071456984549201 ) ) ;
#21568=CARTESIAN_POINT ( 'NONE',  ( -36.03906250000000000, -114.9929510916434339, 14.11852480586264846 ) ) ;
#21570=CARTESIAN_POINT ( 'NONE',  ( -38.00000000000000711, -114.9929510916434339, 11.91443571948719615 ) ) ;
#21572=CARTESIAN_POINT ( 'NONE',  ( -34.50000000000000000, -114.1414532730574507, 9.517316564499758158 ) ) ;
#21581=CARTESIAN_POINT ( 'NONE',  ( -37.46093750000000711, -114.9929510916434339, 13.11852480586264669 ) ) ;
#21583=CARTESIAN_POINT ( 'NONE',  ( -38.99999999999999289, -113.9407375970686900, 8.253524454178448266 ) ) ;
#21594=CARTESIAN_POINT ( 'NONE',  ( -36.94073759706866156, -111.0000000000000284, 5.628524454178450043 ) ) ;
#21605=CARTESIAN_POINT ( 'NONE',  ( -34.50000000000000000, -111.0140978167138570, -0.3747823525984258497 ) ) ;
#21609=CARTESIAN_POINT ( 'NONE',  ( -35.50000000000000711, -114.9929510916434339, 10.51725893871048889 ) ) ;
#21614=CARTESIAN_POINT ( 'NONE',  ( -34.50000000000000000, -113.9929510916434339, 12.26648026267477398 ) ) ;
#21617=CARTESIAN_POINT ( 'NONE',  ( -34.50000000000000000, -113.9948283797722439, 10.50648163149984171 ) ) ;
#21618=CARTESIAN_POINT ( 'NONE',  ( -35.99181955245763476, -115.9929510916434481, 13.11847460610632510 ) ) ;
#21633=CARTESIAN_POINT ( 'NONE',  ( -35.50000000000000000, -113.0140978167137717, 0.8903425666012282358 ) ) ;
#21636=CARTESIAN_POINT ( 'NONE',  ( -35.50000000000000711, -114.9929510916434339, 11.21034663311131929 ) ) ;
#21643=CARTESIAN_POINT ( 'NONE',  ( -35.50000000000000000, -112.8920926830253677, 2.874852253704053062 ) ) ;
#21647=CARTESIAN_POINT ( 'NONE',  ( -37.74901162816869515, -114.6652019342044042, 8.066024454178448266 ) ) ;
#21655=CARTESIAN_POINT ( 'NONE',  ( -34.50000000000000000, -113.0140978167138712, -0.4685323525984296800 ) ) ;
#21661=CARTESIAN_POINT ( 'NONE',  ( -37.89983305244309975, -114.9929510916434339, 12.92579853460519246 ) ) ;
#21664=CARTESIAN_POINT ( 'NONE',  ( -34.50000000000000000, -112.0140900043366088, -0.5935324770972457697 ) ) ;
#21667=CARTESIAN_POINT ( 'NONE',  ( -36.06250000000000711, -115.9929510916434481, 14.11852480586265024 ) ) ;
#21674=CARTESIAN_POINT ( 'NONE',  ( -38.00000000000000711, -115.9929510916434481, 12.59102132592609102 ) ) ;
#21696=CARTESIAN_POINT ( 'NONE',  ( -35.00000000000000000, -113.9407375970686900, 6.996475545821551734 ) ) ;
#21716=CARTESIAN_POINT ( 'NONE',  ( -36.87500000000098765, -115.9929510916434481, 14.11852480586265024 ) ) ;
#21727=CARTESIAN_POINT ( 'NONE',  ( -38.30190309005061522, -111.0245472910330022, 8.027725545821551734 ) ) ;
#21751=CARTESIAN_POINT ( 'NONE',  ( -34.50000000000000000, -112.2144317118258527, -1.239329810084414341 ) ) ;
#21752=CARTESIAN_POINT ( 'NONE',  ( -36.00976557831293690, -114.9929510916434339, 14.11852773550420359 ) ) ;
#21754=CARTESIAN_POINT ( 'NONE',  ( -35.50000000000000000, -113.9948283797722439, 10.50648163149984171 ) ) ;
#21756=CARTESIAN_POINT ( 'NONE',  ( -35.93867112612154813, -114.9929510916434339, 14.11732072679899197 ) ) ;
#21766=CARTESIAN_POINT ( 'NONE',  ( -36.24999999999983658, -114.9929510916434339, 13.11852480586264669 ) ) ;
#21769=CARTESIAN_POINT ( 'NONE',  ( -36.23083527818512550, -116.0245472910329880, 7.784774454178451819 ) ) ;
#21779=CARTESIAN_POINT ( 'NONE',  ( -40.02454729103296671, -115.1833782841879525, 6.659774454178448266 ) ) ;
#21790=CARTESIAN_POINT ( 'NONE',  ( -34.50000000000000000, -112.7319952733504635, 2.855726801009121463 ) ) ;
#21794=CARTESIAN_POINT ( 'NONE',  ( -35.50000000000000711, -114.0743172650041686, 9.508870970061893857 ) ) ;
#21797=CARTESIAN_POINT ( 'NONE',  ( -36.03906250000000000, -113.9929510916434339, 14.11852480586265024 ) ) ;
#21801=CARTESIAN_POINT ( 'NONE',  ( -34.50000000000000000, -113.9929510916434339, 12.60752341388803721 ) ) ;
#21804=CARTESIAN_POINT ( 'NONE',  ( -38.00000000000000711, -115.9929510916434481, 11.73841344789285657 ) ) ;
#21817=CARTESIAN_POINT ( 'NONE',  ( -35.50000000000000000, -113.0140978167137717, 0.8752176474015607166 ) ) ;
#21819=CARTESIAN_POINT ( 'NONE',  ( -37.74901162816869515, -114.6652019342044042, 8.066024454178448266 ) ) ;
#21821=CARTESIAN_POINT ( 'NONE',  ( -35.50000000000000711, -114.9929510916434339, 12.59652202191340642 ) ) ;
#21827=CARTESIAN_POINT ( 'NONE',  ( -35.50000000000000000, -111.4147656069378058, -1.853877267569947529 ) ) ;
#21830=CARTESIAN_POINT ( 'NONE',  ( -37.05926240293131713, -115.9999999999999858, 3.378524454178448710 ) ) ;
#21838=CARTESIAN_POINT ( 'NONE',  ( -34.50000000000000000, -115.0140978167138712, -0.6247823525984407267 ) ) ;
#21843=CARTESIAN_POINT ( 'NONE',  ( -35.50000000000000000, -113.9929510916433060, 10.50625754673589540 ) ) ;
#21848=CARTESIAN_POINT ( 'NONE',  ( -34.50000000000000000, -115.0795240838853886, -1.623175561345890472 ) ) ;
#21849=CARTESIAN_POINT ( 'NONE',  ( -35.50000000000000000, -114.2067765580549832, 8.517583185305328541 ) ) ;
#21856=CARTESIAN_POINT ( 'NONE',  ( -37.62959469683911351, -115.9929510916434481, 13.10254527216511633 ) ) ;
#21877=CARTESIAN_POINT ( 'NONE',  ( -38.45611840935523418, -112.6276912846090568, 9.433975545821551734 ) ) ;
#21881=CIRCLE ( 'NONE', #12690, 0.5000000000000004441 ) ;
#21890=CARTESIAN_POINT ( 'NONE',  ( -35.50000000000000711, -114.9929517792218689, 10.50900788599415314 ) ) ;
#21897=CARTESIAN_POINT ( 'NONE',  ( -36.01562499999997158, -115.9929510916434481, 14.11852480586265024 ) ) ;
#21907=CARTESIAN_POINT ( 'NONE',  ( -35.54388159064475872, -115.3723087153909432, 7.183975545821551734 ) ) ;
#21932=CARTESIAN_POINT ( 'NONE',  ( -34.50000000000000000, -112.9486715495423681, -1.623175561345890472 ) ) ;
#21933=CARTESIAN_POINT ( 'NONE',  ( -35.80421860361284558, -114.9929510916434339, 14.10650203519841916 ) ) ;
#21934=CARTESIAN_POINT ( 'NONE',  ( -35.50000000000000000, -113.9836614335179377, 10.50514867547815534 ) ) ;
#21937=CARTESIAN_POINT ( 'NONE',  ( -35.51674767832921731, -114.9929510916434339, 14.04194344061634503 ) ) ;
#21947=CARTESIAN_POINT ( 'NONE',  ( -34.00000000000000000, -114.0592624029313242, 3.003524454178448710 ) ) ;
#21956=CARTESIAN_POINT ( 'NONE',  ( -33.97545270896703329, -115.1833782841879810, 4.090225545821551734 ) ) ;
#21967=CARTESIAN_POINT ( 'NONE',  ( -34.50000000000000000, -117.0140978167138854, 0.0002176474015577929428 ) ) ;
#21973=CARTESIAN_POINT ( 'NONE',  ( -34.50000000000000000, -113.9929510916434339, 10.72628538622835670 ) ) ;
#21980=CARTESIAN_POINT ( 'NONE',  ( -34.50000000000000000, -113.9929510916432207, 10.50625754673563250 ) ) ;
#21981=CARTESIAN_POINT ( 'NONE',  ( -39.00000000000000711, -114.9929510916434339, 10.50625754673587231 ) ) ;
#21982=CARTESIAN_POINT ( 'NONE',  ( -35.50000000000000711, -114.9929296450195721, 10.49869535309826674 ) ) ;
#21994=CARTESIAN_POINT ( 'NONE',  ( -35.50000000000000000, -113.0140978167138712, 0.6252176474015680441 ) ) ;
#21996=CARTESIAN_POINT ( 'NONE',  ( -37.97545270896701908, -113.5265240346955977, 5.347274454178449155 ) ) ;
#22002=CARTESIAN_POINT ( 'NONE',  ( -35.50000000000000000, -115.2751396785629510, -2.608751991713152307 ) ) ;
#22006=CARTESIAN_POINT ( 'NONE',  ( -36.94073759706868287, -112.0000000000000142, 4.128524454178449155 ) ) ;
#22011=CARTESIAN_POINT ( 'NONE',  ( -34.50000000000000000, -112.1859307030124739, 1.448610958621386224 ) ) ;
#22021=CARTESIAN_POINT ( 'NONE',  ( -35.50000000000000000, -113.9929510916434339, 10.50625754673586876 ) ) ;
#22025=CARTESIAN_POINT ( 'NONE',  ( -34.50000000000000000, -111.0278007905855588, 1.116632271043183078 ) ) ;
#22027=CARTESIAN_POINT ( 'NONE',  ( -37.59808119975203766, -115.9929510916434481, 14.11551573851449071 ) ) ;
#22034=CARTESIAN_POINT ( 'NONE',  ( -35.50000000000000711, -114.1189822439768449, 9.514224058074130852 ) ) ;
#22054=CARTESIAN_POINT ( 'NONE',  ( -37.74901162816868805, -113.3347980657955958, 7.933975545821553510 ) ) ;
#22074=CARTESIAN_POINT ( 'NONE',  ( -39.00000206272865455, -115.9929510916434481, 12.61164896875035879 ) ) ;
#22082=CARTESIAN_POINT ( 'NONE',  ( -35.02454729103298803, -113.1123104723225197, 6.902725545821550845 ) ) ;
#22109=CARTESIAN_POINT ( 'NONE',  ( -34.50000000000000000, -114.8057644833805568, -1.624782352598427959 ) ) ;
#22110=CARTESIAN_POINT ( 'NONE',  ( -39.00000000000000711, -114.9929510916434339, 12.59652202191340820 ) ) ;
#22111=CARTESIAN_POINT ( 'NONE',  ( -38.00000000000000711, -114.9929510916434339, 11.73841344789285657 ) ) ;
#22113=CARTESIAN_POINT ( 'NONE',  ( -35.95093014754292682, -114.9929510916434339, 14.11777216781842448 ) ) ;
#22122=CARTESIAN_POINT ( 'NONE',  ( -34.02454729103298092, -115.3019030900506294, 3.097274454178448710 ) ) ;
#22132=CARTESIAN_POINT ( 'NONE',  ( -39.16322519054178741, -111.9205845034225177, 3.433975545821550845 ) ) ;
#22146=CARTESIAN_POINT ( 'NONE',  ( -34.50000000000000000, -116.7615919857705080, -1.632210089000343700 ) ) ;
#22149=CARTESIAN_POINT ( 'NONE',  ( -35.93473953453761283, -114.9929510916434339, 13.11451721564123574 ) ) ;
#22150=CARTESIAN_POINT ( 'NONE',  ( -35.07817881376918479, -113.9929510916434339, 13.81802396319203474 ) ) ;
#22154=CARTESIAN_POINT ( 'NONE',  ( -34.50000000000000000, -113.9929510916434339, 10.50625754673586876 ) ) ;
#22155=CARTESIAN_POINT ( 'NONE',  ( -39.00000000000000711, -114.9929510916434339, 11.91443571948719615 ) ) ;
#22157=CARTESIAN_POINT ( 'NONE',  ( -35.50000000000000711, -114.9927795562974069, 10.48735431211914815 ) ) ;
#22169=CARTESIAN_POINT ( 'NONE',  ( -35.50000000000000711, -115.1446187476384040, -1.616767172155725740 ) ) ;
#22171=CARTESIAN_POINT ( 'NONE',  ( -36.94073759706868287, -112.0000000000000142, 4.128524454178449155 ) ) ;
#22175=CARTESIAN_POINT ( 'NONE',  ( -35.50000000000000711, -112.3465879560236687, 1.629585756119413364 ) ) ;
#22178=CARTESIAN_POINT ( 'NONE',  ( -36.94073759706868287, -112.0000000000000142, 8.628524454178448266 ) ) ;
#22184=CARTESIAN_POINT ( 'NONE',  ( -34.50000000000000000, -115.0140978167138712, 0.0002176474015577929428 ) ) ;
#22190=CARTESIAN_POINT ( 'NONE',  ( -35.50000000000000000, -113.9929510916434197, 10.50625754673586876 ) ) ;
#22193=CARTESIAN_POINT ( 'NONE',  ( -34.50000000000000000, -112.8920926830253677, 2.874852253704053062 ) ) ;
#22195=CARTESIAN_POINT ( 'NONE',  ( -39.00000000000000000, -115.9929510916434481, 11.73841344789285657 ) ) ;
#22201=CARTESIAN_POINT ( 'NONE',  ( -38.00000000000000711, -115.9929510916434481, 12.50851088611646311 ) ) ;
#22223=CARTESIAN_POINT ( 'NONE',  ( -36.02454729103297382, -113.5265240346956261, 5.402725545821552622 ) ) ;
#22233=CARTESIAN_POINT ( 'NONE',  ( -35.50000000000000711, -112.0140978167138712, 0.7189676474015718188 ) ) ;
#22238=CARTESIAN_POINT ( 'NONE',  ( -35.50000000000000711, -114.0998638248492085, 9.511920366020609308 ) ) ;
#22243=CARTESIAN_POINT ( 'NONE',  ( -34.50000000000000000, -114.9929510916434339, 12.26648026267477221 ) ) ;
#22246=CARTESIAN_POINT ( 'NONE',  ( -37.42187499999996447, -115.9929510916434481, 14.11852480586265024 ) ) ;
#22258=CARTESIAN_POINT ( 'NONE',  ( -37.05926240293131713, -112.0000000000000142, 6.621475545821550845 ) ) ;
#22285=CARTESIAN_POINT ( 'NONE',  ( -34.50000000000000000, -115.8137639216009234, -1.239329810084483841 ) ) ;
#22287=CARTESIAN_POINT ( 'NONE',  ( -36.01562499999996447, -114.9929510916434339, 14.11852480586264846 ) ) ;
#22289=CARTESIAN_POINT ( 'NONE',  ( -35.50000000000000000, -113.9929510916434339, 10.51175824272318415 ) ) ;
#22291=CARTESIAN_POINT ( 'NONE',  ( -34.51922597003733273, -114.9929510916434339, 12.86289566494349224 ) ) ;
#22302=CARTESIAN_POINT ( 'NONE',  ( -34.92058450342251064, -116.1632251905417945, 6.191024454178448266 ) ) ;
#22305=CARTESIAN_POINT ( 'NONE',  ( -35.50000000000000711, -114.1807644833817648, -1.624782352598427959 ) ) ;
#22323=CARTESIAN_POINT ( 'NONE',  ( -34.50000000000000000, -117.0140978167138854, -0.1247823525984438492 ) ) ;
#22325=CARTESIAN_POINT ( 'NONE',  ( -35.99181955245763476, -114.9929510916434339, 13.11847460610632687 ) ) ;
#22328=CARTESIAN_POINT ( 'NONE',  ( -34.50000000000000000, -113.9929510916434339, 10.61627146648203990 ) ) ;
#22331=CARTESIAN_POINT ( 'NONE',  ( -34.50000000000000000, -113.9929510916434339, 12.57451923796416260 ) ) ;
#22334=CARTESIAN_POINT ( 'NONE',  ( -35.50000000000000711, -114.8847986568751907, 10.03799953695244618 ) ) ;
#22345=CARTESIAN_POINT ( 'NONE',  ( -35.50000000000000000, -115.0304602784513293, -0.6247823525985405357 ) ) ;
#22347=CARTESIAN_POINT ( 'NONE',  ( -38.97545270896704039, -113.1123104723225197, 3.847274454178449599 ) ) ;
#22351=CARTESIAN_POINT ( 'NONE',  ( -35.50000000000000711, -112.0140978167138712, 0.8127176474015721519 ) ) ;
#22360=CARTESIAN_POINT ( 'NONE',  ( -34.50000000000000000, -112.0140978167138712, 0.8127176474015721519 ) ) ;
#22365=MANIFOLD_SOLID_BREP ( 'Sweep3', #23278 ) ;
#22366=EDGE_CURVE ( 'NONE', #34373, #14462, #17031, .T. ) ;
#22367=CARTESIAN_POINT ( 'NONE',  ( -35.50000000000000000, -113.9929510916434339, 12.39849696637031684 ) ) ;
#22370=CARTESIAN_POINT ( 'NONE',  ( -34.50000000000000000, -113.1451905347060460, 2.905063584339864668 ) ) ;
#22371=CARTESIAN_POINT ( 'NONE',  ( -39.00000000000000000, -115.9929510916434481, 12.53051367006571937 ) ) ;
#22396=CARTESIAN_POINT ( 'NONE',  ( -37.97545270896702618, -114.4734759653044023, 3.152725545821551734 ) ) ;
#22402=CARTESIAN_POINT ( 'NONE',  ( -35.50000000000000711, -116.0140896356112989, -0.6575071456984549201 ) ) ;
#22406=CARTESIAN_POINT ( 'NONE',  ( -35.50000000000000711, -114.1152303497977414, 9.513755561829650986 ) ) ;
#22417=CARTESIAN_POINT ( 'NONE',  ( -35.50000000000000000, -114.2253558743059330, 8.519800927820798009 ) ) ;
#22418=CARTESIAN_POINT ( 'NONE',  ( -35.50000000000000711, -112.0157046079661995, -0.6902086197697556713 ) ) ;
#22426=CARTESIAN_POINT ( 'NONE',  ( -37.05926240293131713, -112.0000000000000142, 8.121475545821549957 ) ) ;
#22455=CARTESIAN_POINT ( 'NONE',  ( -34.50000000000000000, -112.9977353549762000, -0.6247823525983134951 ) ) ;
#22458=CARTESIAN_POINT ( 'NONE',  ( -34.50000000000000000, -114.2114213871176958, 8.518137620934190579 ) ) ;
#22463=CARTESIAN_POINT ( 'NONE',  ( -37.24999999999992895, -114.9929510916434339, 14.11852480586264846 ) ) ;
#22472=CARTESIAN_POINT ( 'NONE',  ( -38.00000000000000711, -114.9929510916434339, 11.91443571948719615 ) ) ;
#22474=CARTESIAN_POINT ( 'NONE',  ( -34.92058450342251064, -116.1632251905417945, 4.691024454178447378 ) ) ;
#22476=CARTESIAN_POINT ( 'NONE',  ( -35.50000000000000711, -114.8474311500471572, -1.624782352598427959 ) ) ;
#22496=CARTESIAN_POINT ( 'NONE',  ( -34.50000000000000000, -116.2431927316855109, -2.224114562372550008 ) ) ;
#22500=CARTESIAN_POINT ( 'NONE',  ( -35.60016694755736921, -114.9929510916434339, 12.92579853460621209 ) ) ;
#22501=CARTESIAN_POINT ( 'NONE',  ( -34.50000000000000000, -114.1712995509219724, 9.522174004479579068 ) ) ;
#22504=CARTESIAN_POINT ( 'NONE',  ( -34.50000000000000000, -113.9929510916434339, 11.38636890470581164 ) ) ;
#22506=CARTESIAN_POINT ( 'NONE',  ( -38.00000000000000711, -115.9929510916434481, 12.26648026267477221 ) ) ;
#22519=CARTESIAN_POINT ( 'NONE',  ( -35.50000000000000000, -113.0140978167139991, -0.6247823525984269599 ) ) ;
#22521=CARTESIAN_POINT ( 'NONE',  ( -36.23083527818512550, -116.0245472910329880, 3.284774454178449155 ) ) ;
#22529=CARTESIAN_POINT ( 'NONE',  ( -35.50000000000000711, -112.6043641208289188, 1.789429170677330649 ) ) ;
#22536=CARTESIAN_POINT ( 'NONE',  ( -34.50000000000000000, -115.0140978167138712, 0.3752176474015737617 ) ) ;
#22544=CARTESIAN_POINT ( 'NONE',  ( -35.50000000000000000, -113.9929510916434339, 10.50625754673586876 ) ) ;
#22547=CARTESIAN_POINT ( 'NONE',  ( -34.50000000000000000, -116.0140978167138712, 0.8752176474015622709 ) ) ;
#22548=CARTESIAN_POINT ( 'NONE',  ( -38.98077402996267438, -115.9929510916434481, 12.86289566494346204 ) ) ;
#22571=CARTESIAN_POINT ( 'NONE',  ( -36.64504884055821776, -112.9754527089670688, 3.715225545821552178 ) ) ;
#22578=CARTESIAN_POINT ( 'NONE',  ( -35.50000000000000711, -114.6807644833805000, -1.624782352598427959 ) ) ;
#22581=CARTESIAN_POINT ( 'NONE',  ( -35.50000000000000711, -114.9929501463477663, 10.50247632894551231 ) ) ;
#22585=CARTESIAN_POINT ( 'NONE',  ( -34.50000000000000000, -114.4026847875275337, 9.592046023459676718 ) ) ;
#22588=CARTESIAN_POINT ( 'NONE',  ( -35.50000000000000000, -115.9929510916434481, 10.68227981832981044 ) ) ;
#22598=CARTESIAN_POINT ( 'NONE',  ( -38.99999999999999289, -114.0592624029313242, 7.746475545821551734 ) ) ;
#22623=CARTESIAN_POINT ( 'NONE',  ( -34.50000000000000000, -115.0140978167139707, -0.6091573525984161908 ) ) ;
#22627=CARTESIAN_POINT ( 'NONE',  ( -39.00000000000000711, -114.9929510916434339, 12.56351784598954779 ) ) ;
#22631=CARTESIAN_POINT ( 'NONE',  ( -34.50000000000000000, -114.3049001878960240, 8.530677542735578101 ) ) ;
#22640=CARTESIAN_POINT ( 'NONE',  ( -39.16322519054179452, -116.0794154965774823, 5.066024454178449155 ) ) ;
#22642=CARTESIAN_POINT ( 'NONE',  ( -35.50000000000000711, -113.4307644833805000, -1.624782352598427959 ) ) ;
#22658=CARTESIAN_POINT ( 'NONE',  ( -38.99999999999999289, -114.0592624029313242, 7.746475545821551734 ) ) ;
#22665=CARTESIAN_POINT ( 'NONE',  ( -35.50000000000000000, -111.0140978167138570, 0.8127176474015720409 ) ) ;
#22668=CARTESIAN_POINT ( 'NONE',  ( -37.43749999999998579, -114.9929510916434339, 13.11852480586264669 ) ) ;
#22669=CARTESIAN_POINT ( 'NONE',  ( -37.88878409051687157, -113.9929510916434339, 14.07058620477052280 ) ) ;
#22672=CARTESIAN_POINT ( 'NONE',  ( -35.90191880024782023, -113.9929510916434339, 14.11551573851449071 ) ) ;
#22675=CARTESIAN_POINT ( 'NONE',  ( -35.69272627125609176, -114.9929510916434339, 13.01835785830562209 ) ) ;
#22691=CARTESIAN_POINT ( 'NONE',  ( -35.50000000000000000, -115.0140978167138712, -0.5622823525984408377 ) ) ;
#22693=CARTESIAN_POINT ( 'NONE',  ( -35.54388159064475872, -112.6276912846090568, 5.816024454178449155 ) ) ;
#22697=CARTESIAN_POINT ( 'NONE',  ( -35.54388159064475872, -112.6276912846090568, 7.316024454178449155 ) ) ;
#22701=CARTESIAN_POINT ( 'NONE',  ( -35.50000000000000711, -112.1222502514821144, 1.343475657184566296 ) ) ;
#22704=CARTESIAN_POINT ( 'NONE',  ( -38.99999999999999289, -113.9407375970686900, 5.253524454178449155 ) ) ;
#22709=CARTESIAN_POINT ( 'NONE',  ( -34.50000000000000000, -115.0140978167138712, -0.4685323525984310122 ) ) ;
#22721=CARTESIAN_POINT ( 'NONE',  ( -36.15625000000007816, -113.9929510916434339, 13.11852480586264846 ) ) ;
#22724=CARTESIAN_POINT ( 'NONE',  ( -34.50000000000000000, -111.0140978167138570, -0.1247823525984260717 ) ) ;
#22726=CARTESIAN_POINT ( 'NONE',  ( -35.50640865667917723, -115.9929510916434481, 12.69998175888958691 ) ) ;
#22752=CARTESIAN_POINT ( 'NONE',  ( -37.66520193420439711, -114.7490116281687023, 7.558975545821551734 ) ) ;
#22760=CARTESIAN_POINT ( 'NONE',  ( -35.97955704204053262, -114.9929510916434339, 13.11812344617474579 ) ) ;
#22772=CARTESIAN_POINT ( 'NONE',  ( -39.00000000000000000, -115.9929510916434481, 10.50625754673587053 ) ) ;
#22773=CARTESIAN_POINT ( 'NONE',  ( -35.50000000000000711, -112.0140978167138712, 0.8127176474015721519 ) ) ;
#22783=CARTESIAN_POINT ( 'NONE',  ( -36.02454729103297382, -113.5265240346956261, 5.402725545821552622 ) ) ;
#22793=CARTESIAN_POINT ( 'NONE',  ( -35.81662171581203324, -110.9754527089670546, 5.215225545821552622 ) ) ;
#22800=SHAPE_DEFINITION_REPRESENTATION ( #28193, #31216 ) ;
#22810=CARTESIAN_POINT ( 'NONE',  ( -34.50000000000000000, -115.0140978167138712, -0.3747823525984421145 ) ) ;
#22814=CARTESIAN_POINT ( 'NONE',  ( -34.50000000000000000, -115.9926080209513657, 10.46845107750242398 ) ) ;
#22817=CARTESIAN_POINT ( 'NONE',  ( -37.88768952767750164, -115.9754527089670262, 1.972274454178448710 ) ) ;
#22818=CARTESIAN_POINT ( 'NONE',  ( -34.50000000000000000, -114.2183886307118428, 8.518969274377507617 ) ) ;
#22831=CARTESIAN_POINT ( 'NONE',  ( -38.30190309005061522, -111.0245472910330022, 3.527725545821551734 ) ) ;
#22833=CARTESIAN_POINT ( 'NONE',  ( -35.50000000000000711, -116.0140896356112989, -0.6575071456984549201 ) ) ;
#22844=CARTESIAN_POINT ( 'NONE',  ( -38.37230871539094323, -115.4561184093552413, 6.058975545821551734 ) ) ;
#22850=CARTESIAN_POINT ( 'NONE',  ( -35.50000000000000000, -116.9119893297194324, -1.269118781492768910 ) ) ;
#22854=CARTESIAN_POINT ( 'NONE',  ( -37.42187499999997158, -114.9929510916434339, 13.11852480586264669 ) ) ;
#22856=CARTESIAN_POINT ( 'NONE',  ( -39.00000000000000000, -113.9929510916434339, 12.59652202191340820 ) ) ;
#22860=CARTESIAN_POINT ( 'NONE',  ( -37.56132887387857267, -113.9929510916434339, 14.11732072679899197 ) ) ;
#22862=CARTESIAN_POINT ( 'NONE',  ( -35.50000000000000711, -114.9929510916434339, 12.59652202191340642 ) ) ;
#22869=CARTESIAN_POINT ( 'NONE',  ( -35.50000000000000711, -114.9819937217110635, 10.35556074009299188 ) ) ;
#22880=CARTESIAN_POINT ( 'NONE',  ( -35.50000000000000000, -115.0140978167138712, 0.3752176474015736507 ) ) ;
#22882=CARTESIAN_POINT ( 'NONE',  ( -35.00000000000000000, -114.0592624029313242, 3.003524454178448710 ) ) ;
#22885=CARTESIAN_POINT ( 'NONE',  ( -37.88768952767750164, -115.9754527089670262, 4.972274454178448266 ) ) ;
#22887=CARTESIAN_POINT ( 'NONE',  ( -35.50000000000000711, -112.0140900043366088, -0.5935324770972457697 ) ) ;
#22895=CARTESIAN_POINT ( 'NONE',  ( -34.50000000000000000, -115.1770117227680998, -1.611965039240062181 ) ) ;
#22896=CARTESIAN_POINT ( 'NONE',  ( -35.50000000000000711, -112.4434344552011282, 1.705278471174987986 ) ) ;
#22903=CARTESIAN_POINT ( 'NONE',  ( -35.99181955245763476, -113.9929510916434339, 13.11847460610632510 ) ) ;
#22904=CARTESIAN_POINT ( 'NONE',  ( -34.50000000000000000, -112.8356783780338759, 1.859636627348750348 ) ) ;
#22908=CARTESIAN_POINT ( 'NONE',  ( -36.87500000000098765, -113.9929510916434339, 13.11852480586264846 ) ) ;
#22909=CARTESIAN_POINT ( 'NONE',  ( -35.50000000000000000, -115.9915791193162420, 10.43066258751475139 ) ) ;
#22931=CARTESIAN_POINT ( 'NONE',  ( -36.02454729103298092, -114.4734759653044307, 1.597274454178448932 ) ) ;
#22941=CARTESIAN_POINT ( 'NONE',  ( -35.50000000000000711, -114.9929510916434339, 10.61627146648203812 ) ) ;
#22947=CARTESIAN_POINT ( 'NONE',  ( -34.50000000000000000, -114.9860996047076895, 10.38555023491505835 ) ) ;
#22953=CARTESIAN_POINT ( 'NONE',  ( -39.00000000000000000, -115.9929510916434481, 10.85830208992306822 ) ) ;
#22954=CARTESIAN_POINT ( 'NONE',  ( -35.50000000000000711, -113.1256619669233885, 1.895633585076891947 ) ) ;
#22963=CARTESIAN_POINT ( 'NONE',  ( -36.64504884055821776, -112.9754527089670688, 6.715225545821551734 ) ) ;
#22971=CARTESIAN_POINT ( 'NONE',  ( -35.81662171581204746, -117.0245472910329738, 6.284774454178449155 ) ) ;
#22989=CARTESIAN_POINT ( 'NONE',  ( -34.50000000000000000, -112.8356783780338759, 1.859636627348750348 ) ) ;
#22993=CARTESIAN_POINT ( 'NONE',  ( -34.50000000000000000, -115.9929510916434481, 10.68227981832981044 ) ) ;
#22997=CARTESIAN_POINT ( 'NONE',  ( -38.98797722933582577, -114.9929510916434339, 12.81430620224974959 ) ) ;
#23008=CARTESIAN_POINT ( 'NONE',  ( -33.97545270896703329, -115.1833782841879810, 5.590225545821552622 ) ) ;
#23011=CARTESIAN_POINT ( 'NONE',  ( -35.50000000000000711, -116.0140978167138712, -0.3122823525984417259 ) ) ;
#23022=CARTESIAN_POINT ( 'NONE',  ( -38.99999999999999289, -114.0592624029313242, 3.246475545821551734 ) ) ;
#23027=CARTESIAN_POINT ( 'NONE',  ( -35.50000000000000000, -116.2431927316855109, -2.224114562372550008 ) ) ;
#23033=CARTESIAN_POINT ( 'NONE',  ( -37.99959864031215773, -114.9929510916434339, 12.63896776382213538 ) ) ;
#23035=CARTESIAN_POINT ( 'NONE',  ( -39.00000000000000000, -113.9929510916434339, 12.44250253426875119 ) ) ;
#23038=CARTESIAN_POINT ( 'NONE',  ( -37.34375000000001421, -113.9929510916434339, 14.11852480586265024 ) ) ;
#23040=CARTESIAN_POINT ( 'NONE',  ( -36.06250000000002132, -114.9929510916434339, 13.11852480586264669 ) ) ;
#23046=CARTESIAN_POINT ( 'NONE',  ( -35.50000000000000711, -114.9912366357066986, 10.44580456020104720 ) ) ;
#23053=CARTESIAN_POINT ( 'NONE',  ( -35.50000000000000000, -114.8057644833805853, -0.6247823525984269599 ) ) ;
#23060=CARTESIAN_POINT ( 'NONE',  ( -38.97545270896704039, -113.1123104723225197, 2.347274454178448710 ) ) ;
#23063=CARTESIAN_POINT ( 'NONE',  ( -35.50000000000000711, -112.0651520602111191, -0.9469505670458575608 ) ) ;
#23068=SURFACE_STYLE_FILL_AREA ( #15132 ) ;
#23072=CARTESIAN_POINT ( 'NONE',  ( -34.50000000000000000, -116.0140978167138712, -0.3747823525984422255 ) ) ;
#23073=CARTESIAN_POINT ( 'NONE',  ( -35.50000000000000711, -113.8159288351371714, 1.978028123174813802 ) ) ;
#23078=CARTESIAN_POINT ( 'NONE',  ( -37.58145695302688694, -113.9929510916434339, 13.11211614918362756 ) ) ;
#23083=CARTESIAN_POINT ( 'NONE',  ( -35.50000000000000000, -113.9929510916434339, 10.61627146648203990 ) ) ;
#23084=CARTESIAN_POINT ( 'NONE',  ( -35.50000000000000000, -115.9929510916434481, 12.53051367006571581 ) ) ;
#23094=CARTESIAN_POINT ( 'NONE',  ( -35.50000000000000711, -113.0796441757086939, 1.890140615870383956 ) ) ;
#23102=CARTESIAN_POINT ( 'NONE',  ( -34.50000000000000000, -111.7850029017436810, -2.224114562373086912 ) ) ;
#23107=CARTESIAN_POINT ( 'NONE',  ( -36.02454729103298092, -114.4734759653044307, 4.597274454178449155 ) ) ;
#23116=CARTESIAN_POINT ( 'NONE',  ( -34.50000000000000000, -113.3822401464312719, 0.9191614010536472978 ) ) ;
#23122=CARTESIAN_POINT ( 'NONE',  ( -35.56312645773537895, -114.9929510916434339, 12.87038173996308998 ) ) ;
#23125=CARTESIAN_POINT ( 'NONE',  ( -35.98977351030467986, -114.9929510916434339, 14.11852173794918386 ) ) ;
#23130=CARTESIAN_POINT ( 'NONE',  ( -35.50000000000000000, -115.9929492010520846, 10.50058572605509966 ) ) ;
#23132=CARTESIAN_POINT ( 'NONE',  ( -35.50000000000000711, -112.0209493036498287, 0.9959249592223760050 ) ) ;
#23144=CARTESIAN_POINT ( 'NONE',  ( -36.64504884055821776, -112.9754527089670688, 9.715225545821551734 ) ) ;
#23154=CARTESIAN_POINT ( 'NONE',  ( -39.97545270896702618, -115.3019030900506152, 9.152725545821551734 ) ) ;
#23174=CARTESIAN_POINT ( 'NONE',  ( -34.50000000000000000, -115.0140978167138712, -0.6247823525984403936 ) ) ;
#23177=CARTESIAN_POINT ( 'NONE',  ( -34.50000000000000000, -114.3049001878960240, 8.530677542735578101 ) ) ;
#23180=CARTESIAN_POINT ( 'NONE',  ( -38.37230871539094323, -112.5438815906447729, 2.441024454178448710 ) ) ;
#23181=CARTESIAN_POINT ( 'NONE',  ( -37.69578139638701941, -114.9929510916434339, 14.10650203519847778 ) ) ;
#23192=CARTESIAN_POINT ( 'NONE',  ( -39.16322519054178741, -111.9205845034225177, 4.933975545821551734 ) ) ;
#23194=CARTESIAN_POINT ( 'NONE',  ( -35.50000000000000000, -113.0140978167138712, -0.5622823525984297355 ) ) ;
#23205=CARTESIAN_POINT ( 'NONE',  ( -38.99999999999999289, -114.0592624029313242, 6.246475545821550845 ) ) ;
#23210=CARTESIAN_POINT ( 'NONE',  ( -35.50000000000000000, -112.0066700803175763, -2.372276521656937920 ) ) ;
#23217=CARTESIAN_POINT ( 'NONE',  ( -37.56526046546250086, -114.9929510916434339, 13.11451721564129258 ) ) ;
#23218=CARTESIAN_POINT ( 'NONE',  ( -34.50000000000000000, -114.1068310684433129, 9.512752019463897923 ) ) ;
#23221=CARTESIAN_POINT ( 'NONE',  ( -38.99984940073100148, -113.9929510916434339, 12.64306614848957544 ) ) ;
#23223=CARTESIAN_POINT ( 'NONE',  ( -37.42187499999997158, -114.9929510916434339, 13.11852480586264669 ) ) ;
#23230=CARTESIAN_POINT ( 'NONE',  ( -35.50000000000000711, -114.9929510916434339, 11.21034663311131929 ) ) ;
#23232=CARTESIAN_POINT ( 'NONE',  ( -38.99999999999999289, -113.9407375970686900, 2.253524454178449155 ) ) ;
#23238=CARTESIAN_POINT ( 'NONE',  ( -34.50000000000000000, -113.0140978167137717, 0.8903425666012282358 ) ) ;
#23242=CARTESIAN_POINT ( 'NONE',  ( -35.54388159064475872, -112.6276912846090568, 2.816024454178448710 ) ) ;
#23244=CARTESIAN_POINT ( 'NONE',  ( -35.50000000000000711, -112.0140978167138712, -0.3122823525984337878 ) ) ;
#23252=CARTESIAN_POINT ( 'NONE',  ( -34.50000000000000000, -112.8835768857893527, -1.616767172155725740 ) ) ;
#23253=CARTESIAN_POINT ( 'NONE',  ( -35.50000000000000711, -112.7765286249690035, 1.847058736912741583 ) ) ;
#23257=CARTESIAN_POINT ( 'NONE',  ( -37.99899697755054717, -113.9929510916434339, 12.65121853911336913 ) ) ;
#23260=CARTESIAN_POINT ( 'NONE',  ( -36.07812499999994316, -113.9929510916434339, 13.11852480586264846 ) ) ;
#23262=CARTESIAN_POINT ( 'NONE',  ( -35.50000000000000000, -115.9056129652226872, 9.909279992139808257 ) ) ;
#23271=CARTESIAN_POINT ( 'NONE',  ( -35.50000000000000711, -112.0221129971568104, -0.7553032835231431319 ) ) ;
#23275=CARTESIAN_POINT ( 'NONE',  ( -35.50000000000000711, -114.8847986568751907, 10.03799953695244618 ) ) ;
#23278=CLOSED_SHELL ( 'NONE', ( #29282, #12587, #1298, #15166, #27967, #7790, #16534, #13405 ) ) ;
#23281=CARTESIAN_POINT ( 'NONE',  ( -34.50000000000000000, -113.3474311500483935, -2.624782352598442614 ) ) ;
#23285=CARTESIAN_POINT ( 'NONE',  ( -37.97545270896701908, -113.5265240346955977, 3.847274454178448710 ) ) ;
#23291=CARTESIAN_POINT ( 'NONE',  ( -34.50000000000000000, -113.4742757288593964, 0.9301473394660054739 ) ) ;
#23297=CARTESIAN_POINT ( 'NONE',  ( -35.99181955245763476, -114.9929510916434339, 13.11847460610632687 ) ) ;
#23300=CARTESIAN_POINT ( 'NONE',  ( -36.12500000000014211, -114.9929510916434339, 14.11852480586264846 ) ) ;
#23309=CARTESIAN_POINT ( 'NONE',  ( -35.50000000000000000, -115.9929510916434481, 11.91443571948720148 ) ) ;
#23310=CARTESIAN_POINT ( 'NONE',  ( -35.50000000000000711, -113.0974311500471714, -1.624782352598427959 ) ) ;
#23321=CARTESIAN_POINT ( 'NONE',  ( -36.02454729103297382, -113.5265240346956261, 8.402725545821549957 ) ) ;
#23331=CARTESIAN_POINT ( 'NONE',  ( -34.92058450342249643, -111.8367748094582197, 8.308975545821549957 ) ) ;
#23352=CARTESIAN_POINT ( 'NONE',  ( -36.24999999999983658, -115.9929510916434481, 14.11852480586265024 ) ) ;
#23358=CARTESIAN_POINT ( 'NONE',  ( -37.74437085908087397, -114.9929510916434339, 14.09929883582536903 ) ) ;
#23367=CARTESIAN_POINT ( 'NONE',  ( -35.69809690994938478, -111.0245472910330022, 8.722274454178450043 ) ) ;
#23370=CARTESIAN_POINT ( 'NONE',  ( -35.50000000000000000, -113.0140978167140702, 0.8752176474015694874 ) ) ;
#23385=CARTESIAN_POINT ( 'NONE',  ( -35.62769128460905677, -112.5438815906447729, 3.808975545821551290 ) ) ;
#23393=CARTESIAN_POINT ( 'NONE',  ( -35.50000000000000000, -117.0140978167138854, -0.3747823525984422255 ) ) ;
#23399=CARTESIAN_POINT ( 'NONE',  ( -38.00000000000000711, -114.9929510916434339, 12.59102132592608925 ) ) ;
#23401=CARTESIAN_POINT ( 'NONE',  ( -34.50000000000000000, -114.4026847875275337, 9.592046023459676718 ) ) ;
#23405=CARTESIAN_POINT ( 'NONE',  ( -37.43749999999998579, -114.9929510916434339, 13.11852480586264669 ) ) ;
#23408=CARTESIAN_POINT ( 'NONE',  ( -37.43749999999998579, -113.9929510916434339, 14.11852480586265024 ) ) ;
#23410=CARTESIAN_POINT ( 'NONE',  ( -37.46874999999996447, -114.9929510916434339, 13.11852480586264669 ) ) ;
#23416=CARTESIAN_POINT ( 'NONE',  ( -35.60016694755736921, -114.9929510916434339, 12.92579853460621209 ) ) ;
#23424=CARTESIAN_POINT ( 'NONE',  ( -34.50000000000000000, -113.0140978167138712, -0.5622823525984297355 ) ) ;
#23428=CARTESIAN_POINT ( 'NONE',  ( -38.45611840935523418, -115.3723087153909432, 3.566024454178448710 ) ) ;
#23433=CARTESIAN_POINT ( 'NONE',  ( -35.50000000000000711, -115.6286452741999113, -1.424448457485488095 ) ) ;
#23444=CARTESIAN_POINT ( 'NONE',  ( -34.50000000000000000, -114.1807644833817648, -1.624782352598427959 ) ) ;
#23445=CARTESIAN_POINT ( 'NONE',  ( -35.50000000000000711, -112.0141053790792114, 0.9054673897245171243 ) ) ;
#23453=CARTESIAN_POINT ( 'NONE',  ( -35.52552712174883709, -113.9929510916434339, 12.77960891308624625 ) ) ;
#23455=CARTESIAN_POINT ( 'NONE',  ( -35.60016694755736211, -113.9929510916434339, 12.92579853460621386 ) ) ;
#23456=CARTESIAN_POINT ( 'NONE',  ( -35.50000000000000000, -115.9926080209513657, 10.46845107750242398 ) ) ;
#23467=CARTESIAN_POINT ( 'NONE',  ( -35.50000000000000711, -113.8474311500459777, -1.624782352598427959 ) ) ;
#23474=CARTESIAN_POINT ( 'NONE',  ( -34.50000000000000000, -117.0140978167138854, 0.3752176474015737617 ) ) ;
#23478=CARTESIAN_POINT ( 'NONE',  ( -36.64504884055823908, -115.0245472910329880, 3.284774454178449155 ) ) ;
#23482=CARTESIAN_POINT ( 'NONE',  ( -35.50000000000000000, -113.4307644833805142, -0.6247823525984269599 ) ) ;
#23487=CARTESIAN_POINT ( 'NONE',  ( -36.87500000000098055, -114.9929510916434339, 13.11852480586264669 ) ) ;
#23490=CARTESIAN_POINT ( 'NONE',  ( -34.51202277066418844, -114.9929510916434339, 12.81430620224972294 ) ) ;
#23495=CARTESIAN_POINT ( 'NONE',  ( -36.12500000000014211, -115.9929510916434481, 13.11852480586264846 ) ) ;
#23496=CARTESIAN_POINT ( 'NONE',  ( -35.50000000000000711, -116.0140978167138712, -0.3747823525984422255 ) ) ;
#23507=CARTESIAN_POINT ( 'NONE',  ( -37.47347596530441649, -113.0245472910329880, 9.527725545821551734 ) ) ;
#23511=EDGE_LOOP ( 'NONE', ( #8511, #8241 ) ) ;
#23514=CARTESIAN_POINT ( 'NONE',  ( -38.18337828418796676, -117.0245472910329738, 7.465225545821552622 ) ) ;
#23535=CARTESIAN_POINT ( 'NONE',  ( -35.93867112612154102, -115.9929510916434481, 14.11732072679899197 ) ) ;
#23537=CARTESIAN_POINT ( 'NONE',  ( -35.54388159064475872, -112.6276912846090568, 2.816024454178448710 ) ) ;
#23538=CARTESIAN_POINT ( 'NONE',  ( -34.54793860109200665, -115.9929510916434481, 13.00730889637958221 ) ) ;
#23547=CARTESIAN_POINT ( 'NONE',  ( -34.83677480945819838, -111.9205845034225462, 8.816024454178446490 ) ) ;
#23550=CARTESIAN_POINT ( 'NONE',  ( -35.50000000000000000, -113.0140978167141128, -0.6247823525984907977 ) ) ;
#23571=CARTESIAN_POINT ( 'NONE',  ( -35.50000000000000000, -113.1807644833805426, -2.624782352598442614 ) ) ;
#23579=CARTESIAN_POINT ( 'NONE',  ( -34.50000000000000000, -114.9929510916434339, 11.73841344789270202 ) ) ;
#23581=CARTESIAN_POINT ( 'NONE',  ( -37.99359134332094357, -114.9929510916434339, 12.69998175888958158 ) ) ;
#23585=CARTESIAN_POINT ( 'NONE',  ( -34.50000000000000000, -114.8847986568751907, 10.03799953695244618 ) ) ;
#23587=CARTESIAN_POINT ( 'NONE',  ( -37.99959864031215773, -114.9929510916434339, 12.63896776382213538 ) ) ;
#23593=CARTESIAN_POINT ( 'NONE',  ( -35.69272627125609176, -114.9929510916434339, 13.01835785830562209 ) ) ;
#23601=CARTESIAN_POINT ( 'NONE',  ( -34.50000000000000000, -113.0140978167138712, -0.3747823525984258497 ) ) ;
#23604=CARTESIAN_POINT ( 'NONE',  ( -35.54388159064475872, -112.6276912846090568, 8.816024454178448266 ) ) ;
#23608=CARTESIAN_POINT ( 'NONE',  ( -34.92058450342251064, -116.1632251905417945, 3.191024454178448710 ) ) ;
#23611=CARTESIAN_POINT ( 'NONE',  ( -35.50000000000000711, -112.1403507321855528, -1.128496220798856253 ) ) ;
#23624=CARTESIAN_POINT ( 'NONE',  ( -34.50000000000000000, -112.0651520602111191, -0.9469505670458575608 ) ) ;
#23631=CARTESIAN_POINT ( 'NONE',  ( -34.50000000000000000, -113.9929510916433060, 10.50625754673589540 ) ) ;
#23634=CARTESIAN_POINT ( 'NONE',  ( -35.56312645773537895, -113.9929510916434339, 12.87038173996308998 ) ) ;
#23635=CARTESIAN_POINT ( 'NONE',  ( -37.99994980024369085, -115.9929510916434481, 12.62670525340494621 ) ) ;
#23649=CARTESIAN_POINT ( 'NONE',  ( -35.50000000000000711, -112.0140978167138712, 0.0002176474015661141945 ) ) ;
#23652=CARTESIAN_POINT ( 'NONE',  ( -35.50000000000000711, -114.1302255537607095, 9.515717283514957714 ) ) ;
#23656=CARTESIAN_POINT ( 'NONE',  ( -34.50000000000000000, -113.0765974847181781, -2.624803185604914102 ) ) ;
#23661=CARTESIAN_POINT ( 'NONE',  ( -36.02454729103297382, -113.5265240346956261, 8.402725545821549957 ) ) ;
#23664=CARTESIAN_POINT ( 'NONE',  ( -35.50000000000000000, -115.0140978167138712, 0.8752176474015623819 ) ) ;
#23670=CARTESIAN_POINT ( 'NONE',  ( -37.99974912065192711, -114.9929510916434339, 12.63488142334838571 ) ) ;
#23672=CARTESIAN_POINT ( 'NONE',  ( -34.54793860109200665, -114.9929510916434339, 13.00730889637958221 ) ) ;
#23676=CARTESIAN_POINT ( 'NONE',  ( -36.07812499999994316, -115.9929510916434481, 13.11852480586264846 ) ) ;
#23677=CARTESIAN_POINT ( 'NONE',  ( -35.50000000000000711, -116.0140978167138712, -0.1247823525984439463 ) ) ;
#23689=CARTESIAN_POINT ( 'NONE',  ( -36.25098837183129774, -113.3347980657956242, 2.816024454178448710 ) ) ;
#23697=CARTESIAN_POINT ( 'NONE',  ( -38.18337828418796676, -117.0245472910329738, 8.965225545821551734 ) ) ;
#23716=CARTESIAN_POINT ( 'NONE',  ( -34.49999793727135966, -115.9929510916434481, 12.61164896875036767 ) ) ;
#23718=CARTESIAN_POINT ( 'NONE',  ( -37.05926240293131713, -115.9999999999999858, 3.378524454178448710 ) ) ;
#23719=CARTESIAN_POINT ( 'NONE',  ( -34.50000000000000000, -115.7766462221073454, 9.569741527169023598 ) ) ;
#23731=CARTESIAN_POINT ( 'NONE',  ( -36.23083527818512550, -111.9754527089670404, 5.215225545821551734 ) ) ;
#23733=CARTESIAN_POINT ( 'NONE',  ( -35.50000000000000711, -116.0140978167138712, 0.8752176474015622709 ) ) ;
#23744=CARTESIAN_POINT ( 'NONE',  ( -35.00000000000000000, -113.9407375970690310, 9.996475545821589037 ) ) ;
#23750=CARTESIAN_POINT ( 'NONE',  ( -35.50000000000000711, -113.6318576702834804, 1.956056246348823580 ) ) ;
#23758=CARTESIAN_POINT ( 'NONE',  ( -34.50000000000000000, -112.8655373925166572, 1.864575885149403423 ) ) ;
#23760=CARTESIAN_POINT ( 'NONE',  ( -34.50000000000000000, -114.9929510916434339, 10.85830208992344303 ) ) ;
#23763=CARTESIAN_POINT ( 'NONE',  ( -35.91854304697313438, -114.9929510916434339, 13.11211614918345703 ) ) ;
#23765=CARTESIAN_POINT ( 'NONE',  ( -34.50000000000000000, -114.9929510916434339, 10.52000928670414126 ) ) ;
#23767=CARTESIAN_POINT ( 'NONE',  ( -38.00000000000000711, -114.9929510916434339, 12.59652202191340820 ) ) ;
#23775=CARTESIAN_POINT ( 'NONE',  ( -36.00585935943767169, -114.9929510916434339, 13.11852578240983291 ) ) ;
#23778=CARTESIAN_POINT ( 'NONE',  ( -35.00000000000000000, -114.0592624029313242, 4.503524454178448266 ) ) ;
#23784=CARTESIAN_POINT ( 'NONE',  ( -34.50000000000000000, -113.0140978167134449, 0.8752176474011410523 ) ) ;
#23789=CARTESIAN_POINT ( 'NONE',  ( -39.16322519054179452, -116.0794154965774823, 2.066024454178448710 ) ) ;
#23802=CARTESIAN_POINT ( 'NONE',  ( -34.50000000000000000, -111.0140821919592327, -0.5779076015960634694 ) ) ;
#23810=CARTESIAN_POINT ( 'NONE',  ( -34.50000000000000000, -113.9929510916434339, 10.50625754673586876 ) ) ;
#23813=CARTESIAN_POINT ( 'NONE',  ( -38.00000000000000711, -113.9929510916434339, 10.50625754673587053 ) ) ;
#23814=CARTESIAN_POINT ( 'NONE',  ( -37.34375000000001421, -115.9929510916434481, 13.11852480586264846 ) ) ;
#23826=CARTESIAN_POINT ( 'NONE',  ( -35.50000000000000711, -112.0269151300720409, -0.7876962586524208776 ) ) ;
#23828=CARTESIAN_POINT ( 'NONE',  ( -35.50000000000000711, -114.2598117360253696, 9.542047897280109936 ) ) ;
#23833=CARTESIAN_POINT ( 'NONE',  ( -34.50000000000000000, -112.0066700803175763, -2.372276521656937920 ) ) ;
#23837=CARTESIAN_POINT ( 'NONE',  ( -39.02454729103295961, -114.7691647218148745, 3.659774454178448710 ) ) ;
#23841=CARTESIAN_POINT ( 'NONE',  ( -35.50000000000000000, -115.0140978167139707, -0.6247823525984387283 ) ) ;
#23842=AXIS2_PLACEMENT_3D ( 'NONE', #30391, #30209, #8406 ) ;
#23849=CARTESIAN_POINT ( 'NONE',  ( -37.43749999999998579, -114.9929510916434339, 13.11852480586264669 ) ) ;
#23852=CARTESIAN_POINT ( 'NONE',  ( -34.50000000000000000, -113.8474311500459777, -1.624782352598427959 ) ) ;
#23853=CARTESIAN_POINT ( 'NONE',  ( -34.50000000000000000, -114.9929510916434339, 12.50851088611648088 ) ) ;
#23858=CARTESIAN_POINT ( 'NONE',  ( -35.93473953453761993, -115.9929510916434481, 13.11451721564123396 ) ) ;
#23872=( BOUNDED_SURFACE ( )  B_SPLINE_SURFACE ( 3, 3, ( 
 ( #6364, #1321, #12125, #17328, #14822, #16976, #23094, #9417, #17698, #28696, #4043, #14991, #25993, #12669, #9780, #1685, #2241, #21101, #21283, #31570, #9956, #15874, #26714, #15517, #26897, #1872, #20917, #4755, #4928, #1499, #32282, #29237, #31740, #12846, #35002, #23649, #20570, #34633, #4581, #15160, #15698, #18230, #2052, #28868, #26537, #23271, #23826, #34270, #34812, #18591, #7073, #7601, #10133, #32104, #10321, #31914, #7249, #20743, #7432, #29591, #9603, #18047, #6896, #18410, #17871, #4220, #23467, #26165, #12485, #13026, #34460, #29044, #24014, #29411, #4392, #15339, #26353, #22169, #16593, #5803, #16047, #10494, #8499, #27066, #16762, #24888, #24182, #18764, #30296, #35530, #32637, #27604, #2940, #7963, #2586, #27244, #18942, #5283, #19474, #24360, #35348, #30114 ),
 ( #29941, #32814, #10857, #16221, #8135, #42, #19115, #13550, #10674, #24538, #27773, #11032, #11197, #21458, #21817, #13206, #13900, #5452, #35177, #27423, #16404, #5634, #30472, #2409, #33168, #2772, #21633, #13735, #213, #24714, #32453, #21994, #32991, #5111, #7779, #8306, #29768, #13377, #19286, #3113, #9021, #20337, #17291, #34053, #11551, #1110, #6322, #14589, #14775, #3463, #14414, #563, #922, #25785, #12079, #22519, #17653, #28120, #14063, #8663, #3286, #9379, #25059, #28470, #31347, #19632, #3816, #25423, #30989, #385, #6674, #23053, #6497, #11384, #5974, #22345, #33339, #16931, #30639, #27936, #14244, #25243, #20161, #738, #33509, #17472, #8837, #19799, #11719, #17114, #30811, #6149, #22691, #33684, #19984, #28296, #3640, #25602, #11903, #22880, #33873, #31168 ),
 ( #9199, #5202, #4177, #31531, #9560, #9912, #9737, #29859, #28657, #4003, #26495, #20528, #14947, #1828, #34231, #12805, #31696, #25953, #23784, #20698, #34421, #1278, #7030, #6855, #12264, #7207, #23238, #29003, #17827, #34770, #10092, #28827, #18189, #29200, #15299, #18861, #15117, #26129, #23601, #1460, #4548, #23424, #18005, #26312, #12441, #1648, #4353, #12626, #15479, #34593, #20875, #31876, #7872, #21059, #32065, #28587, #17762, #28063, #22455, #20451, #3404, #28763, #1222, #507, #30748, #6607, #11831, #8948, #3937, #14884, #19914, #14518, #3571, #30929, #17225, #31464, #672, #11653, #6433, #28231, #17050, #12201, #9137, #25184, #17581, #23174, #25533, #34168, #20274, #848, #4116, #22623, #14351, #25358, #1048, #22810, #11484, #33447, #8768, #25895, #6084, #19735 ),
 ( #33617, #9491, #6261, #33812, #20099, #31106, #14703, #17401, #28404, #3747, #25716, #12020, #22989, #33992, #9318, #31280, #6790, #1394, #32127, #13575, #10698, #26066, #10348, #24209, #7455, #16249, #4779, #12371, #18436, #26739, #15724, #16075, #35561, #13234, #5310, #10519, #10164, #13058, #32305, #18794, #35373, #4951, #21664, #24045, #35030, #29799, #2080, #32474, #18617, #29435, #27268, #35200, #15057, #32669, #2610, #15904, #24566, #7991, #26927, #30140, #21309, #7628, #29615, #27095, #2268, #19143, #23852, #8162, #18973, #21135, #34840, #29971, #21482, #10883, #7807, #5138, #21848, #2433, #13402, #24386, #32844, #11057, #27801, #33194, #25087, #27966, #415, #30498, #27630, #19495, #20013, #3316, #3490, #13759, #3138, #33717, #8867, #33366, #9055, #19657, #14092, #22547 ),
 ( #6003, #25451, #11407, #30842, #22370, #70, #2968, #22193, #8692, #25269, #5830, #592, #13927, #24917, #30669, #8522, #14270, #16788, #11226, #11579, #16962, #240, #33538, #19831, #22025, #6180, #16431, #14442, #17143, #30323, #5660, #28148, #769, #33020, #16618, #11747, #22724, #5478, #27452, #8333, #2800, #24742, #19312, #26175, #1878, #18239, #12680, #12855, #12132, #6543, #4589, #23102, #23833, #20924, #20207, #14830, #26360, #31577, #28706, #23656, #34642, #4054, #34280, #23281, #14997, #1329, #15525, #20382, #9611, #20578, #26000, #12309, #26545, #31394, #6728, #1510, #6908, #1158, #31923, #28875, #9254, #1694, #7259, #17879, #29244, #4403, #4228, #31218, #17704, #34102, #9425, #20750, #15167, #17518, #28521, #3871, #9965, #25836, #12492, #23474, #34469, #9787 ),
 ( #31748, #7080, #18055, #29054, #15348, #26905, #18773, #21643, #29777, #24191, #21291, #13215, #13742, #32646, #32823, #7441, #21465, #27432, #2592, #27074, #2781, #13384, #32461, #16230, #16412, #13033, #8142, #5117, #7607, #24366, #10866, #35184, #32111, #10500, #16056, #26722, #27251, #2416, #13557, #4763, #35354, #34820, #10683, #10142, #7970, #30122, #18599, #19122, #18950, #29950, #21827, #7787, #5290, #32288, #24547, #5460, #21111, #29597, #18418, #35539, #29417, #15705, #35009, #2059, #24023, #10330, #4937, #15884, #2248, #25250, #3647, #5983, #17300, #33694, #28127, #28303, #27612, #22002, #19991, #2950, #24723, #748, #51, #30303, #6157, #11392, #8506, #3471, #14424, #19480, #14071, #30648, #16601, #17122, #19640, #25431, #5641, #16939, #11038, #27945, #6330, #3295 ),
 ( #30482, #5812, #11727, #19293, #14252, #32999, #9031, #16770, #13909, #24895, #25066, #27781, #221, #11204, #11560, #572, #22529, #33518, #22175, #33177, #22701, #8312, #8847, #3118, #19809, #30996, #30819, #394, #22351, #33347, #8674, #17478, #20707, #12634, #9568, #28835, #20537, #23244, #31540, #31707, #6683, #31882, #22887, #34238, #7215, #931, #17664, #9208, #23063, #23611, #1655, #6864, #15125, #9386, #17836, #14785, #25962, #9921, #1467, #1286, #28478, #4185, #18197, #26135, #25794, #3824, #4011, #14954, #14597, #18013, #12447, #20344, #20881, #12271, #20169, #34430, #1116, #34603, #12089, #34060, #25609, #28666, #23433, #31354, #9745, #33880, #7037, #29010, #4359, #15306, #26321, #6503, #11913, #31175, #29208, #2554, #35319, #15485, #34970, #13177, #21067, #5250 ) ),
 .UNSPECIFIED., .T., .F., .F. ) 
 B_SPLINE_SURFACE_WITH_KNOTS ( ( 4, 3, 4 ),
 ( 4, 2, 2, 2, 2, 2, 2, 2, 2, 2, 2, 2, 2, 2, 2, 2, 2, 2, 2, 2, 2, 2, 2, 2, 2, 2, 2, 2, 2, 2, 2, 2, 2, 2, 2, 2, 2, 2, 2, 2, 2, 2, 2, 2, 2, 2, 2, 2, 2, 2, 4 ),
 ( 0.000000000000000000, 0.5000000000000000000, 1.000000000000000000 ),
 ( 0.000000000000000000, 0.05194669433742771930, 0.07792004150614158242, 0.09090671509049851051, 0.09740005188267697456, 0.1038933886748554386, 0.1123700156520060500, 0.1208466426291566476, 0.1377998965834578704, 0.1717064044920602883, 0.2056129124006627062, 0.2225661663549639291, 0.2310427933321145266, 0.2395194203092651519, 0.2482763131408625423, 0.2570332059724599327, 0.2745469916356546580, 0.3095745629620442196, 0.3446021342884337813, 0.3621159199516285621, 0.3708728127832259247, 0.3796297056148233429, 0.3887999023441631730, 0.3979700990735030031, 0.4163104925321826633, 0.4529912794495420392, 0.4896720663669014151, 0.5080124598255810753, 0.5171826565549209054, 0.5263528532842607355, 0.5380287103930572190, 0.5497045675018538136, 0.5730562817194468916, 0.6197597101546329368, 0.6664631385898189819, 0.6898148528074120600, 0.7014907099162086546, 0.7131665670250051381, 0.7223367637543449682, 0.7315069604836847983, 0.7498473539423643475, 0.7865281408597235568, 0.8232089277770826552, 0.8415493212357623154, 0.8507195179651021455, 0.8598897146944418646, 0.8686466075260392827, 0.8774035003576365899, 0.8949172860208314262, 0.9299448573472208768, 1.000000000000000000 ),
 .UNSPECIFIED. ) 
 GEOMETRIC_REPRESENTATION_ITEM ( )  RATIONAL_B_SPLINE_SURFACE ( (
 ( 1.000000000000000000, 1.000000000000000000, 1.000000000000000000, 1.000000000000000000, 1.000000000000000000, 1.000000000000000000, 1.000000000000000000, 1.000000000000000000, 1.000000000000000000, 1.000000000000000000, 1.000000000000000000, 1.000000000000000000, 1.000000000000000000, 1.000000000000000000, 1.000000000000000000, 1.000000000000000000, 1.000000000000000000, 1.000000000000000000, 1.000000000000000000, 1.000000000000000000, 1.000000000000000000, 1.000000000000000000, 1.000000000000000000, 1.000000000000000000, 1.000000000000000000, 1.000000000000000000, 1.000000000000000000, 1.000000000000000000, 1.000000000000000000, 1.000000000000000000, 1.000000000000000000, 1.000000000000000000, 1.000000000000000000, 1.000000000000000000, 1.000000000000000000, 1.000000000000000000, 1.000000000000000000, 1.000000000000000000, 1.000000000000000000, 1.000000000000000000, 1.000000000000000000, 1.000000000000000000, 1.000000000000000000, 1.000000000000000000, 1.000000000000000000, 1.000000000000000000, 1.000000000000000000, 1.000000000000000000, 1.000000000000000000, 1.000000000000000000, 1.000000000000000000, 1.000000000000000000, 1.000000000000000000, 1.000000000000000000, 1.000000000000000000, 1.000000000000000000, 1.000000000000000000, 1.000000000000000000, 1.000000000000000000, 1.000000000000000000, 1.000000000000000000, 1.000000000000000000, 1.000000000000000000, 1.000000000000000000, 1.000000000000000000, 1.000000000000000000, 1.000000000000000000, 1.000000000000000000, 1.000000000000000000, 1.000000000000000000, 1.000000000000000000, 1.000000000000000000, 1.000000000000000000, 1.000000000000000000, 1.000000000000000000, 1.000000000000000000, 1.000000000000000000, 1.000000000000000000, 1.000000000000000000, 1.000000000000000000, 1.000000000000000000, 1.000000000000000000, 1.000000000000000000, 1.000000000000000000, 1.000000000000000000, 1.000000000000000000, 1.000000000000000000, 1.000000000000000000, 1.000000000000000000, 1.000000000000000000, 1.000000000000000000, 1.000000000000000000, 1.000000000000000000, 1.000000000000000000, 1.000000000000000000, 1.000000000000000000, 1.000000000000000000, 1.000000000000000000, 1.000000000000000000, 1.000000000000000000, 1.000000000000000000, 1.000000000000000000),
 ( 0.3333333333333333703, 0.3333333333333333703, 0.3333333333333333703, 0.3333333333333333703, 0.3333333333333333703, 0.3333333333333333703, 0.3333333333333333703, 0.3333333333333333703, 0.3333333333333333703, 0.3333333333333333703, 0.3333333333333333703, 0.3333333333333333703, 0.3333333333333333703, 0.3333333333333333703, 0.3333333333333333703, 0.3333333333333333703, 0.3333333333333333703, 0.3333333333333333703, 0.3333333333333333703, 0.3333333333333333703, 0.3333333333333333703, 0.3333333333333333703, 0.3333333333333333703, 0.3333333333333333703, 0.3333333333333333703, 0.3333333333333333703, 0.3333333333333333703, 0.3333333333333333703, 0.3333333333333333703, 0.3333333333333333703, 0.3333333333333333703, 0.3333333333333333703, 0.3333333333333333703, 0.3333333333333333703, 0.3333333333333333703, 0.3333333333333333703, 0.3333333333333333703, 0.3333333333333333703, 0.3333333333333333703, 0.3333333333333333703, 0.3333333333333333703, 0.3333333333333333703, 0.3333333333333333703, 0.3333333333333333703, 0.3333333333333333703, 0.3333333333333333703, 0.3333333333333333703, 0.3333333333333333703, 0.3333333333333333703, 0.3333333333333333703, 0.3333333333333333703, 0.3333333333333333703, 0.3333333333333333703, 0.3333333333333333703, 0.3333333333333333703, 0.3333333333333333703, 0.3333333333333333703, 0.3333333333333333703, 0.3333333333333333703, 0.3333333333333333703, 0.3333333333333333703, 0.3333333333333333703, 0.3333333333333333703, 0.3333333333333333703, 0.3333333333333333703, 0.3333333333333333703, 0.3333333333333333703, 0.3333333333333333703, 0.3333333333333333703, 0.3333333333333333703, 0.3333333333333333703, 0.3333333333333333703, 0.3333333333333333703, 0.3333333333333333703, 0.3333333333333333703, 0.3333333333333333703, 0.3333333333333333703, 0.3333333333333333703, 0.3333333333333333703, 0.3333333333333333703, 0.3333333333333333703, 0.3333333333333333703, 0.3333333333333333703, 0.3333333333333333703, 0.3333333333333333703, 0.3333333333333333703, 0.3333333333333333703, 0.3333333333333333703, 0.3333333333333333703, 0.3333333333333333703, 0.3333333333333333703, 0.3333333333333333703, 0.3333333333333333703, 0.3333333333333333703, 0.3333333333333333703, 0.3333333333333333703, 0.3333333333333333703, 0.3333333333333333703, 0.3333333333333333703, 0.3333333333333333703, 0.3333333333333333703, 0.3333333333333333703),
 ( 0.3333333333333333703, 0.3333333333333333703, 0.3333333333333333703, 0.3333333333333333703, 0.3333333333333333703, 0.3333333333333333703, 0.3333333333333333703, 0.3333333333333333703, 0.3333333333333333703, 0.3333333333333333703, 0.3333333333333333703, 0.3333333333333333703, 0.3333333333333333703, 0.3333333333333333703, 0.3333333333333333703, 0.3333333333333333703, 0.3333333333333333703, 0.3333333333333333703, 0.3333333333333333703, 0.3333333333333333703, 0.3333333333333333703, 0.3333333333333333703, 0.3333333333333333703, 0.3333333333333333703, 0.3333333333333333703, 0.3333333333333333703, 0.3333333333333333703, 0.3333333333333333703, 0.3333333333333333703, 0.3333333333333333703, 0.3333333333333333703, 0.3333333333333333703, 0.3333333333333333703, 0.3333333333333333703, 0.3333333333333333703, 0.3333333333333333703, 0.3333333333333333703, 0.3333333333333333703, 0.3333333333333333703, 0.3333333333333333703, 0.3333333333333333703, 0.3333333333333333703, 0.3333333333333333703, 0.3333333333333333703, 0.3333333333333333703, 0.3333333333333333703, 0.3333333333333333703, 0.3333333333333333703, 0.3333333333333333703, 0.3333333333333333703, 0.3333333333333333703, 0.3333333333333333703, 0.3333333333333333703, 0.3333333333333333703, 0.3333333333333333703, 0.3333333333333333703, 0.3333333333333333703, 0.3333333333333333703, 0.3333333333333333703, 0.3333333333333333703, 0.3333333333333333703, 0.3333333333333333703, 0.3333333333333333703, 0.3333333333333333703, 0.3333333333333333703, 0.3333333333333333703, 0.3333333333333333703, 0.3333333333333333703, 0.3333333333333333703, 0.3333333333333333703, 0.3333333333333333703, 0.3333333333333333703, 0.3333333333333333703, 0.3333333333333333703, 0.3333333333333333703, 0.3333333333333333703, 0.3333333333333333703, 0.3333333333333333703, 0.3333333333333333703, 0.3333333333333333703, 0.3333333333333333703, 0.3333333333333333703, 0.3333333333333333703, 0.3333333333333333703, 0.3333333333333333703, 0.3333333333333333703, 0.3333333333333333703, 0.3333333333333333703, 0.3333333333333333703, 0.3333333333333333703, 0.3333333333333333703, 0.3333333333333333703, 0.3333333333333333703, 0.3333333333333333703, 0.3333333333333333703, 0.3333333333333333703, 0.3333333333333333703, 0.3333333333333333703, 0.3333333333333333703, 0.3333333333333333703, 0.3333333333333333703, 0.3333333333333333703),
 ( 1.000000000000000000, 1.000000000000000000, 1.000000000000000000, 1.000000000000000000, 1.000000000000000000, 1.000000000000000000, 1.000000000000000000, 1.000000000000000000, 1.000000000000000000, 1.000000000000000000, 1.000000000000000000, 1.000000000000000000, 1.000000000000000000, 1.000000000000000000, 1.000000000000000000, 1.000000000000000000, 1.000000000000000000, 1.000000000000000000, 1.000000000000000000, 1.000000000000000000, 1.000000000000000000, 1.000000000000000000, 1.000000000000000000, 1.000000000000000000, 1.000000000000000000, 1.000000000000000000, 1.000000000000000000, 1.000000000000000000, 1.000000000000000000, 1.000000000000000000, 1.000000000000000000, 1.000000000000000000, 1.000000000000000000, 1.000000000000000000, 1.000000000000000000, 1.000000000000000000, 1.000000000000000000, 1.000000000000000000, 1.000000000000000000, 1.000000000000000000, 1.000000000000000000, 1.000000000000000000, 1.000000000000000000, 1.000000000000000000, 1.000000000000000000, 1.000000000000000000, 1.000000000000000000, 1.000000000000000000, 1.000000000000000000, 1.000000000000000000, 1.000000000000000000, 1.000000000000000000, 1.000000000000000000, 1.000000000000000000, 1.000000000000000000, 1.000000000000000000, 1.000000000000000000, 1.000000000000000000, 1.000000000000000000, 1.000000000000000000, 1.000000000000000000, 1.000000000000000000, 1.000000000000000000, 1.000000000000000000, 1.000000000000000000, 1.000000000000000000, 1.000000000000000000, 1.000000000000000000, 1.000000000000000000, 1.000000000000000000, 1.000000000000000000, 1.000000000000000000, 1.000000000000000000, 1.000000000000000000, 1.000000000000000000, 1.000000000000000000, 1.000000000000000000, 1.000000000000000000, 1.000000000000000000, 1.000000000000000000, 1.000000000000000000, 1.000000000000000000, 1.000000000000000000, 1.000000000000000000, 1.000000000000000000, 1.000000000000000000, 1.000000000000000000, 1.000000000000000000, 1.000000000000000000, 1.000000000000000000, 1.000000000000000000, 1.000000000000000000, 1.000000000000000000, 1.000000000000000000, 1.000000000000000000, 1.000000000000000000, 1.000000000000000000, 1.000000000000000000, 1.000000000000000000, 1.000000000000000000, 1.000000000000000000, 1.000000000000000000),
 ( 0.3333333333333333703, 0.3333333333333333703, 0.3333333333333333703, 0.3333333333333333703, 0.3333333333333333703, 0.3333333333333333703, 0.3333333333333333703, 0.3333333333333333703, 0.3333333333333333703, 0.3333333333333333703, 0.3333333333333333703, 0.3333333333333333703, 0.3333333333333333703, 0.3333333333333333703, 0.3333333333333333703, 0.3333333333333333703, 0.3333333333333333703, 0.3333333333333333703, 0.3333333333333333703, 0.3333333333333333703, 0.3333333333333333703, 0.3333333333333333703, 0.3333333333333333703, 0.3333333333333333703, 0.3333333333333333703, 0.3333333333333333703, 0.3333333333333333703, 0.3333333333333333703, 0.3333333333333333703, 0.3333333333333333703, 0.3333333333333333703, 0.3333333333333333703, 0.3333333333333333703, 0.3333333333333333703, 0.3333333333333333703, 0.3333333333333333703, 0.3333333333333333703, 0.3333333333333333703, 0.3333333333333333703, 0.3333333333333333703, 0.3333333333333333703, 0.3333333333333333703, 0.3333333333333333703, 0.3333333333333333703, 0.3333333333333333703, 0.3333333333333333703, 0.3333333333333333703, 0.3333333333333333703, 0.3333333333333333703, 0.3333333333333333703, 0.3333333333333333703, 0.3333333333333333703, 0.3333333333333333703, 0.3333333333333333703, 0.3333333333333333703, 0.3333333333333333703, 0.3333333333333333703, 0.3333333333333333703, 0.3333333333333333703, 0.3333333333333333703, 0.3333333333333333703, 0.3333333333333333703, 0.3333333333333333703, 0.3333333333333333703, 0.3333333333333333703, 0.3333333333333333703, 0.3333333333333333703, 0.3333333333333333703, 0.3333333333333333703, 0.3333333333333333703, 0.3333333333333333703, 0.3333333333333333703, 0.3333333333333333703, 0.3333333333333333703, 0.3333333333333333703, 0.3333333333333333703, 0.3333333333333333703, 0.3333333333333333703, 0.3333333333333333703, 0.3333333333333333703, 0.3333333333333333703, 0.3333333333333333703, 0.3333333333333333703, 0.3333333333333333703, 0.3333333333333333703, 0.3333333333333333703, 0.3333333333333333703, 0.3333333333333333703, 0.3333333333333333703, 0.3333333333333333703, 0.3333333333333333703, 0.3333333333333333703, 0.3333333333333333703, 0.3333333333333333703, 0.3333333333333333703, 0.3333333333333333703, 0.3333333333333333703, 0.3333333333333333703, 0.3333333333333333703, 0.3333333333333333703, 0.3333333333333333703, 0.3333333333333333703),
 ( 0.3333333333333333703, 0.3333333333333333703, 0.3333333333333333703, 0.3333333333333333703, 0.3333333333333333703, 0.3333333333333333703, 0.3333333333333333703, 0.3333333333333333703, 0.3333333333333333703, 0.3333333333333333703, 0.3333333333333333703, 0.3333333333333333703, 0.3333333333333333703, 0.3333333333333333703, 0.3333333333333333703, 0.3333333333333333703, 0.3333333333333333703, 0.3333333333333333703, 0.3333333333333333703, 0.3333333333333333703, 0.3333333333333333703, 0.3333333333333333703, 0.3333333333333333703, 0.3333333333333333703, 0.3333333333333333703, 0.3333333333333333703, 0.3333333333333333703, 0.3333333333333333703, 0.3333333333333333703, 0.3333333333333333703, 0.3333333333333333703, 0.3333333333333333703, 0.3333333333333333703, 0.3333333333333333703, 0.3333333333333333703, 0.3333333333333333703, 0.3333333333333333703, 0.3333333333333333703, 0.3333333333333333703, 0.3333333333333333703, 0.3333333333333333703, 0.3333333333333333703, 0.3333333333333333703, 0.3333333333333333703, 0.3333333333333333703, 0.3333333333333333703, 0.3333333333333333703, 0.3333333333333333703, 0.3333333333333333703, 0.3333333333333333703, 0.3333333333333333703, 0.3333333333333333703, 0.3333333333333333703, 0.3333333333333333703, 0.3333333333333333703, 0.3333333333333333703, 0.3333333333333333703, 0.3333333333333333703, 0.3333333333333333703, 0.3333333333333333703, 0.3333333333333333703, 0.3333333333333333703, 0.3333333333333333703, 0.3333333333333333703, 0.3333333333333333703, 0.3333333333333333703, 0.3333333333333333703, 0.3333333333333333703, 0.3333333333333333703, 0.3333333333333333703, 0.3333333333333333703, 0.3333333333333333703, 0.3333333333333333703, 0.3333333333333333703, 0.3333333333333333703, 0.3333333333333333703, 0.3333333333333333703, 0.3333333333333333703, 0.3333333333333333703, 0.3333333333333333703, 0.3333333333333333703, 0.3333333333333333703, 0.3333333333333333703, 0.3333333333333333703, 0.3333333333333333703, 0.3333333333333333703, 0.3333333333333333703, 0.3333333333333333703, 0.3333333333333333703, 0.3333333333333333703, 0.3333333333333333703, 0.3333333333333333703, 0.3333333333333333703, 0.3333333333333333703, 0.3333333333333333703, 0.3333333333333333703, 0.3333333333333333703, 0.3333333333333333703, 0.3333333333333333703, 0.3333333333333333703, 0.3333333333333333703, 0.3333333333333333703),
 ( 1.000000000000000000, 1.000000000000000000, 1.000000000000000000, 1.000000000000000000, 1.000000000000000000, 1.000000000000000000, 1.000000000000000000, 1.000000000000000000, 1.000000000000000000, 1.000000000000000000, 1.000000000000000000, 1.000000000000000000, 1.000000000000000000, 1.000000000000000000, 1.000000000000000000, 1.000000000000000000, 1.000000000000000000, 1.000000000000000000, 1.000000000000000000, 1.000000000000000000, 1.000000000000000000, 1.000000000000000000, 1.000000000000000000, 1.000000000000000000, 1.000000000000000000, 1.000000000000000000, 1.000000000000000000, 1.000000000000000000, 1.000000000000000000, 1.000000000000000000, 1.000000000000000000, 1.000000000000000000, 1.000000000000000000, 1.000000000000000000, 1.000000000000000000, 1.000000000000000000, 1.000000000000000000, 1.000000000000000000, 1.000000000000000000, 1.000000000000000000, 1.000000000000000000, 1.000000000000000000, 1.000000000000000000, 1.000000000000000000, 1.000000000000000000, 1.000000000000000000, 1.000000000000000000, 1.000000000000000000, 1.000000000000000000, 1.000000000000000000, 1.000000000000000000, 1.000000000000000000, 1.000000000000000000, 1.000000000000000000, 1.000000000000000000, 1.000000000000000000, 1.000000000000000000, 1.000000000000000000, 1.000000000000000000, 1.000000000000000000, 1.000000000000000000, 1.000000000000000000, 1.000000000000000000, 1.000000000000000000, 1.000000000000000000, 1.000000000000000000, 1.000000000000000000, 1.000000000000000000, 1.000000000000000000, 1.000000000000000000, 1.000000000000000000, 1.000000000000000000, 1.000000000000000000, 1.000000000000000000, 1.000000000000000000, 1.000000000000000000, 1.000000000000000000, 1.000000000000000000, 1.000000000000000000, 1.000000000000000000, 1.000000000000000000, 1.000000000000000000, 1.000000000000000000, 1.000000000000000000, 1.000000000000000000, 1.000000000000000000, 1.000000000000000000, 1.000000000000000000, 1.000000000000000000, 1.000000000000000000, 1.000000000000000000, 1.000000000000000000, 1.000000000000000000, 1.000000000000000000, 1.000000000000000000, 1.000000000000000000, 1.000000000000000000, 1.000000000000000000, 1.000000000000000000, 1.000000000000000000, 1.000000000000000000, 1.000000000000000000) ) ) 
 REPRESENTATION_ITEM ( '' )  SURFACE ( )  );
#23873=CARTESIAN_POINT ( 'NONE',  ( -35.99999999999999289, -114.0592624029313242, 6.003524454178450043 ) ) ;
#23883=CARTESIAN_POINT ( 'NONE',  ( -38.45611840935523418, -112.6276912846090568, 3.433975545821551290 ) ) ;
#23890=EDGE_CURVE ( 'NONE', #17346, #18651, #202, .T. ) ;
#23903=CARTESIAN_POINT ( 'NONE',  ( -34.68937937320795584, -115.9929510916434481, 13.37409560816408671 ) ) ;
#23905=CARTESIAN_POINT ( 'NONE',  ( -38.97545270896704039, -113.1123104723225055, 8.347274454178448266 ) ) ;
#23906=CARTESIAN_POINT ( 'NONE',  ( -34.50000000000000000, -115.9929081983957104, 10.49113315946066294 ) ) ;
#23915=CARTESIAN_POINT ( 'NONE',  ( -34.97545270896703329, -114.7691647218148745, 5.590225545821552622 ) ) ;
#23937=CARTESIAN_POINT ( 'NONE',  ( -35.50000000000000711, -112.9876085932806262, 1.879154677457530065 ) ) ;
#23938=EDGE_CURVE ( 'NONE', #31629, #24733, #3684, .T. ) ;
#23944=CARTESIAN_POINT ( 'NONE',  ( -34.50000000000000000, -114.9929510916434339, 12.17846912687782712 ) ) ;
#23947=CARTESIAN_POINT ( 'NONE',  ( -37.75185693410092824, -114.9929510916434339, 13.05539834812634581 ) ) ;
#23950=CARTESIAN_POINT ( 'NONE',  ( -34.50000000000000000, -114.9819937217110635, 10.35556074009299188 ) ) ;
#23954=CARTESIAN_POINT ( 'NONE',  ( -37.52044295795950291, -114.9929510916434339, 13.11812344617477244 ) ) ;
#23960=CARTESIAN_POINT ( 'NONE',  ( -37.99974912065192711, -114.9929510916434339, 12.63488142334838571 ) ) ;
#23962=CARTESIAN_POINT ( 'NONE',  ( -35.02454729103298803, -114.8876895276775087, 7.597274454178450931 ) ) ;
#23970=CARTESIAN_POINT ( 'NONE',  ( -37.05926240293131713, -115.9999999999999858, 7.878524454178450043 ) ) ;
#23982=CARTESIAN_POINT ( 'NONE',  ( -34.50000000000000000, -111.3577635893106361, 2.022004269840791402 ) ) ;
#23991=CARTESIAN_POINT ( 'NONE',  ( -35.50000000000000711, -114.1189822439768449, 9.514224058074130852 ) ) ;
#23993=CARTESIAN_POINT ( 'NONE',  ( -34.50000000000000000, -113.9929510916438460, 10.50625754673626133 ) ) ;
#23997=CARTESIAN_POINT ( 'NONE',  ( -34.50000000000000000, -113.9836614335179377, 10.50514867547815534 ) ) ;
#23999=CARTESIAN_POINT ( 'NONE',  ( -36.15625000000007816, -115.9929510916434481, 13.11852480586264846 ) ) ;
#24014=CARTESIAN_POINT ( 'NONE',  ( -35.50000000000000711, -114.8474311500471572, -1.624782352598427959 ) ) ;
#24018=CARTESIAN_POINT ( 'NONE',  ( -35.50000000000000711, -114.9656200615856818, 10.26631071845107179 ) ) ;
#24023=CARTESIAN_POINT ( 'NONE',  ( -35.50000000000000000, -113.4307644833805142, -2.624782352598442614 ) ) ;
#24026=CARTESIAN_POINT ( 'NONE',  ( -36.64504884055823908, -115.0245472910329880, 6.284774454178449155 ) ) ;
#24031=CARTESIAN_POINT ( 'NONE',  ( -34.50000000000000000, -113.0140978167138712, -0.1247823525984260717 ) ) ;
#24040=CARTESIAN_POINT ( 'NONE',  ( -37.34375000000001421, -114.9929510916434339, 13.11852480586264669 ) ) ;
#24045=CARTESIAN_POINT ( 'NONE',  ( -34.50000000000000000, -112.0141059978162019, -0.6575071456984691309 ) ) ;
#24051=CARTESIAN_POINT ( 'NONE',  ( -37.37500000000009237, -115.9929510916434481, 13.11852480586264846 ) ) ;
#24052=CARTESIAN_POINT ( 'NONE',  ( -35.50000000000000711, -112.9486715495423681, -1.623175561345890472 ) ) ;
#24062=CARTESIAN_POINT ( 'NONE',  ( -37.47347596530441649, -114.9754527089670262, 7.972274454178450043 ) ) ;
#24066=ORIENTED_EDGE ( 'NONE', *, *, #8362, .F. ) ;
#24074=CARTESIAN_POINT ( 'NONE',  ( -38.99999999999999289, -114.0592624029313242, 7.746475545821551734 ) ) ;
#24093=DIRECTION ( 'NONE',  ( -1.000000000000000000, 0.000000000000000000, 0.000000000000000000 ) ) ;
#24094=CARTESIAN_POINT ( 'NONE',  ( -36.94073759706868287, -112.0000000000000142, 7.128524454178449155 ) ) ;
#24095=CARTESIAN_POINT ( 'NONE',  ( -34.50481333282507279, -115.9929510916434481, 12.74107470552716315 ) ) ;
#24103=CARTESIAN_POINT ( 'NONE',  ( -39.97545270896702618, -115.3019030900506152, 9.152725545821551734 ) ) ;
#24120=CARTESIAN_POINT ( 'NONE',  ( -35.50000000000000711, -113.0796441757086939, 1.890140615870383956 ) ) ;
#24125=CARTESIAN_POINT ( 'NONE',  ( -34.50000000000000000, -112.9876085932806262, 1.879154677457530065 ) ) ;
#24126=CARTESIAN_POINT ( 'NONE',  ( -34.50000000000000000, -114.5636144531578680, 9.676196722963288366 ) ) ;
#24128=CARTESIAN_POINT ( 'NONE',  ( -35.99386409314529800, -114.9929510916434339, 13.11852378322482515 ) ) ;
#24130=CARTESIAN_POINT ( 'NONE',  ( -34.50000000000000000, -114.9929517792218689, 10.50900788599415314 ) ) ;
#24138=CARTESIAN_POINT ( 'NONE',  ( -37.56526046546250086, -114.9929510916434339, 13.11451721564129258 ) ) ;
#24141=CARTESIAN_POINT ( 'NONE',  ( -39.07941549657748936, -111.8367748094582055, 2.441024454178448710 ) ) ;
#24148=CARTESIAN_POINT ( 'NONE',  ( -37.05926240293133134, -116.9999999999999858, 4.878524454178448266 ) ) ;
#24159=CARTESIAN_POINT ( 'NONE',  ( -34.50000000000000000, -111.0140978167138570, 0.7502176474015694874 ) ) ;
#24164=CARTESIAN_POINT ( 'NONE',  ( -35.50000000000000711, -114.1414532730574507, 9.517316564499758158 ) ) ;
#24165=CARTESIAN_POINT ( 'NONE',  ( -34.50000000000000000, -113.9465028010160381, 10.50071319044726081 ) ) ;
#24168=CARTESIAN_POINT ( 'NONE',  ( -37.98402046630260287, -113.9929510916434339, 12.74811950270164296 ) ) ;
#24169=CARTESIAN_POINT ( 'NONE',  ( -37.49414064056232831, -115.9929510916434481, 13.11852578240983291 ) ) ;
#24182=CARTESIAN_POINT ( 'NONE',  ( -35.50000000000000711, -115.9821387493194891, -0.8839717462762166633 ) ) ;
#24187=CARTESIAN_POINT ( 'NONE',  ( -35.50000000000000711, -114.9929510916434339, 10.72628538622835670 ) ) ;
#24191=CARTESIAN_POINT ( 'NONE',  ( -35.50000000000000000, -112.8230659962028994, 2.866612799894348029 ) ) ;
#24194=CARTESIAN_POINT ( 'NONE',  ( -36.25098837183129774, -113.3347980657956242, 7.316024454178450043 ) ) ;
#24200=CARTESIAN_POINT ( 'NONE',  ( -34.50000000000000000, -113.0140978167138712, -0.5622823525984297355 ) ) ;
#24204=CARTESIAN_POINT ( 'NONE',  ( -38.00000000000000711, -114.9929510916434339, 11.91443571948719615 ) ) ;
#24209=CARTESIAN_POINT ( 'NONE',  ( -34.50000000000000000, -112.0250551866464548, 1.025914454044489332 ) ) ;
#24216=CARTESIAN_POINT ( 'NONE',  ( -35.50000000000000711, -114.1068310684433129, 9.512752019463897923 ) ) ;
#24238=CARTESIAN_POINT ( 'NONE',  ( -37.88768952767750875, -112.0245472910329880, 8.027725545821549957 ) ) ;
#24258=PRODUCT_DEFINITION ( 'UNKNOWN', '', #15498, #17678 ) ;
#24259=CARTESIAN_POINT ( 'NONE',  ( -36.23083527818513261, -116.0245472910329880, 6.284774454178449155 ) ) ;
#24263=CARTESIAN_POINT ( 'NONE',  ( -34.50000000000000000, -115.9792481177720731, 10.26484292309424795 ) ) ;
#24274=CARTESIAN_POINT ( 'NONE',  ( -35.69809690994941320, -116.9754527089670546, 8.777725545821549957 ) ) ;
#24286=CARTESIAN_POINT ( 'NONE',  ( -38.45611840935523418, -112.6276912846090568, 9.433975545821551734 ) ) ;
#24293=CARTESIAN_POINT ( 'NONE',  ( -35.50000000000000711, -112.3995503592287690, -1.424448457485529618 ) ) ;
#24299=CARTESIAN_POINT ( 'NONE',  ( -34.50000000000000000, -112.0140978167138712, -0.4997823525984337878 ) ) ;
#24301=CARTESIAN_POINT ( 'NONE',  ( -35.98977351030467986, -114.9929510916434339, 14.11852173794918386 ) ) ;
#24304=CARTESIAN_POINT ( 'NONE',  ( -35.50000000000000000, -113.9813390189866027, 10.50487145766371100 ) ) ;
#24306=CARTESIAN_POINT ( 'NONE',  ( -34.50000000000000000, -114.0998638248492085, 9.511920366020609308 ) ) ;
#24308=CARTESIAN_POINT ( 'NONE',  ( -38.00000000000000711, -114.9929510916434339, 12.53051367006571937 ) ) ;
#24313=CARTESIAN_POINT ( 'NONE',  ( -37.37500000000009237, -114.9929510916434339, 13.11852480586264669 ) ) ;
#24317=CARTESIAN_POINT ( 'NONE',  ( -35.62769128460905677, -115.4561184093552413, 6.191024454178448266 ) ) ;
#24325=CARTESIAN_POINT ( 'NONE',  ( -34.97545270896703329, -113.2308352781851539, 8.909774454178450043 ) ) ;
#24337=CARTESIAN_POINT ( 'NONE',  ( -34.50000000000000000, -111.0140821919084715, 0.8283428459075261596 ) ) ;
#24341=CARTESIAN_POINT ( 'NONE',  ( -35.50000000000000711, -114.1712995509219724, 9.522174004479579068 ) ) ;
#24343=CARTESIAN_POINT ( 'NONE',  ( -34.50000000000000000, -113.9929510916434339, 10.50625754673609258 ) ) ;
#24346=CARTESIAN_POINT ( 'NONE',  ( -37.80727372874345349, -113.9929510916434339, 13.01835785830664705 ) ) ;
#24347=CARTESIAN_POINT ( 'NONE',  ( -38.00000000000000711, -115.9929510916434481, 12.60752341388803721 ) ) ;
#24360=CARTESIAN_POINT ( 'NONE',  ( -35.50000000000000711, -116.0140978167138712, 0.3752176474015736507 ) ) ;
#24362=CARTESIAN_POINT ( 'NONE',  ( -35.50000000000000711, -114.9929510916434339, 10.68227981832981044 ) ) ;
#24366=CARTESIAN_POINT ( 'NONE',  ( -35.50000000000000000, -111.0140978167138570, 0.7502176474015694874 ) ) ;
#24369=CARTESIAN_POINT ( 'NONE',  ( -34.97545270896703329, -113.2308352781851539, 2.909774454178448710 ) ) ;
#24375=CARTESIAN_POINT ( 'NONE',  ( -34.50000000000000000, -113.0140978167138712, -0.3122823525984338988 ) ) ;
#24382=CARTESIAN_POINT ( 'NONE',  ( -37.54084996655477369, -114.9929510916434339, 13.11692036158760466 ) ) ;
#24386=CARTESIAN_POINT ( 'NONE',  ( -34.50000000000000000, -115.2732872103912030, -1.592823285204062911 ) ) ;
#24392=CARTESIAN_POINT ( 'NONE',  ( -37.51635661748575501, -115.9929510916434481, 13.11827392651459512 ) ) ;
#24413=CARTESIAN_POINT ( 'NONE',  ( -35.54388159064475872, -115.3723087153909432, 5.683975545821551734 ) ) ;
#24431=CARTESIAN_POINT ( 'NONE',  ( -39.02454729103295961, -114.7691647218148745, 6.659774454178449155 ) ) ;
#24433=CARTESIAN_POINT ( 'NONE',  ( -37.54906985245723661, -115.9929510916434481, 14.11777216781844757 ) ) ;
#24443=CARTESIAN_POINT ( 'NONE',  ( -39.02454729103295961, -113.2308352781851539, 3.340225545821550845 ) ) ;
#24463=CARTESIAN_POINT ( 'NONE',  ( -35.50000000000000711, -112.9486715495423681, -1.623175561345890472 ) ) ;
#24473=CARTESIAN_POINT ( 'NONE',  ( -34.50000000000000000, -115.2732872103912030, -1.592823285204062911 ) ) ;
#24474=CARTESIAN_POINT ( 'NONE',  ( -38.95206139890800046, -114.9929510916434339, 13.00730889637963728 ) ) ;
#24476=CARTESIAN_POINT ( 'NONE',  ( -35.50000000000000000, -113.9557924591415627, 10.50182206170499555 ) ) ;
#24478=CARTESIAN_POINT ( 'NONE',  ( -35.97545865737298953, -114.9929510916434339, 14.11837420659365705 ) ) ;
#24487=CARTESIAN_POINT ( 'NONE',  ( -37.52044295795950291, -114.9929510916434339, 13.11812344617477244 ) ) ;
#24489=CARTESIAN_POINT ( 'NONE',  ( -36.11231047232249125, -112.0245472910329880, 8.722274454178448266 ) ) ;
#24498=CARTESIAN_POINT ( 'NONE',  ( -38.30190309005061522, -111.0245472910330022, 3.527725545821551734 ) ) ;
#24510=CARTESIAN_POINT ( 'NONE',  ( -34.50000000000000000, -111.7850029017436810, -2.224114562373086912 ) ) ;
#24517=CARTESIAN_POINT ( 'NONE',  ( -35.50000000000000711, -114.8211182053456838, 9.932864235516914775 ) ) ;
#24521=CARTESIAN_POINT ( 'NONE',  ( -34.50300906734826611, -113.9929510916434339, 12.71660600561482468 ) ) ;
#24524=CARTESIAN_POINT ( 'NONE',  ( -37.99359134332094357, -113.9929510916434339, 12.69998175888958514 ) ) ;
#24526=CARTESIAN_POINT ( 'NONE',  ( -35.50000000000000711, -114.1489256397697289, 9.518467544735724317 ) ) ;
#24538=CARTESIAN_POINT ( 'NONE',  ( -35.50000000000000000, -113.0601156079281253, 0.8807106166081309917 ) ) ;
#24540=CARTESIAN_POINT ( 'NONE',  ( -35.50000000000000711, -114.9929510916434339, 12.50851088611648088 ) ) ;
#24547=CARTESIAN_POINT ( 'NONE',  ( -35.50000000000000000, -112.4957190293567066, -2.560864217808777266 ) ) ;
#24551=CARTESIAN_POINT ( 'NONE',  ( -37.05926240293133134, -115.0000000000000000, 6.378524454178448266 ) ) ;
#24557=CARTESIAN_POINT ( 'NONE',  ( -34.50000000000000000, -115.0304602784513293, -0.6247823525985405357 ) ) ;
#24563=CARTESIAN_POINT ( 'NONE',  ( -35.50000000000000000, -113.9929510916434339, 12.59102132592610346 ) ) ;
#24566=CARTESIAN_POINT ( 'NONE',  ( -34.50000000000000000, -112.8835768857893527, -1.616767172155725740 ) ) ;
#24568=CARTESIAN_POINT ( 'NONE',  ( -37.34375000000001421, -115.9929510916434481, 14.11852480586265024 ) ) ;
#24575=CARTESIAN_POINT ( 'NONE',  ( -35.50000000000000711, -114.1302255537607095, 9.515717283514957714 ) ) ;
#24597=CARTESIAN_POINT ( 'NONE',  ( -36.11231047232249125, -115.9754527089670262, 8.777725545821555286 ) ) ;
#24615=CARTESIAN_POINT ( 'NONE',  ( -38.99699093265172678, -115.9929510916434481, 12.71660600561481402 ) ) ;
#24624=CARTESIAN_POINT ( 'NONE',  ( -37.97545270896702618, -114.4734759653044023, 3.152725545821551734 ) ) ;
#24630=ORIENTED_EDGE ( 'NONE', *, *, #17320, .T. ) ;
#24650=CARTESIAN_POINT ( 'NONE',  ( -34.50000000000000000, -112.9813730236132585, -1.624774171495860786 ) ) ;
#24651=CARTESIAN_POINT ( 'NONE',  ( -38.99879592093640923, -114.9929510916434339, 12.67985367974111455 ) ) ;
#24652=CARTESIAN_POINT ( 'NONE',  ( -38.00000000000000711, -114.9929510916434339, 11.21034663311206181 ) ) ;
#24654=CARTESIAN_POINT ( 'NONE',  ( -34.54793860109200665, -114.9929510916434339, 13.00730889637958221 ) ) ;
#24665=CARTESIAN_POINT ( 'NONE',  ( -39.07941549657748936, -111.8367748094582055, 8.441024454178448266 ) ) ;
#24676=CARTESIAN_POINT ( 'NONE',  ( -34.02454729103297382, -112.6980969099494132, 3.902725545821552178 ) ) ;
#24688=CARTESIAN_POINT ( 'NONE',  ( -34.50000000000000000, -117.0108842342086888, -0.7556348869410856040 ) ) ;
#24692=CARTESIAN_POINT ( 'NONE',  ( -35.50000000000000711, -114.9929510916434339, 10.61627146648203812 ) ) ;
#24694=CARTESIAN_POINT ( 'NONE',  ( -37.42187499999996447, -113.9929510916434339, 14.11852480586265024 ) ) ;
#24698=CARTESIAN_POINT ( 'NONE',  ( -34.50000000000000000, -113.9929510916435049, 10.50625754673586876 ) ) ;
#24702=CARTESIAN_POINT ( 'NONE',  ( -35.50000000000000711, -114.5636144531578680, 9.676196722963288366 ) ) ;
#24714=CARTESIAN_POINT ( 'NONE',  ( -35.50000000000000000, -113.0140978167138712, 0.7502176474015694874 ) ) ;
#24716=CARTESIAN_POINT ( 'NONE',  ( -36.94073759706866156, -113.0000000000000000, 4.128524454178449155 ) ) ;
#24723=CARTESIAN_POINT ( 'NONE',  ( -35.50000000000000000, -115.6584342456100671, -2.522673865603758614 ) ) ;
#24726=CARTESIAN_POINT ( 'NONE',  ( -37.05926240293131713, -115.9999999999999858, 7.878524454178450043 ) ) ;
#24733=VERTEX_POINT ( 'NONE', #6844 ) ;
#24734=CARTESIAN_POINT ( 'NONE',  ( -34.50000000000000000, -113.0140978167138712, 0.6252176474015680441 ) ) ;
#24738=CARTESIAN_POINT ( 'NONE',  ( -35.50100302244945993, -113.9929510916434339, 12.65121853911337446 ) ) ;
#24742=CARTESIAN_POINT ( 'NONE',  ( -34.50000000000000000, -111.0140978167138570, -0.5622823525984297355 ) ) ;
#24744=CARTESIAN_POINT ( 'NONE',  ( -38.99999693208653895, -115.9929510916434481, 12.62875129555797749 ) ) ;
#24750=CIRCLE ( 'NONE', #20711, 0.5000000000000004441 ) ;
#24751=CARTESIAN_POINT ( 'NONE',  ( -38.00000000000000711, -115.9929510916434481, 11.73841344789285657 ) ) ;
#24771=CARTESIAN_POINT ( 'NONE',  ( -37.05926240293131713, -112.0000000000000142, 8.121475545821549957 ) ) ;
#24791=CARTESIAN_POINT ( 'NONE',  ( -35.97545865737298953, -115.9929510916434481, 14.11837420659365527 ) ) ;
#24800=CARTESIAN_POINT ( 'NONE',  ( -37.97545270896702618, -114.4734759653044023, 4.652725545821551734 ) ) ;
#24825=CARTESIAN_POINT ( 'NONE',  ( -34.50000000000000000, -113.2224311500466030, -1.624782352598427959 ) ) ;
#24827=CARTESIAN_POINT ( 'NONE',  ( -37.56132887387857267, -114.9929510916434339, 14.11732072679899197 ) ) ;
#24828=CARTESIAN_POINT ( 'NONE',  ( -35.50000000000000000, -113.9929510916433344, 10.50625754673586876 ) ) ;
#24830=CARTESIAN_POINT ( 'NONE',  ( -34.50000000000000000, -114.9929510916434339, 12.17846912687782712 ) ) ;
#24841=CARTESIAN_POINT ( 'NONE',  ( -38.18337828418795965, -110.9754527089670546, 4.034774454178449155 ) ) ;
#24849=CARTESIAN_POINT ( 'NONE',  ( -40.02454729103296671, -112.8166217158120332, 4.840225545821551734 ) ) ;
#24851=DIRECTION ( 'NONE',  ( 0.000000000000000000, 0.000000000000000000, -1.000000000000000000 ) ) ;
#24861=CARTESIAN_POINT ( 'NONE',  ( -34.50000000000000000, -117.0140978167138854, 0.3752176474015737617 ) ) ;
#24864=CARTESIAN_POINT ( 'NONE',  ( -35.49999931242378892, -114.9929510916434339, 12.61439929482945566 ) ) ;
#24866=CARTESIAN_POINT ( 'NONE',  ( -35.95093014754292682, -113.9929510916434339, 14.11777216781842625 ) ) ;
#24873=CARTESIAN_POINT ( 'NONE',  ( -34.50000000000000000, -113.9929510916433912, 10.50625754673588474 ) ) ;
#24874=CARTESIAN_POINT ( 'NONE',  ( -38.99984940073101569, -114.9929510916434339, 12.64306614848957189 ) ) ;
#24875=CARTESIAN_POINT ( 'NONE',  ( -35.50000000000000711, -114.0928965812550757, 9.511088712577292270 ) ) ;
#24888=CARTESIAN_POINT ( 'NONE',  ( -35.50000000000000711, -115.9630435732166518, -0.9469505670456015434 ) ) ;
#24890=CARTESIAN_POINT ( 'NONE',  ( -36.52652403469556930, -113.0245472910329880, 8.722274454178450043 ) ) ;
#24895=CARTESIAN_POINT ( 'NONE',  ( -35.50000000000000711, -112.9415908020655195, 1.873661708251232572 ) ) ;
#24899=CARTESIAN_POINT ( 'NONE',  ( -38.97545270896704039, -113.1123104723225197, 6.847274454178450931 ) ) ;
#24904=CARTESIAN_POINT ( 'NONE',  ( -34.50000000000000000, -115.0140978167138712, -0.3122823525984416704 ) ) ;
#24912=CARTESIAN_POINT ( 'NONE',  ( -35.50000000000000000, -113.9929510916434339, 10.68227981832981044 ) ) ;
#24917=CARTESIAN_POINT ( 'NONE',  ( -34.50000000000000000, -112.5389594332240222, 2.818899826424027477 ) ) ;
#24918=CARTESIAN_POINT ( 'NONE',  ( -35.50000000000000000, -114.2253558743059330, 8.519800927820798009 ) ) ;
#24924=CARTESIAN_POINT ( 'NONE',  ( -37.58145695302688694, -115.9929510916434481, 13.11211614918362756 ) ) ;
#24944=CARTESIAN_POINT ( 'NONE',  ( -35.62769128460905677, -112.5438815906447729, 9.808975545821551734 ) ) ;
#24964=CARTESIAN_POINT ( 'NONE',  ( -37.51022648969539119, -115.9929510916434481, 14.11852173794918563 ) ) ;
#24974=CARTESIAN_POINT ( 'NONE',  ( -37.76916472181486739, -116.0245472910329880, 8.965225545821551734 ) ) ;
#24999=CARTESIAN_POINT ( 'NONE',  ( -34.50000000000000000, -112.5103839485166333, -1.498529437127682495 ) ) ;
#25000=CARTESIAN_POINT ( 'NONE',  ( -39.00000000000000711, -114.9929510916434339, 12.59102132592608925 ) ) ;
#25001=CARTESIAN_POINT ( 'NONE',  ( -35.50000000000000000, -113.9929510916434339, 10.50625754673588474 ) ) ;
#25003=CARTESIAN_POINT ( 'NONE',  ( -35.61121590948313553, -114.9929510916434339, 14.07058620477040733 ) ) ;
#25014=CARTESIAN_POINT ( 'NONE',  ( -39.99999999999999289, -113.9407375970686758, 3.753524454178448710 ) ) ;
#25016=CARTESIAN_POINT ( 'NONE',  ( -35.50000000000000711, -113.6807644833805995, -1.624782352598427959 ) ) ;
#25037=CARTESIAN_POINT ( 'NONE',  ( -34.50000000000000000, -117.0140978167138854, -0.3747823525984421145 ) ) ;
#25040=CARTESIAN_POINT ( 'NONE',  ( -35.50000000000000711, -114.9929510916434339, 12.56351784598954424 ) ) ;
#25041=CARTESIAN_POINT ( 'NONE',  ( -36.50000000000010658, -113.9929510916434339, 14.11852480586265024 ) ) ;
#25045=CARTESIAN_POINT ( 'NONE',  ( -34.50000000000000000, -113.9929510916434339, 10.55026311463432087 ) ) ;
#25046=CARTESIAN_POINT ( 'NONE',  ( -39.00000000000000711, -114.9929510916434339, 12.44250253426874941 ) ) ;
#25048=CARTESIAN_POINT ( 'NONE',  ( -35.50000000000000711, -114.9929501463477663, 10.50247632894551231 ) ) ;
#25059=CARTESIAN_POINT ( 'NONE',  ( -35.50000000000000000, -113.2224311500466030, -0.6247823525984269599 ) ) ;
#25061=CARTESIAN_POINT ( 'NONE',  ( -35.00000000000000000, -114.0592624029313242, 4.503524454178448266 ) ) ;
#25066=CARTESIAN_POINT ( 'NONE',  ( -35.50000000000000711, -112.9185811467682754, 1.870920967077121411 ) ) ;
#25070=CARTESIAN_POINT ( 'NONE',  ( -37.88768952767750164, -115.9754527089670262, 7.972274454178450043 ) ) ;
#25075=CARTESIAN_POINT ( 'NONE',  ( -34.50000000000000000, -112.0209493036498287, 0.9959249592223760050 ) ) ;
#25084=CARTESIAN_POINT ( 'NONE',  ( -35.50000000000000000, -113.9929510916434339, 10.50625754673588474 ) ) ;
#25087=CARTESIAN_POINT ( 'NONE',  ( -34.50000000000000000, -115.8878449012421754, -1.128496220799388494 ) ) ;
#25088=CARTESIAN_POINT ( 'NONE',  ( -39.00000000000000000, -115.9929510916434481, 12.44250253426875119 ) ) ;
#25117=CARTESIAN_POINT ( 'NONE',  ( -37.35495115944176803, -115.0245472910329880, 2.965225545821551734 ) ) ;
#25128=CARTESIAN_POINT ( 'NONE',  ( -35.50000000000000711, -113.8474311500459777, -1.624782352598427959 ) ) ;
#25137=CARTESIAN_POINT ( 'NONE',  ( -34.50000000000000000, -114.0743172650041686, 9.508870970061893857 ) ) ;
#25141=CARTESIAN_POINT ( 'NONE',  ( -37.48437500000004263, -115.9929510916434481, 14.11852480586265024 ) ) ;
#25154=CARTESIAN_POINT ( 'NONE',  ( -37.35495115944176803, -115.0245472910329880, 2.965225545821551734 ) ) ;
#25167=EDGE_LOOP ( 'NONE', ( #17963, #30612, #21538, #24630, #15708 ) ) ;
#25184=CARTESIAN_POINT ( 'NONE',  ( -34.50000000000000000, -115.0140978167134165, -0.6247823525984399495 ) ) ;
#25188=CARTESIAN_POINT ( 'NONE',  ( -34.50000000000000000, -115.9929510916434481, 10.51175824272318415 ) ) ;
#25191=CARTESIAN_POINT ( 'NONE',  ( -35.98977351030467986, -114.9929510916434339, 14.11852173794918386 ) ) ;
#25202=CARTESIAN_POINT ( 'NONE',  ( -36.94073759706866156, -111.0000000000000284, 2.628524454178448710 ) ) ;
#25204=CARTESIAN_POINT ( 'NONE',  ( -35.50000000000000711, -112.0140978167138712, -0.4685323525984295134 ) ) ;
#25222=CARTESIAN_POINT ( 'NONE',  ( -35.50000000000000000, -113.2372261171341563, 2.916049522752222511 ) ) ;
#25224=CARTESIAN_POINT ( 'NONE',  ( -35.50100302244946704, -114.9929510916434339, 12.65121853911337269 ) ) ;
#25225=CARTESIAN_POINT ( 'NONE',  ( -34.50000000000000000, -113.9929510916434339, 11.91443571948720148 ) ) ;
#25228=CARTESIAN_POINT ( 'NONE',  ( -34.50000000000000000, -113.9929510916434339, 12.53051367006571581 ) ) ;
#25231=CARTESIAN_POINT ( 'NONE',  ( -35.50000000000000711, -114.9902084924877954, 10.43071793783961176 ) ) ;
#25243=CARTESIAN_POINT ( 'NONE',  ( -35.50000000000000000, -115.0140978167138428, -0.6247823525979866455 ) ) ;
#25245=CARTESIAN_POINT ( 'NONE',  ( -37.35495115944176092, -112.9754527089670688, 8.534774454178448266 ) ) ;
#25250=CARTESIAN_POINT ( 'NONE',  ( -35.50000000000000000, -114.5974311500472567, -2.624782352598442614 ) ) ;
#25260=CARTESIAN_POINT ( 'NONE',  ( -34.50000000000000000, -112.0141059978162019, -0.6575071456984691309 ) ) ;
#25266=CARTESIAN_POINT ( 'NONE',  ( -35.50000000000000000, -113.9929510916434339, 10.50625754673586876 ) ) ;
#25269=CARTESIAN_POINT ( 'NONE',  ( -34.50000000000000000, -112.8230659962028994, 2.866612799894348029 ) ) ;
#25270=CARTESIAN_POINT ( 'NONE',  ( -35.50000000000000000, -114.5266723804073195, 8.577838247824468354 ) ) ;
#25296=CARTESIAN_POINT ( 'NONE',  ( -36.25098837183130485, -114.6652019342044184, 5.683975545821551734 ) ) ;
#25302=CARTESIAN_POINT ( 'NONE',  ( -35.50000000000000711, -114.8057644833805568, -1.624782352598427959 ) ) ;
#25306=CARTESIAN_POINT ( 'NONE',  ( -35.50000000000000711, -114.9927795562974069, 10.48735431211914815 ) ) ;
#25312=CARTESIAN_POINT ( 'NONE',  ( -34.50000000000000000, -114.9929510916434339, 10.51175824272318415 ) ) ;
#25319=CARTESIAN_POINT ( 'NONE',  ( -35.50000000000000000, -114.2899554544714960, 8.528375582263644006 ) ) ;
#25320=CARTESIAN_POINT ( 'NONE',  ( -35.50000000000000711, -112.6043641208289188, 1.789429170677330649 ) ) ;
#25331=CARTESIAN_POINT ( 'NONE',  ( -37.05926240293131713, -113.0000000000000000, 3.621475545821551734 ) ) ;
#25358=CARTESIAN_POINT ( 'NONE',  ( -34.50000000000000000, -115.0140978167138712, -0.4997823525984417259 ) ) ;
#25361=CARTESIAN_POINT ( 'NONE',  ( -39.00000000000000711, -114.9929510916434339, 12.26648026267477043 ) ) ;
#25368=CARTESIAN_POINT ( 'NONE',  ( -34.50000000000000000, -114.2450133963102843, 8.522190569412378736 ) ) ;
#25377=CARTESIAN_POINT ( 'NONE',  ( -40.02454729103296671, -115.1833782841879525, 6.659774454178448266 ) ) ;
#25379=CARTESIAN_POINT ( 'NONE',  ( -35.50000000000000711, -112.0221129971568104, -0.7553032835231431319 ) ) ;
#25397=CARTESIAN_POINT ( 'NONE',  ( -34.50000000000000000, -116.0215255531121983, -2.372276521655488857 ) ) ;
#25402=CARTESIAN_POINT ( 'NONE',  ( -36.62499999999902656, -114.9929510916434339, 13.11852480586264669 ) ) ;
#25403=CARTESIAN_POINT ( 'NONE',  ( -38.99518666717493431, -113.9929510916434339, 12.74107470552714894 ) ) ;
#25408=CARTESIAN_POINT ( 'NONE',  ( -34.50000000000000000, -113.9929510916434339, 10.50625754673587409 ) ) ;
#25410=CARTESIAN_POINT ( 'NONE',  ( -35.50000000000000711, -114.9929510916434339, 11.91443571948719971 ) ) ;
#25423=CARTESIAN_POINT ( 'NONE',  ( -35.50000000000000000, -114.1807644833817648, -0.6247823525984269599 ) ) ;
#25425=CARTESIAN_POINT ( 'NONE',  ( -37.88768952767750164, -115.9754527089670262, 3.472274454178448266 ) ) ;
#25427=CARTESIAN_POINT ( 'NONE',  ( -37.88768952767750164, -115.9754527089670262, 3.472274454178448266 ) ) ;
#25431=CARTESIAN_POINT ( 'NONE',  ( -35.50000000000000000, -117.0140978167138854, -0.3747823525984422255 ) ) ;
#25434=CARTESIAN_POINT ( 'NONE',  ( -38.37230871539094323, -112.5438815906447729, 3.941024454178448710 ) ) ;
#25439=CARTESIAN_POINT ( 'NONE',  ( -34.50000000000000000, -112.6043641208289188, 1.789429170677330649 ) ) ;
#25448=CARTESIAN_POINT ( 'NONE',  ( -36.24999999999983658, -113.9929510916434339, 13.11852480586264846 ) ) ;
#25451=CARTESIAN_POINT ( 'NONE',  ( -34.50000000000000000, -113.6974040292745656, 2.970979214817929481 ) ) ;
#25452=CARTESIAN_POINT ( 'NONE',  ( -38.25557080230232998, -115.9929510916434481, 13.92914543265419525 ) ) ;
#25474=CARTESIAN_POINT ( 'NONE',  ( -35.99999999999999289, -113.9407375970686758, 6.996475545821551734 ) ) ;
#25482=CARTESIAN_POINT ( 'NONE',  ( -35.50000000000000711, -114.9307644833806137, -1.624782352598427959 ) ) ;
#25485=CARTESIAN_POINT ( 'NONE',  ( -35.50000000000000711, -114.9929510916434339, 12.26648026267477221 ) ) ;
#25490=CARTESIAN_POINT ( 'NONE',  ( -34.50000000000000000, -114.9912366357066986, 10.44580456020104720 ) ) ;
#25494=CARTESIAN_POINT ( 'NONE',  ( -35.50000000000000000, -114.1928420708668028, 8.515919878418792166 ) ) ;
#25495=CARTESIAN_POINT ( 'NONE',  ( -35.50000000000000711, -112.8655373925166572, 1.864575885149403423 ) ) ;
#25505=CARTESIAN_POINT ( 'NONE',  ( -36.33479806579561000, -114.7490116281687165, 1.691024454178448932 ) ) ;
#25515=CARTESIAN_POINT ( 'NONE',  ( -34.92058450342251064, -116.1632251905417945, 7.691024454178450043 ) ) ;
#25533=CARTESIAN_POINT ( 'NONE',  ( -34.50000000000000000, -115.0140978167140986, -0.6247823525984417259 ) ) ;
#25539=CARTESIAN_POINT ( 'NONE',  ( -34.50000000000000000, -115.9382890315277308, 10.02636389016632812 ) ) ;
#25543=CARTESIAN_POINT ( 'NONE',  ( -39.00000000000000711, -114.9929510916434339, 12.56351784598954779 ) ) ;
#25551=CARTESIAN_POINT ( 'NONE',  ( -39.07941549657749647, -116.1632251905417803, 7.558975545821551734 ) ) ;
#25554=CARTESIAN_POINT ( 'NONE',  ( -35.50000000000000711, -116.0012805033554883, -0.7876962586524312027 ) ) ;
#25568=CARTESIAN_POINT ( 'NONE',  ( -34.97545270896703329, -114.7691647218148745, 4.090225545821551734 ) ) ;
#25575=CARTESIAN_POINT ( 'NONE',  ( -35.50000000000000000, -112.8832452823708792, -2.621568770093253953 ) ) ;
#25578=CARTESIAN_POINT ( 'NONE',  ( -36.87500000000098055, -114.9929510916434339, 13.11852480586264669 ) ) ;
#25580=CARTESIAN_POINT ( 'NONE',  ( -38.98077402996267438, -113.9929510916434339, 12.86289566494346204 ) ) ;
#25583=CARTESIAN_POINT ( 'NONE',  ( -37.69578139638701941, -113.9929510916434339, 14.10650203519847778 ) ) ;
#25585=CARTESIAN_POINT ( 'NONE',  ( -35.95915003344517658, -114.9929510916434339, 13.11692036158763308 ) ) ;
#25592=CARTESIAN_POINT ( 'NONE',  ( -35.50000000000000711, -114.9929510916434339, 10.51725893871048889 ) ) ;
#25602=CARTESIAN_POINT ( 'NONE',  ( -35.50000000000000000, -115.0140978167138712, -0.1247823525984438492 ) ) ;
#25605=CARTESIAN_POINT ( 'NONE',  ( -35.00000000000000000, -114.0592624029313242, 1.503524454178448710 ) ) ;
#25607=CARTESIAN_POINT ( 'NONE',  ( -36.11231047232249125, -112.0245472910329880, 4.222274454178449155 ) ) ;
#25609=CARTESIAN_POINT ( 'NONE',  ( -35.50000000000000711, -115.3362660311619692, -1.573728109101206085 ) ) ;
#25618=CARTESIAN_POINT ( 'NONE',  ( -34.50000000000000000, -112.6605569508015350, 1.812590711673265575 ) ) ;
#25625=CARTESIAN_POINT ( 'NONE',  ( -37.99599240977853754, -113.9929510916434339, 12.68378527132499656 ) ) ;
#25628=CARTESIAN_POINT ( 'NONE',  ( -36.31249999999994316, -113.9929510916434339, 13.11852480586264846 ) ) ;
#25629=CARTESIAN_POINT ( 'NONE',  ( -35.83891589277641287, -115.9929510916434481, 13.09299768411358400 ) ) ;
#25654=CARTESIAN_POINT ( 'NONE',  ( -36.33479806579561000, -114.7490116281687165, 4.691024454178447378 ) ) ;
#25665=CARTESIAN_POINT ( 'NONE',  ( -35.83891589277640577, -114.9929510916434339, 13.09299768411358222 ) ) ;
#25670=CARTESIAN_POINT ( 'NONE',  ( -34.50000000000000000, -114.6604609523327838, 9.751889438017201428 ) ) ;
#25675=CARTESIAN_POINT ( 'NONE',  ( -35.50000000000000000, -115.9710363517788068, 10.20486393345008835 ) ) ;
#25687=CARTESIAN_POINT ( 'NONE',  ( -37.74901162816869515, -114.6652019342044042, 2.066024454178448710 ) ) ;
#25697=CARTESIAN_POINT ( 'NONE',  ( -38.30190309005061522, -116.9754527089670546, 7.972274454178450043 ) ) ;
#25716=CARTESIAN_POINT ( 'NONE',  ( -34.50000000000000000, -112.9185811467682754, 1.870920967077121411 ) ) ;
#25719=CARTESIAN_POINT ( 'NONE',  ( -34.50000000000000000, -114.3496480102005251, 8.538090462223289379 ) ) ;
#25723=CARTESIAN_POINT ( 'NONE',  ( -34.50000000000000000, -114.4680894751352156, 8.562575367713533225 ) ) ;
#25735=CARTESIAN_POINT ( 'NONE',  ( -34.00000000000000000, -114.0592624029313242, 9.003524454178446490 ) ) ;
#25737=CARTESIAN_POINT ( 'NONE',  ( -35.50000000000000711, -116.0140978167138712, -0.4997823525984418369 ) ) ;
#25749=CARTESIAN_POINT ( 'NONE',  ( -35.62769128460905677, -112.5438815906447729, 5.308975545821551734 ) ) ;
#25754=CARTESIAN_POINT ( 'NONE',  ( -35.50000000000000000, -112.3697613878167658, -2.522673865603075605 ) ) ;
#25759=CARTESIAN_POINT ( 'NONE',  ( -38.00000000000000711, -114.9929510916434339, 12.56351784598954779 ) ) ;
#25761=CARTESIAN_POINT ( 'NONE',  ( -34.50000000000000000, -114.0185793162512908, 9.502217742515812304 ) ) ;
#25764=CARTESIAN_POINT ( 'NONE',  ( -35.51674767832922441, -113.9929510916434339, 14.04194344061634325 ) ) ;
#25766=CARTESIAN_POINT ( 'NONE',  ( -36.01562499999996447, -114.9929510916434339, 13.11852480586264669 ) ) ;
#25775=CARTESIAN_POINT ( 'NONE',  ( -35.50000000000000711, -114.9902084924877954, 10.43071793783961176 ) ) ;
#25785=CARTESIAN_POINT ( 'NONE',  ( -35.50000000000000000, -113.0140978167129617, -0.6247823525984270709 ) ) ;
#25787=CARTESIAN_POINT ( 'NONE',  ( -34.97545270896703329, -113.2308352781851539, 7.409774454178451819 ) ) ;
#25791=CARTESIAN_POINT ( 'NONE',  ( -39.02454729103295961, -114.7691647218148745, 2.159774454178448710 ) ) ;
#25794=CARTESIAN_POINT ( 'NONE',  ( -35.50000000000000711, -113.4307644833805000, -1.624782352598427959 ) ) ;
#25801=CARTESIAN_POINT ( 'NONE',  ( -34.50000000000000000, -116.0140978167138712, -0.4997823525984418369 ) ) ;
#25809=CARTESIAN_POINT ( 'NONE',  ( -36.99999999999988631, -113.9929510916434339, 13.11852480586264846 ) ) ;
#25811=CARTESIAN_POINT ( 'NONE',  ( -34.50000000000000000, -113.0796441757086939, 1.890140615870383956 ) ) ;
#25813=CARTESIAN_POINT ( 'NONE',  ( -35.50000000000000000, -113.9929510916434339, 10.59426868253284226 ) ) ;
#25814=CARTESIAN_POINT ( 'NONE',  ( -35.50000000000000000, -115.9895221797699065, 10.38535157366622563 ) ) ;
#25836=CARTESIAN_POINT ( 'NONE',  ( -34.50000000000000000, -117.0140978167138854, -0.1247823525984438492 ) ) ;
#25840=CARTESIAN_POINT ( 'NONE',  ( -36.94073759706866156, -113.0000000000000000, 2.628524454178448710 ) ) ;
#25844=CARTESIAN_POINT ( 'NONE',  ( -34.50000000000000000, -113.0140978167134449, 0.8752176474011410523 ) ) ;
#25845=CARTESIAN_POINT ( 'NONE',  ( -35.50000000000000711, -115.8878449012421754, -1.128496220799388494 ) ) ;
#25849=CARTESIAN_POINT ( 'NONE',  ( -35.50000000000000711, -114.9929510916434339, 12.59102132592610523 ) ) ;
#25853=CARTESIAN_POINT ( 'NONE',  ( -34.50000000000000000, -114.9929510916434339, 12.17846912687782712 ) ) ;
#25860=CARTESIAN_POINT ( 'NONE',  ( -35.50000000000000000, -115.7766462221073454, 9.569741527169023598 ) ) ;
#25861=CARTESIAN_POINT ( 'NONE',  ( -35.50000000000000711, -112.0140978167138712, 0.6252176474015680441 ) ) ;
#25872=CARTESIAN_POINT ( 'NONE',  ( -36.25098837183130485, -114.6652019342044184, 7.183975545821551734 ) ) ;
#25879=CARTESIAN_POINT ( 'NONE',  ( -39.99999999999999289, -114.0592624029313242, 6.246475545821551734 ) ) ;
#25895=CARTESIAN_POINT ( 'NONE',  ( -34.50000000000000000, -115.0140978167138712, 0.3752176474015737617 ) ) ;
#25898=CARTESIAN_POINT ( 'NONE',  ( -34.50000000000000000, -115.9895221797699065, 10.38535157366622563 ) ) ;
#25902=CARTESIAN_POINT ( 'NONE',  ( -34.50000000000000000, -114.1185248058629611, 8.507048908356933836 ) ) ;
#25911=CARTESIAN_POINT ( 'NONE',  ( -36.94073759706868287, -116.9999999999999858, 2.871475545821551290 ) ) ;
#25913=CARTESIAN_POINT ( 'NONE',  ( -35.50000000000000000, -114.1185248058627053, 1.007048908356900085 ) ) ;
#25921=CARTESIAN_POINT ( 'NONE',  ( -35.54388159064475872, -115.3723087153909432, 5.683975545821551734 ) ) ;
#25927=CARTESIAN_POINT ( 'NONE',  ( -35.50000000000000000, -114.3474311500471572, -2.624782352598442614 ) ) ;
#25934=CARTESIAN_POINT ( 'NONE',  ( -37.99899697755054717, -114.9929510916434339, 12.65121853911336736 ) ) ;
#25936=CARTESIAN_POINT ( 'NONE',  ( -38.42182118622945808, -113.9929510916434339, 13.81802396319329773 ) ) ;
#25940=CARTESIAN_POINT ( 'NONE',  ( -38.99699093265172678, -113.9929510916434339, 12.71660600561481402 ) ) ;
#25942=CARTESIAN_POINT ( 'NONE',  ( -35.50100302244946704, -114.9929510916434339, 12.65121853911337269 ) ) ;
#25946=ORIENTED_EDGE ( 'NONE', *, *, #17320, .F. ) ;
#25947=CARTESIAN_POINT ( 'NONE',  ( -35.51597953369718397, -114.9929510916434339, 12.74811950270164473 ) ) ;
#25949=CARTESIAN_POINT ( 'NONE',  ( -38.99999999999999289, -113.9407375970686900, 3.753524454178449155 ) ) ;
#25953=CARTESIAN_POINT ( 'NONE',  ( -34.50000000000000000, -113.0140978167142833, 0.8752176474015604946 ) ) ;
#25955=CARTESIAN_POINT ( 'NONE',  ( -36.11231047232249125, -112.0245472910329880, 7.222274454178451819 ) ) ;
#25958=CARTESIAN_POINT ( 'NONE',  ( -35.02454729103298803, -114.8876895276775087, 6.097274454178449155 ) ) ;
#25962=CARTESIAN_POINT ( 'NONE',  ( -35.50000000000000711, -112.8835768857893527, -1.616767172155725740 ) ) ;
#25969=CARTESIAN_POINT ( 'NONE',  ( -34.50000000000000000, -112.8920926830253677, 2.874852253704053062 ) ) ;
#25977=CARTESIAN_POINT ( 'NONE',  ( -37.98402046630260287, -113.9929510916434339, 12.74811950270164296 ) ) ;
#25982=CARTESIAN_POINT ( 'NONE',  ( -35.50000000000000000, -113.9929510916434339, 12.56351784598954424 ) ) ;
#25984=CARTESIAN_POINT ( 'NONE',  ( -35.49999931242378182, -115.9929510916434481, 12.61439929482945743 ) ) ;
#25993=CARTESIAN_POINT ( 'NONE',  ( -35.50000000000000711, -112.8356783780338759, 1.859636627348750348 ) ) ;
#26000=CARTESIAN_POINT ( 'NONE',  ( -34.50000000000000000, -114.6807644833805000, -2.624782352598442614 ) ) ;
#26005=CARTESIAN_POINT ( 'NONE',  ( -38.02454729103296671, -114.3549511594417396, 2.159774454178448710 ) ) ;
#26006=ORIENTED_EDGE ( 'NONE', *, *, #9269, .F. ) ;
#26011=CARTESIAN_POINT ( 'NONE',  ( -34.50000000000000000, -113.0140978167139991, 0.8752176474014555785 ) ) ;
#26019=CARTESIAN_POINT ( 'NONE',  ( -35.50000000000000711, -114.9929510916434339, 11.38636890470581164 ) ) ;
#26023=CARTESIAN_POINT ( 'NONE',  ( -37.49023442168701337, -114.9929510916434339, 14.11852773550420359 ) ) ;
#26027=CARTESIAN_POINT ( 'NONE',  ( -39.00000000000000000, -115.9929510916434481, 12.17846912687782179 ) ) ;
#26029=CARTESIAN_POINT ( 'NONE',  ( -35.50000000000000711, -114.6807644833805000, -1.624782352598427959 ) ) ;
#26037=CARTESIAN_POINT ( 'NONE',  ( -37.99999999999998579, -114.0592624029313242, 7.746475545821553510 ) ) ;
#26049=CARTESIAN_POINT ( 'NONE',  ( -40.02454729103296671, -112.8166217158120332, 7.840225545821554398 ) ) ;
#26066=CARTESIAN_POINT ( 'NONE',  ( -34.50000000000000000, -112.0577668799241309, 1.173706424699810569 ) ) ;
#26070=CARTESIAN_POINT ( 'NONE',  ( -37.42187499999996447, -115.9929510916434481, 14.11852480586265024 ) ) ;
#26073=CARTESIAN_POINT ( 'NONE',  ( -39.00000000000000711, -114.9929510916434339, 12.53051367006571937 ) ) ;
#26082=CARTESIAN_POINT ( 'NONE',  ( -34.02454729103297382, -112.6980969099494132, 5.402725545821552622 ) ) ;
#26084=CARTESIAN_POINT ( 'NONE',  ( -35.50000000000000000, -113.0140978167129617, -0.6247823525984270709 ) ) ;
#26096=CARTESIAN_POINT ( 'NONE',  ( -38.45611840935523418, -112.6276912846090568, 6.433975545821550845 ) ) ;
#26101=CARTESIAN_POINT ( 'NONE',  ( -35.50000000000000000, -113.8474311500459777, -2.624782352598442614 ) ) ;
#26107=CARTESIAN_POINT ( 'NONE',  ( -38.00000000000000711, -114.9929510916434339, 12.59652202191340820 ) ) ;
#26108=CARTESIAN_POINT ( 'NONE',  ( -34.50000000000000000, -114.9929510916434339, 10.72628538622835670 ) ) ;
#26110=CARTESIAN_POINT ( 'NONE',  ( -35.95915003344517658, -114.9929510916434339, 13.11692036158763308 ) ) ;
#26112=CARTESIAN_POINT ( 'NONE',  ( -35.93867112612154102, -113.9929510916434339, 14.11732072679899197 ) ) ;
#26114=CARTESIAN_POINT ( 'NONE',  ( -35.50400759022159036, -114.9929510916434339, 12.68378527132497524 ) ) ;
#26120=CARTESIAN_POINT ( 'NONE',  ( -35.50400759022159036, -114.9929510916434339, 12.68378527132497524 ) ) ;
#26122=CARTESIAN_POINT ( 'NONE',  ( -38.45611840935523418, -115.3723087153909432, 2.066024454178448710 ) ) ;
#26129=CARTESIAN_POINT ( 'NONE',  ( -34.50000000000000000, -113.0140978167138712, -0.3122823525984338988 ) ) ;
#26133=CARTESIAN_POINT ( 'NONE',  ( -39.02454729103295961, -114.7691647218148745, 6.659774454178450043 ) ) ;
#26135=CARTESIAN_POINT ( 'NONE',  ( -35.50000000000000711, -113.3474311500483935, -1.624782352598427959 ) ) ;
#26143=CARTESIAN_POINT ( 'NONE',  ( -34.50000000000000000, -113.2224311500466030, -1.624782352598427959 ) ) ;
#26144=CARTESIAN_POINT ( 'NONE',  ( -35.50000000000000711, -112.0209493036498287, 0.9959249592223760050 ) ) ;
#26149=CARTESIAN_POINT ( 'NONE',  ( -37.56526046546249376, -113.9929510916434339, 13.11451721564129258 ) ) ;
#26152=CARTESIAN_POINT ( 'NONE',  ( -35.50000102263781798, -113.9929510916434339, 12.62466071271731494 ) ) ;
#26154=CARTESIAN_POINT ( 'NONE',  ( -35.50000000000000000, -115.9929081983957104, 10.49113315946066294 ) ) ;
#26165=CARTESIAN_POINT ( 'NONE',  ( -35.50000000000000711, -114.1807644833817648, -1.624782352598427959 ) ) ;
#26175=CARTESIAN_POINT ( 'NONE',  ( -34.50000000000000000, -111.0141141789186605, -0.6738694770610589302 ) ) ;
#26179=CARTESIAN_POINT ( 'NONE',  ( -37.66520193420439711, -114.7490116281687023, 9.058975545821549957 ) ) ;
#26184=CARTESIAN_POINT ( 'NONE',  ( -35.50000000000000000, -114.1807644833817648, -0.6247823525984269599 ) ) ;
#26187=CARTESIAN_POINT ( 'NONE',  ( -38.50000000000000711, -114.9929510916434339, 10.50625754673587231 ) ) ;
#26189=CARTESIAN_POINT ( 'NONE',  ( -35.91854304697313438, -114.9929510916434339, 13.11211614918345703 ) ) ;
#26192=CARTESIAN_POINT ( 'NONE',  ( -36.07812499999994316, -114.9929510916434339, 14.11852480586264846 ) ) ;
#26197=CARTESIAN_POINT ( 'NONE',  ( -35.50000000000000000, -115.9929510916434481, 12.59102132592610346 ) ) ;
#26198=CARTESIAN_POINT ( 'NONE',  ( -35.50000000000000711, -115.9630435732166518, -0.9469505670456015434 ) ) ;
#26211=CARTESIAN_POINT ( 'NONE',  ( -37.97545270896702618, -114.4734759653044023, 9.152725545821551734 ) ) ;
#26219=CARTESIAN_POINT ( 'NONE',  ( -34.97545270896703329, -114.7691647218148745, 2.590225545821551734 ) ) ;
#26242=CARTESIAN_POINT ( 'NONE',  ( -35.80421860361284558, -115.9929510916434481, 14.10650203519841916 ) ) ;
#26247=CARTESIAN_POINT ( 'NONE',  ( -34.50000000000000000, -115.9915791193162420, 10.43066258751475139 ) ) ;
#26257=CARTESIAN_POINT ( 'NONE',  ( -40.02454729103296671, -112.8166217158120332, 3.340225545821551290 ) ) ;
#26261=CARTESIAN_POINT ( 'NONE',  ( -35.50000000000000000, -113.0140978167138712, 0.0002176474015660057743 ) ) ;
#26279=CARTESIAN_POINT ( 'NONE',  ( -35.50000000000000000, -111.7850029017436810, -2.224114562373086912 ) ) ;
#26284=CARTESIAN_POINT ( 'NONE',  ( -37.51635661748575501, -114.9929510916434339, 13.11827392651459157 ) ) ;
#26289=CARTESIAN_POINT ( 'NONE',  ( -34.50000000000000000, -114.9929510916434339, 10.55026311463432087 ) ) ;
#26293=CARTESIAN_POINT ( 'NONE',  ( -37.80727372874345349, -114.9929510916434339, 13.01835785830664527 ) ) ;
#26295=CARTESIAN_POINT ( 'NONE',  ( -39.00000000000000000, -113.9929510916434339, 11.91443571948719615 ) ) ;
#26303=CARTESIAN_POINT ( 'NONE',  ( -35.50000000000000711, -114.9929510916434339, 10.94631322572069365 ) ) ;
#26306=CARTESIAN_POINT ( 'NONE',  ( -36.23083527818512550, -116.0245472910329880, 1.784774454178448932 ) ) ;
#26312=CARTESIAN_POINT ( 'NONE',  ( -34.50000000000000000, -113.0140978167137717, -0.6411448143358797758 ) ) ;
#26314=CARTESIAN_POINT ( 'NONE',  ( -38.99999999999999289, -113.9407375970686900, 6.753524454178448266 ) ) ;
#26316=CARTESIAN_POINT ( 'NONE',  ( -38.30190309005061522, -116.9754527089670546, 1.972274454178448932 ) ) ;
#26321=CARTESIAN_POINT ( 'NONE',  ( -35.50000000000000711, -116.0140896356112989, -0.6575071456984549201 ) ) ;
#26329=CARTESIAN_POINT ( 'NONE',  ( -34.50000000000000000, -112.8690837874180062, 2.872105769100646189 ) ) ;
#26330=CARTESIAN_POINT ( 'NONE',  ( -35.50000000000000711, -112.1222502514821144, 1.343475657184566296 ) ) ;
#26338=CARTESIAN_POINT ( 'NONE',  ( -38.00000000000000711, -113.9929510916434339, 11.21034663311206181 ) ) ;
#26340=CARTESIAN_POINT ( 'NONE',  ( -35.50000000000000000, -113.9929510916434339, 10.68227981832981044 ) ) ;
#26342=CARTESIAN_POINT ( 'NONE',  ( -35.91854304697312728, -115.9929510916434481, 13.11211614918345703 ) ) ;
#26353=CARTESIAN_POINT ( 'NONE',  ( -35.50000000000000711, -115.0795240838853886, -1.623175561345890472 ) ) ;
#26356=CARTESIAN_POINT ( 'NONE',  ( -35.50000000000000711, -114.1264797827112574, 9.515205387299289441 ) ) ;
#26360=CARTESIAN_POINT ( 'NONE',  ( -34.50000000000000000, -112.7530559548648341, -2.608751991713152307 ) ) ;
#26364=CARTESIAN_POINT ( 'NONE',  ( -37.97545270896701908, -113.5265240346955977, 5.347274454178449155 ) ) ;
#26370=CARTESIAN_POINT ( 'NONE',  ( -35.50000000000000000, -115.0140978167138712, 0.0002176474015578471800 ) ) ;
#26374=CARTESIAN_POINT ( 'NONE',  ( -37.66108410722335265, -114.9929510916434339, 13.09299768411426790 ) ) ;
#26377=CARTESIAN_POINT ( 'NONE',  ( -34.57658136524562309, -114.9929510916434339, 13.10177712753338497 ) ) ;
#26382=CARTESIAN_POINT ( 'NONE',  ( -35.60016694755736211, -115.9929510916434481, 12.92579853460621386 ) ) ;
#26383=CARTESIAN_POINT ( 'NONE',  ( -35.50000000000000711, -116.0140978167138712, 0.6252176474015648244 ) ) ;
#26396=CARTESIAN_POINT ( 'NONE',  ( -35.99999999999999289, -114.0592624029313242, 4.503524454178447378 ) ) ;
#26404=CARTESIAN_POINT ( 'NONE',  ( -37.76916472181486739, -116.0245472910329880, 2.965225545821551290 ) ) ;
#26428=CARTESIAN_POINT ( 'NONE',  ( -36.01562499999997158, -115.9929510916434481, 14.11852480586265024 ) ) ;
#26430=CARTESIAN_POINT ( 'NONE',  ( -36.94073759706868287, -112.0000000000000142, 4.128524454178449155 ) ) ;
#26432=CARTESIAN_POINT ( 'NONE',  ( -34.50000000000000000, -115.9929524668003182, 10.51038305125561401 ) ) ;
#26441=CARTESIAN_POINT ( 'NONE',  ( -37.05926240293131713, -112.0000000000000142, 5.121475545821551734 ) ) ;
#26443=CARTESIAN_POINT ( 'NONE',  ( -35.50000000000000000, -113.0140978167138712, -0.6247823525985405357 ) ) ;
#26462=CARTESIAN_POINT ( 'NONE',  ( -35.50000000000000711, -113.0557643173828524, -1.624792769101735868 ) ) ;
#26471=CARTESIAN_POINT ( 'NONE',  ( -34.50000000000000000, -112.9415908020655195, 1.873661708251232572 ) ) ;
#26472=CARTESIAN_POINT ( 'NONE',  ( -34.50015059926905536, -114.9929510916434339, 12.64306614848962695 ) ) ;
#26474=CARTESIAN_POINT ( 'NONE',  ( -37.50613590685470911, -114.9929510916434339, 13.11852378322482515 ) ) ;
#26478=CARTESIAN_POINT ( 'NONE',  ( -34.50000000000000000, -114.1264797827112574, 9.515205387299289441 ) ) ;
#26483=( NAMED_UNIT ( * ) SI_UNIT ( $, .STERADIAN. ) SOLID_ANGLE_UNIT ( ) );
#26488=CARTESIAN_POINT ( 'NONE',  ( -37.80727372874345349, -114.9929510916434339, 13.01835785830664527 ) ) ;
#26495=CARTESIAN_POINT ( 'NONE',  ( -34.50000000000000000, -113.0256022645180707, 0.8765908897032291813 ) ) ;
#26500=CARTESIAN_POINT ( 'NONE',  ( -38.99999999999999289, -113.9407375970686900, 8.253524454178448266 ) ) ;
#26514=CARTESIAN_POINT ( 'NONE',  ( -34.50000000000000000, -115.0795240838853886, -1.623175561345890472 ) ) ;
#26522=CARTESIAN_POINT ( 'NONE',  ( -38.00000000000000711, -113.9929510916434339, 12.17846912687782179 ) ) ;
#26525=CARTESIAN_POINT ( 'NONE',  ( -37.89983305244309264, -113.9929510916434339, 12.92579853460519423 ) ) ;
#26526=CARTESIAN_POINT ( 'NONE',  ( -37.93687354226506869, -115.9929510916434481, 12.87038173996323565 ) ) ;
#26537=CARTESIAN_POINT ( 'NONE',  ( -35.50000000000000711, -112.0157046079661995, -0.6902086197697556713 ) ) ;
#26539=CARTESIAN_POINT ( 'NONE',  ( -35.50000000000000711, -114.2305202833893816, 9.534416457224700991 ) ) ;
#26545=CARTESIAN_POINT ( 'NONE',  ( -34.50000000000000000, -114.8474311500471572, -2.624782352598442614 ) ) ;
#26550=CARTESIAN_POINT ( 'NONE',  ( -36.94073759706866156, -113.0000000000000000, 8.628524454178448266 ) ) ;
#26554=CARTESIAN_POINT ( 'NONE',  ( -35.50000000000000000, -113.3474311500483935, -0.6247823525984269599 ) ) ;
#26560=CARTESIAN_POINT ( 'NONE',  ( -35.50000000000000000, -113.9557924591415627, 10.50182206170499555 ) ) ;
#26562=CARTESIAN_POINT ( 'NONE',  ( -35.80421860361284558, -114.9929510916434339, 14.10650203519841916 ) ) ;
#26566=CARTESIAN_POINT ( 'NONE',  ( -36.50000000000010658, -115.9929510916434481, 13.11852480586264846 ) ) ;
#26578=CARTESIAN_POINT ( 'NONE',  ( -36.64504884055823908, -115.0245472910329880, 4.784774454178448266 ) ) ;
#26587=CARTESIAN_POINT ( 'NONE',  ( -39.07941549657749647, -116.1632251905417803, 6.058975545821550845 ) ) ;
#26589=CARTESIAN_POINT ( 'NONE',  ( 0.000000000000000000, 0.000000000000000000, 0.000000000000000000 ) ) ;
#26608=CARTESIAN_POINT ( 'NONE',  ( -34.50000000000000000, -115.9929510916434481, 12.17846912687782712 ) ) ;
#26610=CARTESIAN_POINT ( 'NONE',  ( -37.88768952767750164, -115.9754527089670262, 7.972274454178450043 ) ) ;
#26611=CARTESIAN_POINT ( 'NONE',  ( -34.50000000000000000, -114.5266723804073195, 8.577838247824468354 ) ) ;
#26622=CARTESIAN_POINT ( 'NONE',  ( -36.94073759706868287, -115.9999999999999858, 2.871475545821551290 ) ) ;
#26624=CARTESIAN_POINT ( 'NONE',  ( -35.50000000000000000, -113.0140978167138712, 0.8127176474015720409 ) ) ;
#26637=CARTESIAN_POINT ( 'NONE',  ( -35.62769128460905677, -112.5438815906447729, 9.808975545821551734 ) ) ;
#26645=CARTESIAN_POINT ( 'NONE',  ( -35.50000000000000711, -112.0460568841087223, -0.8839717462762063382 ) ) ;
#26652=CARTESIAN_POINT ( 'NONE',  ( -34.50000000000000000, -114.9912366357066986, 10.44580456020104720 ) ) ;
#26655=CARTESIAN_POINT ( 'NONE',  ( -36.50000000000011369, -114.9929510916434339, 13.11852480586264669 ) ) ;
#26657=CARTESIAN_POINT ( 'NONE',  ( -34.50000000000000000, -114.8211182053456838, 9.932864235516914775 ) ) ;
#26660=CARTESIAN_POINT ( 'NONE',  ( -38.00000000000000711, -114.9929510916434339, 10.50625754673587231 ) ) ;
#26666=CARTESIAN_POINT ( 'NONE',  ( -37.43749999999998579, -114.9929510916434339, 13.11852480586264669 ) ) ;
#26668=CARTESIAN_POINT ( 'NONE',  ( -35.54388159064475872, -112.6276912846090568, 7.316024454178449155 ) ) ;
#26679=CARTESIAN_POINT ( 'NONE',  ( -39.07941549657748936, -111.8367748094582055, 3.941024454178448710 ) ) ;
#26692=CARTESIAN_POINT ( 'NONE',  ( -34.50000000000000000, -112.4957190293567066, -2.560864217808777266 ) ) ;
#26697=CARTESIAN_POINT ( 'NONE',  ( -38.00000000000000711, -113.9929510916434339, 12.57451923796417681 ) ) ;
#26700=CARTESIAN_POINT ( 'NONE',  ( -34.50000000000000000, -113.9697269463297431, 10.50348536859153370 ) ) ;
#26702=CARTESIAN_POINT ( 'NONE',  ( -37.75185693410092824, -115.9929510916434481, 13.05539834812634759 ) ) ;
#26714=CARTESIAN_POINT ( 'NONE',  ( -35.50000000000000711, -112.0414288467712112, 1.115164475686276191 ) ) ;
#26718=CARTESIAN_POINT ( 'NONE',  ( -35.50000000000000711, -114.1068310684433129, 9.512752019463897923 ) ) ;
#26722=CARTESIAN_POINT ( 'NONE',  ( -35.50000000000000000, -111.0140978167138570, 0.0002176474015660057743 ) ) ;
#26726=CARTESIAN_POINT ( 'NONE',  ( -36.94073759706866156, -113.0000000000000000, 7.128524454178450043 ) ) ;
#26730=CARTESIAN_POINT ( 'NONE',  ( -34.50000000000000000, -115.0140978167138712, -0.6247823525984418369 ) ) ;
#26736=CARTESIAN_POINT ( 'NONE',  ( -37.50818044754229419, -114.9929510916434339, 13.11847460610629668 ) ) ;
#26739=CARTESIAN_POINT ( 'NONE',  ( -34.50000000000000000, -112.0140978167138712, 0.7502176474015694874 ) ) ;
#26741=CARTESIAN_POINT ( 'NONE',  ( -34.50015059926905536, -114.9929510916434339, 12.64306614848962695 ) ) ;
#26746=CARTESIAN_POINT ( 'NONE',  ( -35.50100302244945993, -115.9929510916434481, 12.65121853911337446 ) ) ;
#26747=CARTESIAN_POINT ( 'NONE',  ( -35.50000000000000711, -114.9307644833806137, -1.624782352598427959 ) ) ;
#26757=CARTESIAN_POINT ( 'NONE',  ( -37.05926240293133134, -115.0000000000000000, 7.878524454178450043 ) ) ;
#26767=CARTESIAN_POINT ( 'NONE',  ( -38.37230871539094323, -115.4561184093552413, 4.558975545821550845 ) ) ;
#26782=DIRECTION ( 'NONE',  ( 0.000000000000000000, 0.000000000000000000, 1.000000000000000000 ) ) ;
#26786=CARTESIAN_POINT ( 'NONE',  ( -36.11231047232249836, -112.0245472910329880, 5.722274454178448266 ) ) ;
#26787=CARTESIAN_POINT ( 'NONE',  ( -34.50000306791346816, -115.9929510916434481, 12.62875129555796150 ) ) ;
#26797=CARTESIAN_POINT ( 'NONE',  ( -39.16322519054178741, -111.9205845034225177, 9.433975545821549957 ) ) ;
#26819=CARTESIAN_POINT ( 'NONE',  ( -35.50000000000000711, -112.0414288467712112, 1.115164475686276191 ) ) ;
#26826=CARTESIAN_POINT ( 'NONE',  ( -34.68937937320795584, -114.9929510916434339, 13.37409560816408671 ) ) ;
#26829=CARTESIAN_POINT ( 'NONE',  ( -37.99899697755054717, -114.9929510916434339, 12.65121853911336736 ) ) ;
#26831=CARTESIAN_POINT ( 'NONE',  ( -34.50000000000000000, -114.1091535596544873, 9.513028657562415447 ) ) ;
#26834=CARTESIAN_POINT ( 'NONE',  ( -37.62959469683911351, -114.9929510916434339, 13.10254527216511633 ) ) ;
#26842=CARTESIAN_POINT ( 'NONE',  ( -37.75185693410092824, -114.9929510916434339, 13.05539834812634581 ) ) ;
#26845=CARTESIAN_POINT ( 'NONE',  ( -40.02454729103296671, -115.1833782841879525, 2.159774454178448710 ) ) ;
#26853=CARTESIAN_POINT ( 'NONE',  ( -34.00000000000000000, -114.0592624029313242, 4.503524454178447378 ) ) ;
#26867=CARTESIAN_POINT ( 'NONE',  ( -34.50000000000000000, -112.8230659962028994, 2.866612799894348029 ) ) ;
#26874=CARTESIAN_POINT ( 'NONE',  ( -35.50000000000000711, -114.1302255537607095, 9.515717283514957714 ) ) ;
#26876=CARTESIAN_POINT ( 'NONE',  ( -34.50000000000000000, -113.9929510916434339, 10.53376102667243508 ) ) ;
#26881=CARTESIAN_POINT ( 'NONE',  ( -37.50613590685470911, -113.9929510916434339, 13.11852378322482515 ) ) ;
#26882=CARTESIAN_POINT ( 'NONE',  ( -35.95915003344518368, -115.9929510916434481, 13.11692036158763308 ) ) ;
#26897=CARTESIAN_POINT ( 'NONE',  ( -35.50000000000000711, -112.0209493036498287, 0.9959249592223760050 ) ) ;
#26901=CARTESIAN_POINT ( 'NONE',  ( -35.50000000000000711, -114.9929510916434339, 11.38636890470581164 ) ) ;
#26905=CARTESIAN_POINT ( 'NONE',  ( -35.50000000000000000, -113.0071371610607684, 2.888584676720006961 ) ) ;
#26908=CARTESIAN_POINT ( 'NONE',  ( -38.37230871539094323, -112.5438815906447729, 2.441024454178448710 ) ) ;
#26914=CARTESIAN_POINT ( 'NONE',  ( -34.50000000000000000, -113.0140978167138996, -0.6247823525984306237 ) ) ;
#26921=CARTESIAN_POINT ( 'NONE',  ( -37.48437500000004263, -114.9929510916434339, 13.11852480586264669 ) ) ;
#26927=CARTESIAN_POINT ( 'NONE',  ( -34.50000000000000000, -112.9813730236132585, -1.624774171495860786 ) ) ;
#26931=CARTESIAN_POINT ( 'NONE',  ( -37.50818044754229419, -115.9929510916434481, 13.11847460610629845 ) ) ;
#26952=CARTESIAN_POINT ( 'NONE',  ( -34.97545270896703329, -114.7691647218148745, 4.090225545821551734 ) ) ;
#26973=CARTESIAN_POINT ( 'NONE',  ( -35.02454729103298092, -114.8876895276775087, 3.097274454178448710 ) ) ;
#26974=CARTESIAN_POINT ( 'NONE',  ( -34.50000000000000000, -115.9929510916434481, 10.52826033068511435 ) ) ;
#26982=CARTESIAN_POINT ( 'NONE',  ( -34.02454729103297382, -112.6980969099494132, 8.402725545821549957 ) ) ;
#26999=CARTESIAN_POINT ( 'NONE',  ( -35.50000000000000711, -112.0140978167138712, 0.5627176474015717078 ) ) ;
#27004=CARTESIAN_POINT ( 'NONE',  ( -34.50000000000000000, -115.9821387493194891, -0.8839717462762166633 ) ) ;
#27005=CARTESIAN_POINT ( 'NONE',  ( -39.00000000000000711, -114.9929510916434339, 12.57451923796417503 ) ) ;
#27008=CARTESIAN_POINT ( 'NONE',  ( -38.00000000000000711, -114.9929510916434339, 12.39849696637031151 ) ) ;
#27010=CARTESIAN_POINT ( 'NONE',  ( -34.50000000000000000, -114.9929510916434339, 10.56126450660895699 ) ) ;
#27012=CARTESIAN_POINT ( 'NONE',  ( -37.56526046546250086, -114.9929510916434339, 13.11451721564129258 ) ) ;
#27019=CARTESIAN_POINT ( 'NONE',  ( -38.00000000000000711, -114.9929510916434339, 12.39849696637031151 ) ) ;
#27023=CARTESIAN_POINT ( 'NONE',  ( -37.05926240293131713, -115.9999999999999858, 7.878524454178450043 ) ) ;
#27031=CARTESIAN_POINT ( 'NONE',  ( -39.99999999999999289, -113.9407375970686758, 5.253524454178449155 ) ) ;
#27044=CARTESIAN_POINT ( 'NONE',  ( -34.50000000000000000, -111.0140978167138570, 0.6252176474015680441 ) ) ;
#27051=CARTESIAN_POINT ( 'NONE',  ( -38.00000000000000711, -113.9929510916434339, 11.91443571948719615 ) ) ;
#27054=CARTESIAN_POINT ( 'NONE',  ( -34.50000000000000000, -113.9929510916434339, 10.50625754673586876 ) ) ;
#27055=CARTESIAN_POINT ( 'NONE',  ( -37.99974912065192001, -115.9929510916434481, 12.63488142334838749 ) ) ;
#27066=CARTESIAN_POINT ( 'NONE',  ( -35.50000000000000711, -115.8137639216009234, -1.239329810084483841 ) ) ;
#27069=CARTESIAN_POINT ( 'NONE',  ( -35.50000000000000711, -114.9929510916434339, 10.51725893871048889 ) ) ;
#27074=CARTESIAN_POINT ( 'NONE',  ( -35.50000000000000000, -111.3577635893106361, 2.022004269840791402 ) ) ;
#27078=CARTESIAN_POINT ( 'NONE',  ( -37.97545270896701908, -113.5265240346955977, 8.347274454178448266 ) ) ;
#27083=CARTESIAN_POINT ( 'NONE',  ( -34.50000000000000000, -113.0140978167129617, -0.6247823525984270709 ) ) ;
#27090=CARTESIAN_POINT ( 'NONE',  ( -37.49414064056234253, -114.9929510916434339, 13.11852578240983291 ) ) ;
#27095=CARTESIAN_POINT ( 'NONE',  ( -34.50000000000000000, -113.3474311500483935, -1.624782352598427959 ) ) ;
#27100=CARTESIAN_POINT ( 'NONE',  ( -38.00000000000000711, -115.9929510916434481, 12.56351784598954779 ) ) ;
#27122=CARTESIAN_POINT ( 'NONE',  ( -37.88768952767750875, -112.0245472910329880, 5.027725545821550845 ) ) ;
#27141=CARTESIAN_POINT ( 'NONE',  ( -35.00000000000000000, -114.0592624029313242, 6.003524454178450043 ) ) ;
#27143=CARTESIAN_POINT ( 'NONE',  ( -36.62499999999902656, -115.9929510916434481, 14.11852480586265024 ) ) ;
#27154=CARTESIAN_POINT ( 'NONE',  ( -34.97545270896703329, -114.7691647218148745, 4.090225545821551734 ) ) ;
#27175=CARTESIAN_POINT ( 'NONE',  ( -35.50000000000000711, -112.3465879560236687, 1.629585756119413364 ) ) ;
#27182=CARTESIAN_POINT ( 'NONE',  ( -34.50000000000000000, -112.0651520602111191, -0.9469505670458575608 ) ) ;
#27183=CARTESIAN_POINT ( 'NONE',  ( -37.43749999999998579, -114.9929510916434339, 14.11852480586264846 ) ) ;
#27186=CARTESIAN_POINT ( 'NONE',  ( -35.50000000000000000, -113.9929510916435049, 10.50625754673586876 ) ) ;
#27188=CARTESIAN_POINT ( 'NONE',  ( -34.50000000000000000, -114.9929510916434339, 11.73841344789270202 ) ) ;
#27199=CARTESIAN_POINT ( 'NONE',  ( -37.93687354226506869, -114.9929510916434339, 12.87038173996323565 ) ) ;
#27201=CARTESIAN_POINT ( 'NONE',  ( -38.99999999999999289, -113.9407375970686900, 5.253524454178449155 ) ) ;
#27208=CARTESIAN_POINT ( 'NONE',  ( -39.99999999999999289, -113.9407375970686758, 6.753524454178450043 ) ) ;
#27220=CARTESIAN_POINT ( 'NONE',  ( -34.50000000000000000, -113.0765974847181781, -2.624803185604914102 ) ) ;
#27225=CARTESIAN_POINT ( 'NONE',  ( -35.50000000000000711, -114.9929510916434339, 10.68227981832981044 ) ) ;
#27226=CARTESIAN_POINT ( 'NONE',  ( -34.50000000000000000, -113.9929510916434339, 12.59102132592610346 ) ) ;
#27229=CARTESIAN_POINT ( 'NONE',  ( -38.00000000000000711, -113.9929510916434339, 12.56351784598954779 ) ) ;
#27230=CARTESIAN_POINT ( 'NONE',  ( -35.50000000000000711, -114.9929510916434339, 10.52000928670414126 ) ) ;
#27244=CARTESIAN_POINT ( 'NONE',  ( -35.50000000000000711, -116.0140978167138712, -0.3747823525984422255 ) ) ;
#27247=CARTESIAN_POINT ( 'NONE',  ( -35.50000000000000711, -114.9929510916434339, 11.91443571948719971 ) ) ;
#27251=CARTESIAN_POINT ( 'NONE',  ( -35.50000000000000000, -111.0140978167138570, -0.1247823525984260717 ) ) ;
#27254=CARTESIAN_POINT ( 'NONE',  ( -37.99999999999998579, -113.9407375970686758, 6.753524454178450043 ) ) ;
#27259=CARTESIAN_POINT ( 'NONE',  ( -34.50000000000000000, -113.0140978167138712, -0.6247823525983134951 ) ) ;
#27264=CARTESIAN_POINT ( 'NONE',  ( -35.50000000000000000, -113.9929510916434339, 12.17846912687782712 ) ) ;
#27268=CARTESIAN_POINT ( 'NONE',  ( -34.50000000000000000, -112.2144317118258527, -1.239329810084414341 ) ) ;
#27269=CARTESIAN_POINT ( 'NONE',  ( -36.87500000000098765, -115.9929510916434481, 14.11852480586265024 ) ) ;
#27275=CARTESIAN_POINT ( 'NONE',  ( -35.50000000000000711, -114.1091535596544873, 9.513028657562415447 ) ) ;
#27295=CARTESIAN_POINT ( 'NONE',  ( -36.23083527818512550, -111.9754527089670404, 8.215225545821549957 ) ) ;
#27316=CARTESIAN_POINT ( 'NONE',  ( -38.69949915733018742, -115.9929510916434481, 13.54034599209165890 ) ) ;
#27325=CARTESIAN_POINT ( 'NONE',  ( -35.97545270896705460, -114.3549511594417680, 4.090225545821551734 ) ) ;
#27354=CARTESIAN_POINT ( 'NONE',  ( -34.50000000000000000, -113.3474311500483935, -1.624782352598427959 ) ) ;
#27355=CARTESIAN_POINT ( 'NONE',  ( -35.97545865737298953, -114.9929510916434339, 14.11837420659365705 ) ) ;
#27357=CARTESIAN_POINT ( 'NONE',  ( -35.50000000000000000, -113.9929510916434339, 10.50625754673586876 ) ) ;
#27360=CARTESIAN_POINT ( 'NONE',  ( -34.50000000000000000, -114.9929510916434339, 12.56351784598954424 ) ) ;
#27369=CARTESIAN_POINT ( 'NONE',  ( -38.00000000000000711, -114.9929510916434339, 11.21034663311206181 ) ) ;
#27371=CARTESIAN_POINT ( 'NONE',  ( -34.92058450342251064, -116.1632251905417945, 1.691024454178448932 ) ) ;
#27382=CARTESIAN_POINT ( 'NONE',  ( -35.69809690994938478, -111.0245472910330022, 8.722274454178450043 ) ) ;
#27393=CARTESIAN_POINT ( 'NONE',  ( -34.50000000000000000, -115.3399256288223569, -2.599147725881697291 ) ) ;
#27399=CARTESIAN_POINT ( 'NONE',  ( -35.50000000000000711, -114.9929510916434339, 10.72628538622835670 ) ) ;
#27403=CARTESIAN_POINT ( 'NONE',  ( -36.06250000000000711, -113.9929510916434339, 14.11852480586265024 ) ) ;
#27408=CARTESIAN_POINT ( 'NONE',  ( -34.50000000000000000, -113.9929510916434339, 12.56351784598954424 ) ) ;
#27409=CARTESIAN_POINT ( 'NONE',  ( -39.00000000000000711, -114.9929510916434339, 12.59652202191340820 ) ) ;
#27410=CARTESIAN_POINT ( 'NONE',  ( -35.50000000000000711, -114.0185793162512908, 9.502217742515812304 ) ) ;
#27423=CARTESIAN_POINT ( 'NONE',  ( -35.50000000000000000, -113.0140978167142833, 0.8752176474019800478 ) ) ;
#27425=CARTESIAN_POINT ( 'NONE',  ( -37.35495115944176092, -112.9754527089670688, 4.034774454178449155 ) ) ;
#27426=CARTESIAN_POINT ( 'NONE',  ( -35.50040135968785648, -114.9929510916434339, 12.63896776382214071 ) ) ;
#27432=CARTESIAN_POINT ( 'NONE',  ( -35.50000000000000000, -111.8727710936879589, 2.535339294948415922 ) ) ;
#27435=CARTESIAN_POINT ( 'NONE',  ( -35.00000000000000000, -114.0592624029313242, 7.503524454178449155 ) ) ;
#27442=CARTESIAN_POINT ( 'NONE',  ( -34.50000000000000000, -113.0140978167138712, 0.2502176474015764263 ) ) ;
#27449=CARTESIAN_POINT ( 'NONE',  ( -35.50000000000000000, -113.9929510916436470, 10.50625754673581724 ) ) ;
#27452=CARTESIAN_POINT ( 'NONE',  ( -34.50000000000000000, -111.0140978167138570, -0.3747823525984258497 ) ) ;
#27453=CARTESIAN_POINT ( 'NONE',  ( -35.50000000000000000, -114.1371041221139109, 8.509266650872710613 ) ) ;
#27461=CARTESIAN_POINT ( 'NONE',  ( -38.00000000000000711, -115.9929510916434481, 12.59652202191340820 ) ) ;
#27481=CARTESIAN_POINT ( 'NONE',  ( -38.37230871539094323, -115.4561184093552413, 7.558975545821551734 ) ) ;
#27503=CARTESIAN_POINT ( 'NONE',  ( -38.99924736195577424, -115.9929510916434481, 12.66759465831984599 ) ) ;
#27511=CARTESIAN_POINT ( 'NONE',  ( -36.52652403469559061, -114.9754527089670262, 2.777725545821551734 ) ) ;
#27540=CARTESIAN_POINT ( 'NONE',  ( -34.50000000000000000, -113.1807644833805426, -1.624782352598427959 ) ) ;
#27541=CARTESIAN_POINT ( 'NONE',  ( -36.99999999999989342, -114.9929510916434339, 14.11852480586264846 ) ) ;
#27542=CARTESIAN_POINT ( 'NONE',  ( -35.50000000000000000, -113.9929510916434339, 10.50625754673587409 ) ) ;
#27544=CARTESIAN_POINT ( 'NONE',  ( -35.87745010033553683, -114.9929510916434339, 14.11371147303761298 ) ) ;
#27554=CARTESIAN_POINT ( 'NONE',  ( -35.69809690994938478, -111.0245472910330022, 5.722274454178450043 ) ) ;
#27565=CARTESIAN_POINT ( 'NONE',  ( -40.02454729103296671, -112.8166217158120332, 3.340225545821551290 ) ) ;
#27577=CARTESIAN_POINT ( 'NONE',  ( -34.50000000000000000, -117.0140978167138854, -0.5622823525984408377 ) ) ;
#27581=CARTESIAN_POINT ( 'NONE',  ( -37.49414064056234253, -114.9929510916434339, 13.11852578240983291 ) ) ;
#27584=CARTESIAN_POINT ( 'NONE',  ( -34.51202277066418844, -113.9929510916434339, 12.81430620224972294 ) ) ;
#27588=CARTESIAN_POINT ( 'NONE',  ( -34.50000000000000000, -113.9929510916434339, 10.94631322572069365 ) ) ;
#27590=CARTESIAN_POINT ( 'NONE',  ( -39.00000000000000711, -114.9929510916434339, 12.57451923796417503 ) ) ;
#27592=CARTESIAN_POINT ( 'NONE',  ( -35.50000000000000711, -114.0000000000003411, 9.500000000000035527 ) ) ;
#27604=CARTESIAN_POINT ( 'NONE',  ( -35.50000000000000711, -116.0141056290913610, -0.5935324770972248976 ) ) ;
#27607=CARTESIAN_POINT ( 'NONE',  ( -36.52652403469556930, -113.0245472910329880, 5.722274454178450043 ) ) ;
#27612=CARTESIAN_POINT ( 'NONE',  ( -35.50000000000000000, -115.1449503510569059, -2.621568770093253953 ) ) ;
#27616=CARTESIAN_POINT ( 'NONE',  ( -38.99999999999999289, -113.9407375970686900, 8.253524454178448266 ) ) ;
#27623=CARTESIAN_POINT ( 'NONE',  ( -34.50000000000000000, -112.0577668799241309, 1.173706424699810569 ) ) ;
#27626=CARTESIAN_POINT ( 'NONE',  ( -35.50000000000000000, -113.9929510916434339, 10.50625754673588474 ) ) ;
#27630=CARTESIAN_POINT ( 'NONE',  ( -34.50000000000000000, -116.0060826362711595, -0.7553032835231661135 ) ) ;
#27631=CARTESIAN_POINT ( 'NONE',  ( -38.42182118622945808, -115.9929510916434481, 13.81802396319329773 ) ) ;
#27636=EDGE_LOOP ( 'NONE', ( #3385, #4846, #11866, #14213, #30661 ) ) ;
#27638=CARTESIAN_POINT ( 'NONE',  ( -35.50000000000000711, -114.2305202833893816, 9.534416457224700991 ) ) ;
#27656=CARTESIAN_POINT ( 'NONE',  ( -36.94073759706868287, -115.0000000000000000, 5.871475545821551734 ) ) ;
#27666=FACE_OUTER_BOUND ( 'NONE', #16674, .T. ) ;
#27672=CARTESIAN_POINT ( 'NONE',  ( -39.00000000000000000, -115.9929510916434481, 12.53051367006571937 ) ) ;
#27683=CARTESIAN_POINT ( 'NONE',  ( -35.00000000000000000, -113.9407375970686900, 6.996475545821551734 ) ) ;
#27709=CARTESIAN_POINT ( 'NONE',  ( -34.50000000000000000, -115.6286452741999113, -1.424448457485488095 ) ) ;
#27710=CARTESIAN_POINT ( 'NONE',  ( -37.46874999999996447, -114.9929510916434339, 14.11852480586264846 ) ) ;
#27711=CARTESIAN_POINT ( 'NONE',  ( -35.50000000000000000, -113.9929510916434339, 10.50625754673586876 ) ) ;
#27713=CARTESIAN_POINT ( 'NONE',  ( -36.24999999999983658, -114.9929510916434339, 14.11852480586264846 ) ) ;
#27723=CARTESIAN_POINT ( 'NONE',  ( -38.00000000000000711, -114.9929510916434339, 11.73841344789285657 ) ) ;
#27725=CARTESIAN_POINT ( 'NONE',  ( -39.99999999999999289, -113.9407375970686758, 6.753524454178450043 ) ) ;
#27727=CARTESIAN_POINT ( 'NONE',  ( -35.50000000000000711, -116.0060826362711595, -0.7553032835231661135 ) ) ;
#27745=CARTESIAN_POINT ( 'NONE',  ( -35.50000000000000000, -113.5133328644208746, 2.949007337991939259 ) ) ;
#27748=CARTESIAN_POINT ( 'NONE',  ( -35.96730626674924025, -114.9929510916434339, 13.11752178341330044 ) ) ;
#27750=CARTESIAN_POINT ( 'NONE',  ( -36.24999999999983658, -113.9929510916434339, 14.11852480586265024 ) ) ;
#27755=CARTESIAN_POINT ( 'NONE',  ( -34.50000000000000000, -113.9929510916434339, 10.50625754673588474 ) ) ;
#27756=CARTESIAN_POINT ( 'NONE',  ( -39.00000000000000711, -114.9929510916434339, 12.26648026267477043 ) ) ;
#27757=CARTESIAN_POINT ( 'NONE',  ( -35.50000000000000711, -114.9929510916434339, 10.52826033068511435 ) ) ;
#27773=CARTESIAN_POINT ( 'NONE',  ( -35.50000000000000000, -113.0256022645180707, 0.8765908897032291813 ) ) ;
#27775=CARTESIAN_POINT ( 'NONE',  ( -39.02454729103295961, -114.7691647218148745, 2.159774454178448710 ) ) ;
#27781=CARTESIAN_POINT ( 'NONE',  ( -35.50000000000000711, -112.8655373925166572, 1.864575885149403423 ) ) ;
#27785=CARTESIAN_POINT ( 'NONE',  ( -37.05926240293131713, -115.9999999999999858, 6.378524454178448266 ) ) ;
#27791=CARTESIAN_POINT ( 'NONE',  ( -34.50000000000000000, -112.3465879560236687, 1.629585756119413364 ) ) ;
#27795=CARTESIAN_POINT ( 'NONE',  ( -35.50000000000000000, -113.9929510916434339, 10.59426868253284226 ) ) ;
#27801=CARTESIAN_POINT ( 'NONE',  ( -34.50000000000000000, -115.6286452741999113, -1.424448457485488095 ) ) ;
#27802=CARTESIAN_POINT ( 'NONE',  ( -39.00000000000000000, -115.9929510916434481, 12.60752341388803721 ) ) ;
#27826=CARTESIAN_POINT ( 'NONE',  ( -36.33479806579560289, -113.2509883718313262, 3.808975545821551734 ) ) ;
#27836=CARTESIAN_POINT ( 'NONE',  ( -35.50000000000000711, -114.1189822439768449, 9.514224058074130852 ) ) ;
#27839=CARTESIAN_POINT ( 'NONE',  ( -34.50000000000000000, -114.0371586325023117, 9.504435485030890973 ) ) ;
#27842=CARTESIAN_POINT ( 'NONE',  ( -36.99999999999988631, -115.9929510916434481, 14.11852480586265024 ) ) ;
#27851=CARTESIAN_POINT ( 'NONE',  ( -36.23083527818512550, -111.9754527089670404, 9.715225545821551734 ) ) ;
#27877=CARTESIAN_POINT ( 'NONE',  ( -34.50000000000000000, -114.1835524127412924, 8.514811007161055656 ) ) ;
#27881=CARTESIAN_POINT ( 'NONE',  ( -36.87500000000098055, -114.9929510916434339, 14.11852480586264846 ) ) ;
#27891=CARTESIAN_POINT ( 'NONE',  ( -33.97545270896702618, -112.8166217158120475, 7.409774454178449155 ) ) ;
#27893=CARTESIAN_POINT ( 'NONE',  ( -35.50000000000000711, -112.7549084230351752, -1.592823285203595285 ) ) ;
#27911=CARTESIAN_POINT ( 'NONE',  ( -34.50000000000000000, -117.0140978167138854, -0.4997823525984417259 ) ) ;
#27915=CARTESIAN_POINT ( 'NONE',  ( -35.98364338251434447, -114.9929510916434339, 13.11827392651456314 ) ) ;
#27916=CARTESIAN_POINT ( 'NONE',  ( -36.99999999999988631, -113.9929510916434339, 14.11852480586265024 ) ) ;
#27921=CARTESIAN_POINT ( 'NONE',  ( -34.50000000000000000, -113.9929510916434339, 10.59426868253284226 ) ) ;
#27925=CARTESIAN_POINT ( 'NONE',  ( -35.50000000000000711, -114.1264797827112574, 9.515205387299289441 ) ) ;
#27936=CARTESIAN_POINT ( 'NONE',  ( -35.50000000000000000, -115.0140978167138712, -0.6247823525984407267 ) ) ;
#27938=CARTESIAN_POINT ( 'NONE',  ( -39.02454729103295961, -114.7691647218148745, 3.659774454178448710 ) ) ;
#27945=CARTESIAN_POINT ( 'NONE',  ( -35.50000000000000000, -117.0140978167138854, 0.3752176474015736507 ) ) ;
#27953=CARTESIAN_POINT ( 'NONE',  ( -34.50000000000000000, -112.9415908020655195, 1.873661708251232572 ) ) ;
#27962=CARTESIAN_POINT ( 'NONE',  ( -35.50000000000000000, -113.9929510916434339, 12.44250253426871033 ) ) ;
#27966=CARTESIAN_POINT ( 'NONE',  ( -34.50000000000000000, -115.9630435732166518, -0.9469505670456015434 ) ) ;
#27967=ADVANCED_FACE ( 'NONE', ( #34638 ), #2960, .F. ) ;
#27968=CARTESIAN_POINT ( 'NONE',  ( -35.50000000000000000, -114.3496480102005251, 8.538090462223289379 ) ) ;
#27995=CARTESIAN_POINT ( 'NONE',  ( -37.66520193420439711, -114.7490116281687023, 4.558975545821549957 ) ) ;
#28006=CARTESIAN_POINT ( 'NONE',  ( -35.50000000000000711, -115.0468226098135744, -1.624774171496087716 ) ) ;
#28010=CARTESIAN_POINT ( 'NONE',  ( -35.50000000000000711, -114.9922651054798308, 10.46846006712531008 ) ) ;
#28016=CARTESIAN_POINT ( 'NONE',  ( -34.50000000000000000, -114.9929510916434339, 10.72628538622835670 ) ) ;
#28019=CARTESIAN_POINT ( 'NONE',  ( -35.50000000000000000, -115.9929510916434481, 10.59426868253284226 ) ) ;
#28020=CARTESIAN_POINT ( 'NONE',  ( -35.50000000000000711, -112.0460568841087223, -0.8839717462762063382 ) ) ;
#28030=CARTESIAN_POINT ( 'NONE',  ( -35.02454729103298803, -113.1123104723225197, 8.402725545821549957 ) ) ;
#28039=UNCERTAINTY_MEASURE_WITH_UNIT (LENGTH_MEASURE( 1.000000000000000082E-05 ), #17842, 'distance_accuracy_value', 'NONE');
#28063=CARTESIAN_POINT ( 'NONE',  ( -34.50000000000000000, -113.0140978167138712, -0.6247823525985405357 ) ) ;
#28066=CARTESIAN_POINT ( 'NONE',  ( -34.50000000000000000, -115.9929510916434481, 10.52000928670414126 ) ) ;
#28069=CARTESIAN_POINT ( 'NONE',  ( -34.50000000000000000, -114.2265172349312508, 8.519938377296172760 ) ) ;
#28078=CARTESIAN_POINT ( 'NONE',  ( -34.92058450342251064, -116.1632251905417945, 3.191024454178448710 ) ) ;
#28080=CARTESIAN_POINT ( 'NONE',  ( -35.50000000000000711, -112.0269151300720409, -0.7876962586524208776 ) ) ;
#28097=CARTESIAN_POINT ( 'NONE',  ( -34.50000000000000000, -116.9980674558286040, -0.8858242144478970514 ) ) ;
#28100=CARTESIAN_POINT ( 'NONE',  ( -35.52552712174884419, -114.9929510916434339, 12.77960891308624447 ) ) ;
#28101=CARTESIAN_POINT ( 'NONE',  ( -38.92341863475394348, -113.9929510916434339, 13.10177712753322155 ) ) ;
#28105=CARTESIAN_POINT ( 'NONE',  ( -34.50000000000000000, -113.9929510916434339, 10.61627146648203990 ) ) ;
#28108=CARTESIAN_POINT ( 'NONE',  ( -37.24999999999992895, -114.9929510916434339, 13.11852480586264669 ) ) ;
#28120=CARTESIAN_POINT ( 'NONE',  ( -35.50000000000000000, -113.0140978167138712, -0.6247823525985405357 ) ) ;
#28122=CARTESIAN_POINT ( 'NONE',  ( -35.02454729103298803, -114.8876895276775087, 4.597274454178448266 ) ) ;
#28127=CARTESIAN_POINT ( 'NONE',  ( -35.50000000000000000, -114.9515981487115823, -2.624803185604625000 ) ) ;
#28130=CARTESIAN_POINT ( 'NONE',  ( -39.02454729103295961, -114.7691647218148745, 6.659774454178450043 ) ) ;
#28138=CARTESIAN_POINT ( 'NONE',  ( -34.50000000000000000, -113.2637153405686519, 1.912112492696748989 ) ) ;
#28145=CARTESIAN_POINT ( 'NONE',  ( -35.99386409314529800, -113.9929510916434339, 13.11852378322482515 ) ) ;
#28148=CARTESIAN_POINT ( 'NONE',  ( -34.50000000000000000, -111.0140978167138570, 0.6252176474015680441 ) ) ;
#28149=CARTESIAN_POINT ( 'NONE',  ( -39.00000000000000000, -115.9929510916434481, 12.39849696637031151 ) ) ;
#28173=CARTESIAN_POINT ( 'NONE',  ( -36.94073759706868287, -115.0000000000000000, 4.371475545821550845 ) ) ;
#28182=CARTESIAN_POINT ( 'NONE',  ( -35.50000000000000711, -115.8137639216009234, -1.239329810084483841 ) ) ;
#28191=CARTESIAN_POINT ( 'NONE',  ( -34.50000000000000000, -114.0185793162512908, 9.502217742515812304 ) ) ;
#28193=PRODUCT_DEFINITION_SHAPE ( 'NONE', 'NONE',  #24258 ) ;
#28195=CARTESIAN_POINT ( 'NONE',  ( -35.50000000000000000, -114.2183886307118428, 8.518969274377507617 ) ) ;
#28198=CARTESIAN_POINT ( 'NONE',  ( -35.00000000000000000, -116.0140978167138712, 0.8752176474015622709 ) ) ;
#28207=CARTESIAN_POINT ( 'NONE',  ( -35.99999999999999289, -113.9407375970686758, 9.996475545821549957 ) ) ;
#28215=CARTESIAN_POINT ( 'NONE',  ( -34.83677480945819838, -111.9205845034225462, 8.816024454178446490 ) ) ;
#28231=CARTESIAN_POINT ( 'NONE',  ( -34.50000000000000000, -115.0140978167138712, -0.6247823525984407267 ) ) ;
#28234=CARTESIAN_POINT ( 'NONE',  ( -34.50000000000000000, -114.2675000158779710, 8.525177020294046670 ) ) ;
#28239=CARTESIAN_POINT ( 'NONE',  ( -34.50000000000000000, -114.3496480102005251, 8.538090462223289379 ) ) ;
#28249=CARTESIAN_POINT ( 'NONE',  ( -34.83677480945819838, -111.9205845034225462, 5.816024454178450043 ) ) ;
#28252=CARTESIAN_POINT ( 'NONE',  ( -35.50000000000000711, -113.8474311500459777, -1.624782352598427959 ) ) ;
#28262=CARTESIAN_POINT ( 'NONE',  ( -36.23083527818513261, -111.9754527089670404, 6.715225545821550845 ) ) ;
#28270=CARTESIAN_POINT ( 'NONE',  ( -35.50000000000000000, -116.0215255531121983, -2.372276521655488857 ) ) ;
#28273=CARTESIAN_POINT ( 'NONE',  ( -35.50640865667918433, -114.9929510916434339, 12.69998175888958514 ) ) ;
#28276=CARTESIAN_POINT ( 'NONE',  ( -37.62254989966453422, -113.9929510916434339, 14.11371147303758278 ) ) ;
#28279=CARTESIAN_POINT ( 'NONE',  ( -37.18750000000004974, -113.9929510916434339, 14.11852480586265024 ) ) ;
#28281=CARTESIAN_POINT ( 'NONE',  ( -35.50160444427493189, -114.9929510916434339, 12.65937477241749853 ) ) ;
#28287=CARTESIAN_POINT ( 'NONE',  ( -35.50000000000000711, -114.9929510916434339, 12.60752341388803544 ) ) ;
#28296=CARTESIAN_POINT ( 'NONE',  ( -35.50000000000000000, -115.0140978167138712, -0.3747823525984422255 ) ) ;
#28298=CARTESIAN_POINT ( 'NONE',  ( -36.11231047232249125, -112.0245472910329880, 2.722274454178448266 ) ) ;
#28301=CARTESIAN_POINT ( 'NONE',  ( -35.54388159064475872, -112.6276912846090568, 5.816024454178449155 ) ) ;
#28303=CARTESIAN_POINT ( 'NONE',  ( -35.50000000000000000, -115.0631849411758196, -2.624765990393648885 ) ) ;
#28310=CARTESIAN_POINT ( 'NONE',  ( -34.50000000000000000, -112.0269151300720409, -0.7876962586524208776 ) ) ;
#28318=CARTESIAN_POINT ( 'NONE',  ( -37.24999999999992184, -113.9929510916434339, 13.11852480586264846 ) ) ;
#28319=CARTESIAN_POINT ( 'NONE',  ( -34.50000000000000000, -112.0140978167138712, 0.7502176474015694874 ) ) ;
#28321=CARTESIAN_POINT ( 'NONE',  ( -35.95915003344518368, -113.9929510916434339, 13.11692036158763308 ) ) ;
#28322=CARTESIAN_POINT ( 'NONE',  ( -35.50000000000000000, -115.9929510916434481, 10.53376102667243508 ) ) ;
#28344=CARTESIAN_POINT ( 'NONE',  ( -37.97545270896702618, -114.4734759653044023, 7.652725545821552622 ) ) ;
#28356=CARTESIAN_POINT ( 'NONE',  ( -36.01562499999996447, -114.9929510916434339, 13.11852480586264669 ) ) ;
#28361=CARTESIAN_POINT ( 'NONE',  ( -34.50000000000000000, -114.3464919575557843, 9.568884482464163455 ) ) ;
#28366=CARTESIAN_POINT ( 'NONE',  ( -35.50000000000000000, -115.9929524668003182, 10.51038305125561401 ) ) ;
#28367=CARTESIAN_POINT ( 'NONE',  ( -35.50000000000000711, -112.9876085932806262, 1.879154677457530065 ) ) ;
#28376=CARTESIAN_POINT ( 'NONE',  ( -36.02454729103298092, -114.4734759653044307, 1.597274454178448932 ) ) ;
#28386=CARTESIAN_POINT ( 'NONE',  ( -40.02454729103296671, -115.1833782841879525, 8.159774454178448266 ) ) ;
#28404=CARTESIAN_POINT ( 'NONE',  ( -34.50000000000000000, -112.9876085932806262, 1.879154677457530065 ) ) ;
#28408=CARTESIAN_POINT ( 'NONE',  ( -34.50000000000000000, -115.9929510916434481, 10.59426868253284226 ) ) ;
#28411=CARTESIAN_POINT ( 'NONE',  ( -35.62769128460905677, -115.4561184093552413, 1.691024454178448710 ) ) ;
#28413=CARTESIAN_POINT ( 'NONE',  ( -37.62254989966454133, -114.9929510916434339, 14.11371147303758278 ) ) ;
#28422=CARTESIAN_POINT ( 'NONE',  ( -33.97545270896703329, -115.1833782841879810, 4.090225545821551734 ) ) ;
#28424=CARTESIAN_POINT ( 'NONE',  ( -35.50000000000000711, -112.0140978167138712, 0.3752176474015640473 ) ) ;
#28438=CARTESIAN_POINT ( 'NONE',  ( -37.88768952767750875, -112.0245472910329880, 5.027725545821550845 ) ) ;
#28444=CARTESIAN_POINT ( 'NONE',  ( -35.50000000000000000, -116.9884631899972476, -0.9506101647064282290 ) ) ;
#28449=CARTESIAN_POINT ( 'NONE',  ( -37.98402046630260287, -114.9929510916434339, 12.74811950270164118 ) ) ;
#28450=CARTESIAN_POINT ( 'NONE',  ( -39.00000000000000000, -113.9929510916434339, 12.26648026267477221 ) ) ;
#28453=CARTESIAN_POINT ( 'NONE',  ( -37.51022648969539119, -113.9929510916434339, 14.11852173794918563 ) ) ;
#28456=CARTESIAN_POINT ( 'NONE',  ( -35.50000000000000711, -114.9929510916434339, 12.17846912687782712 ) ) ;
#28462=CARTESIAN_POINT ( 'NONE',  ( -35.95915003344517658, -114.9929510916434339, 13.11692036158763308 ) ) ;
#28470=CARTESIAN_POINT ( 'NONE',  ( -35.50000000000000000, -113.3474311500483935, -0.6247823525984269599 ) ) ;
#28472=CARTESIAN_POINT ( 'NONE',  ( -38.99999999999999289, -113.9407375970686900, 5.253524454178449155 ) ) ;
#28474=CARTESIAN_POINT ( 'NONE',  ( -37.76916472181487450, -111.9754527089670404, 4.034774454178449155 ) ) ;
#28478=CARTESIAN_POINT ( 'NONE',  ( -35.50000000000000711, -113.0974311500471714, -1.624782352598427959 ) ) ;
#28485=CARTESIAN_POINT ( 'NONE',  ( -34.50000000000000000, -115.9630435732166518, -0.9469505670456015434 ) ) ;
#28495=CARTESIAN_POINT ( 'NONE',  ( -37.42187499999996447, -113.9929510916434339, 13.11852480586264846 ) ) ;
#28498=CARTESIAN_POINT ( 'NONE',  ( -35.50040135968784938, -113.9929510916434339, 12.63896776382214071 ) ) ;
#28499=CARTESIAN_POINT ( 'NONE',  ( -35.50000000000000000, -115.9929510916434481, 12.17846912687782712 ) ) ;
#28521=CARTESIAN_POINT ( 'NONE',  ( -34.50000000000000000, -117.0140978167138854, -0.4685323525984310122 ) ) ;
#28525=CARTESIAN_POINT ( 'NONE',  ( -36.33479806579560289, -113.2509883718313262, 9.808975545821553510 ) ) ;
#28531=CARTESIAN_POINT ( 'NONE',  ( -34.50000000000000000, -113.0140978167142833, 0.8752176474015604946 ) ) ;
#28533=CARTESIAN_POINT ( 'NONE',  ( -35.50000000000000711, -113.4307644833805000, -1.624782352598427959 ) ) ;
#28536=CARTESIAN_POINT ( 'NONE',  ( -36.24999999999983658, -114.9929510916434339, 13.11852480586264669 ) ) ;
#28541=CARTESIAN_POINT ( 'NONE',  ( -34.50000000000000000, -114.1489256397697289, 9.518467544735724317 ) ) ;
#28547=CARTESIAN_POINT ( 'NONE',  ( -35.50000000000000000, -114.1835524127412924, 8.514811007161055656 ) ) ;
#28548=CARTESIAN_POINT ( 'NONE',  ( -35.50000000000000711, -112.0154707866092707, 0.9357013553229778235 ) ) ;
#28559=CARTESIAN_POINT ( 'NONE',  ( -37.05926240293131713, -113.0000000000000000, 9.621475545821549957 ) ) ;
#28569=CARTESIAN_POINT ( 'NONE',  ( -34.02454729103297382, -112.6980969099494132, 8.402725545821549957 ) ) ;
#28587=CARTESIAN_POINT ( 'NONE',  ( -34.50000000000000000, -113.0140978167139991, -0.6247823525984269599 ) ) ;
#28590=CARTESIAN_POINT ( 'NONE',  ( -34.50000000000000000, -115.9874658933321001, 10.35517832894335832 ) ) ;
#28594=CARTESIAN_POINT ( 'NONE',  ( -39.00000000000000711, -114.9929510916434339, 12.50851088611646311 ) ) ;
#28605=CARTESIAN_POINT ( 'NONE',  ( -34.02454729103297382, -112.6980969099494132, 3.902725545821552178 ) ) ;
#28608=CARTESIAN_POINT ( 'NONE',  ( -35.50000000000000000, -113.0140978167138712, -0.3747823525984258497 ) ) ;
#28622=CARTESIAN_POINT ( 'NONE',  ( -36.23083527818513261, -111.9754527089670404, 3.715225545821551290 ) ) ;
#28629=CARTESIAN_POINT ( 'NONE',  ( -35.50000000000000000, -113.3474311500483935, -2.624782352598442614 ) ) ;
#28634=CARTESIAN_POINT ( 'NONE',  ( -37.89983305244309975, -114.9929510916434339, 12.92579853460519246 ) ) ;
#28635=CARTESIAN_POINT ( 'NONE',  ( -39.00000000000000000, -113.9929510916434339, 10.85830208992306822 ) ) ;
#28638=CARTESIAN_POINT ( 'NONE',  ( -36.01562499999997158, -113.9929510916434339, 14.11852480586265024 ) ) ;
#28641=CARTESIAN_POINT ( 'NONE',  ( -37.18750000000006395, -114.9929510916434339, 13.11852480586264669 ) ) ;
#28648=CARTESIAN_POINT ( 'NONE',  ( -35.50000000000000711, -114.9929510916434339, 12.39849696637031506 ) ) ;
#28651=CARTESIAN_POINT ( 'NONE',  ( -35.00000000000000000, -114.0592624029313242, 1.503524454178448710 ) ) ;
#28657=CARTESIAN_POINT ( 'NONE',  ( -34.50000000000000000, -113.1061333991432321, 0.8862035858144284850 ) ) ;
#28664=CARTESIAN_POINT ( 'NONE',  ( -36.23083527818512550, -116.0245472910329880, 4.784774454178448266 ) ) ;
#28666=CARTESIAN_POINT ( 'NONE',  ( -35.50000000000000711, -115.5178116849130276, -1.498529437126731034 ) ) ;
#28674=CARTESIAN_POINT ( 'NONE',  ( -34.50000000000000000, -113.6974040292745656, 2.970979214817929481 ) ) ;
#28675=CARTESIAN_POINT ( 'NONE',  ( -35.50000000000000711, -112.9415908020655195, 1.873661708251232572 ) ) ;
#28682=CARTESIAN_POINT ( 'NONE',  ( -37.54084996655477369, -113.9929510916434339, 13.11692036158760466 ) ) ;
#28684=CARTESIAN_POINT ( 'NONE',  ( -35.93473953453761993, -113.9929510916434339, 13.11451721564123396 ) ) ;
#28686=CARTESIAN_POINT ( 'NONE',  ( -35.50000000000000000, -115.6492853190479337, 9.359470924297957239 ) ) ;
#28696=CARTESIAN_POINT ( 'NONE',  ( -35.50000000000000711, -112.9415908020655195, 1.873661708251232572 ) ) ;
#28706=CARTESIAN_POINT ( 'NONE',  ( -34.50000000000000000, -112.9650106922503170, -2.624765990393421955 ) ) ;
#28710=CARTESIAN_POINT ( 'NONE',  ( -35.97545270896702618, -113.6450488405582604, 2.909774454178449155 ) ) ;
#28714=CARTESIAN_POINT ( 'NONE',  ( -34.50000000000000000, -113.2441867727860227, 0.9026824934337903672 ) ) ;
#28717=CARTESIAN_POINT ( 'NONE',  ( -35.74814306589956914, -114.9929510916434339, 13.05539834812772781 ) ) ;
#28722=CARTESIAN_POINT ( 'NONE',  ( -37.34375000000001421, -114.9929510916434339, 14.11852480586264846 ) ) ;
#28730=CARTESIAN_POINT ( 'NONE',  ( -35.50000000000000000, -115.9895221797699065, 10.38535157366622563 ) ) ;
#28731=CARTESIAN_POINT ( 'NONE',  ( -35.50000000000000711, -116.0140978167138712, -0.4685323525984310677 ) ) ;
#28740=CARTESIAN_POINT ( 'NONE',  ( -35.99999999999999289, -113.9407375970686758, 6.996475545821551734 ) ) ;
#28747=CARTESIAN_POINT ( 'NONE',  ( -35.69809690994941320, -116.9754527089670546, 5.777725545821551734 ) ) ;
#28763=CARTESIAN_POINT ( 'NONE',  ( -34.50000000000000000, -113.1807644833805426, -0.6247823525984269599 ) ) ;
#28767=CARTESIAN_POINT ( 'NONE',  ( -37.37500000000009237, -115.9929510916434481, 14.11852480586265024 ) ) ;
#28770=CARTESIAN_POINT ( 'NONE',  ( -39.00000000000000711, -114.9929510916434339, 12.39849696637031151 ) ) ;
#28781=CARTESIAN_POINT ( 'NONE',  ( -38.30190309005061522, -111.0245472910330022, 6.527725545821552622 ) ) ;
#28783=CARTESIAN_POINT ( 'NONE',  ( -35.50000000000000000, -113.0140978167137717, -0.6411448143358797758 ) ) ;
#28793=CARTESIAN_POINT ( 'NONE',  ( -37.76916472181486739, -116.0245472910329880, 4.465225545821550845 ) ) ;
#28799=CARTESIAN_POINT ( 'NONE',  ( -35.50000000000000000, -114.9307644833806137, -2.624782352598442614 ) ) ;
#28805=CARTESIAN_POINT ( 'NONE',  ( -37.99359134332094357, -114.9929510916434339, 12.69998175888958158 ) ) ;
#28807=CARTESIAN_POINT ( 'NONE',  ( -34.50000000000000000, -114.1264797827112574, 9.515205387299289441 ) ) ;
#28811=CARTESIAN_POINT ( 'NONE',  ( -38.25557080230232998, -113.9929510916434339, 13.92914543265419525 ) ) ;
#28813=CARTESIAN_POINT ( 'NONE',  ( -35.50000000000000711, -114.9929510916434339, 12.60752341388803544 ) ) ;
#28819=CARTESIAN_POINT ( 'NONE',  ( -35.50005019975638021, -114.9929510916434339, 12.62670525340498529 ) ) ;
#28827=CARTESIAN_POINT ( 'NONE',  ( -34.50000000000000000, -113.0140978167138712, 0.6252176474015680441 ) ) ;
#28829=CARTESIAN_POINT ( 'NONE',  ( -35.00000000000000000, -114.0592624029313242, 7.503524454178449155 ) ) ;
#28833=CARTESIAN_POINT ( 'NONE',  ( -37.05926240293131713, -115.9999999999999858, 6.378524454178448266 ) ) ;
#28835=CARTESIAN_POINT ( 'NONE',  ( -35.50000000000000711, -112.0140978167138712, 0.0002176474015661141945 ) ) ;
#28843=CARTESIAN_POINT ( 'NONE',  ( -34.50000000000000000, -116.0140978167138712, 0.0002176474015577116276 ) ) ;
#28844=CARTESIAN_POINT ( 'NONE',  ( -35.50000000000000711, -113.0106174888879877, 1.881901162060937827 ) ) ;
#28850=CARTESIAN_POINT ( 'NONE',  ( -36.03125000000003553, -113.9929510916434339, 13.11852480586264846 ) ) ;
#28855=CARTESIAN_POINT ( 'NONE',  ( -36.50000000000010658, -113.9929510916434339, 13.11852480586264846 ) ) ;
#28856=CARTESIAN_POINT ( 'NONE',  ( -35.52552712174883709, -115.9929510916434481, 12.77960891308624625 ) ) ;
#28868=CARTESIAN_POINT ( 'NONE',  ( -35.50000000000000711, -112.0141059978162019, -0.6575071456984691309 ) ) ;
#28875=CARTESIAN_POINT ( 'NONE',  ( -34.50000000000000000, -115.5324766040685631, -2.560864217809699195 ) ) ;
#28879=CARTESIAN_POINT ( 'NONE',  ( -37.47347596530441649, -113.0245472910329880, 9.527725545821551734 ) ) ;
#28886=CARTESIAN_POINT ( 'NONE',  ( -35.50000000000000000, -114.8474311500471572, -0.6247823525984269599 ) ) ;
#28891=CARTESIAN_POINT ( 'NONE',  ( -35.50000000000000711, -114.9929510916434339, 12.57451923796416082 ) ) ;
#28895=CARTESIAN_POINT ( 'NONE',  ( -37.52454134262690388, -114.9929510916434339, 14.11837420659362152 ) ) ;
#28901=CARTESIAN_POINT ( 'NONE',  ( -35.50000000000000000, -115.9929510916434481, 11.38636890470581164 ) ) ;
#28903=CARTESIAN_POINT ( 'NONE',  ( -35.50000000000000711, -113.8474311500459777, -1.624782352598427959 ) ) ;
#28913=CARTESIAN_POINT ( 'NONE',  ( -35.97545270896705460, -114.3549511594417680, 5.590225545821552622 ) ) ;
#28923=CARTESIAN_POINT ( 'NONE',  ( -34.00000000000000000, -113.9407375970686758, 9.996475545821549957 ) ) ;
#28944=CARTESIAN_POINT ( 'NONE',  ( -35.07817881376918479, -115.9929510916434481, 13.81802396319203474 ) ) ;
#28945=DIRECTION ( 'NONE',  ( 0.000000000000000000, 0.9929510916431029122, -0.1185248058626136303 ) ) ;
#28947=CARTESIAN_POINT ( 'NONE',  ( -34.57658136524561598, -115.9929510916434481, 13.10177712753338675 ) ) ;
#28958=CARTESIAN_POINT ( 'NONE',  ( -34.83677480945821259, -116.0794154965774965, 5.683975545821551734 ) ) ;
#28960=CARTESIAN_POINT ( 'NONE',  ( -35.50000000000000000, -113.0140978167138996, -0.6247823525984306237 ) ) ;
#28971=CARTESIAN_POINT ( 'NONE',  ( -37.88768952767750875, -112.0245472910329880, 3.527725545821551290 ) ) ;
#28976=CARTESIAN_POINT ( 'NONE',  ( -35.50000000000000000, -112.6882700046066645, -2.599147725882136939 ) ) ;
#28982=CARTESIAN_POINT ( 'NONE',  ( -38.00000000000000711, -114.9929510916434339, 11.73841344789285657 ) ) ;
#28983=CARTESIAN_POINT ( 'NONE',  ( -34.50000000000000000, -114.9929510916434339, 10.56126450660895699 ) ) ;
#28985=CARTESIAN_POINT ( 'NONE',  ( -36.24999999999983658, -114.9929510916434339, 13.11852480586264669 ) ) ;
#28987=CARTESIAN_POINT ( 'NONE',  ( -35.95093014754292682, -113.9929510916434339, 14.11777216781842625 ) ) ;
#28995=CARTESIAN_POINT ( 'NONE',  ( -35.50000000000000711, -114.9929510916434339, 11.91443571948719971 ) ) ;
#29003=CARTESIAN_POINT ( 'NONE',  ( -34.50000000000000000, -113.0140978167139991, 0.8595926474015699315 ) ) ;
#29007=CARTESIAN_POINT ( 'NONE',  ( -37.76916472181487450, -111.9754527089670404, 7.034774454178450931 ) ) ;
#29010=CARTESIAN_POINT ( 'NONE',  ( -35.50000000000000711, -116.0012805033554883, -0.7876962586524312027 ) ) ;
#29019=CARTESIAN_POINT ( 'NONE',  ( -34.50000000000000000, -113.1451905347060460, 2.905063584339864668 ) ) ;
#29020=CARTESIAN_POINT ( 'NONE',  ( -35.50000000000000711, -113.6318576702834804, 1.956056246348823580 ) ) ;
#29027=CIRCLE ( 'NONE', #23842, 0.5000000000000004441 ) ;
#29028=CARTESIAN_POINT ( 'NONE',  ( -38.00000000000000711, -113.9929510916434339, 12.26648026267477221 ) ) ;
#29031=CARTESIAN_POINT ( 'NONE',  ( -35.50000000000000000, -113.9929510916434339, 10.94631322572069365 ) ) ;
#29033=CARTESIAN_POINT ( 'NONE',  ( -35.74814306589956203, -115.9929510916434481, 13.05539834812772781 ) ) ;
#29044=CARTESIAN_POINT ( 'NONE',  ( -35.50000000000000711, -114.8057644833805568, -1.624782352598427959 ) ) ;
#29054=CARTESIAN_POINT ( 'NONE',  ( -35.50000000000000000, -113.2372261171341563, 2.916049522752222511 ) ) ;
#29059=CARTESIAN_POINT ( 'NONE',  ( -37.47347596530441649, -114.9754527089670262, 4.972274454178449155 ) ) ;
#29064=CARTESIAN_POINT ( 'NONE',  ( -35.50000000000000000, -115.0140978167138712, -0.4997823525984417259 ) ) ;
#29071=CARTESIAN_POINT ( 'NONE',  ( -35.50000000000000711, -114.9929510916434339, 10.55026311463432087 ) ) ;
#29073=CARTESIAN_POINT ( 'NONE',  ( -35.97545865737298953, -114.9929510916434339, 14.11837420659365705 ) ) ;
#29079=CARTESIAN_POINT ( 'NONE',  ( -35.91854304697312728, -115.9929510916434481, 13.11211614918345703 ) ) ;
#29080=CARTESIAN_POINT ( 'NONE',  ( -35.50000000000000711, -116.0140978167138712, -0.4997823525984418369 ) ) ;
#29095=CARTESIAN_POINT ( 'NONE',  ( -36.64504884055823908, -115.0245472910329880, 6.284774454178449155 ) ) ;
#29105=CARTESIAN_POINT ( 'NONE',  ( -34.00000000000000000, -113.9407375970686758, 8.496475545821549957 ) ) ;
#29125=PLANE ( 'NONE',  #19944 ) ;
#29127=CARTESIAN_POINT ( 'NONE',  ( -37.46093750000000711, -115.9929510916434481, 14.11852480586265024 ) ) ;
#29129=CARTESIAN_POINT ( 'NONE',  ( -37.88768952767750164, -115.9754527089670262, 4.972274454178449155 ) ) ;
#29130=CARTESIAN_POINT ( 'NONE',  ( -34.50015059926905536, -115.9929510916434481, 12.64306614848962518 ) ) ;
#29142=CARTESIAN_POINT ( 'NONE',  ( -39.02454729103295961, -113.2308352781851539, 4.840225545821551734 ) ) ;
#29146=CARTESIAN_POINT ( 'NONE',  ( -35.50000000000000000, -113.1291422947505936, 0.8889500704178361357 ) ) ;
#29166=CARTESIAN_POINT ( 'NONE',  ( -35.50000000000000711, -112.0651520602111191, -0.9469505670458575608 ) ) ;
#29175=CARTESIAN_POINT ( 'NONE',  ( -34.50000000000000000, -114.9929510916434339, 12.53051367006571581 ) ) ;
#29179=CARTESIAN_POINT ( 'NONE',  ( -35.98364338251434447, -114.9929510916434339, 13.11827392651456314 ) ) ;
#29181=CARTESIAN_POINT ( 'NONE',  ( -34.50000000000000000, -114.1861579685891712, 9.524983039397698192 ) ) ;
#29184=CARTESIAN_POINT ( 'NONE',  ( -37.99899697755054717, -114.9929510916434339, 12.65121853911336736 ) ) ;
#29191=CARTESIAN_POINT ( 'NONE',  ( -35.98364338251434447, -114.9929510916434339, 13.11827392651456314 ) ) ;
#29200=CARTESIAN_POINT ( 'NONE',  ( -34.50000000000000000, -113.0140978167138712, 0.3752176474015639918 ) ) ;
#29204=CARTESIAN_POINT ( 'NONE',  ( -40.02454729103296671, -115.1833782841879525, 2.159774454178448710 ) ) ;
#29208=CARTESIAN_POINT ( 'NONE',  ( -35.50000000000000711, -116.0140978167138712, -0.4685323525984310677 ) ) ;
#29215=CARTESIAN_POINT ( 'NONE',  ( -34.50000000000000000, -112.9813730236132585, -1.624774171495860786 ) ) ;
#29221=CARTESIAN_POINT ( 'NONE',  ( -34.50000000000000000, -113.9929510916434339, 10.50625754673586876 ) ) ;
#29223=CARTESIAN_POINT ( 'NONE',  ( -38.00000000000000711, -113.9929510916434339, 11.73841344789285657 ) ) ;
#29226=CARTESIAN_POINT ( 'NONE',  ( -35.97955704204053262, -115.9929510916434481, 13.11812344617474402 ) ) ;
#29237=CARTESIAN_POINT ( 'NONE',  ( -35.50000000000000711, -112.0140978167138712, 0.6252176474015680441 ) ) ;
#29244=CARTESIAN_POINT ( 'NONE',  ( -34.50000000000000000, -116.7615919857705080, -1.632210089000343700 ) ) ;
#29248=CARTESIAN_POINT ( 'NONE',  ( -36.02454729103298092, -114.4734759653044307, 3.097274454178448710 ) ) ;
#29254=CARTESIAN_POINT ( 'NONE',  ( -35.50000000000000000, -115.0140978167138712, -0.6247823525984408377 ) ) ;
#29258=CARTESIAN_POINT ( 'NONE',  ( -38.00000068757622529, -114.9929510916434339, 12.61439929482944855 ) ) ;
#29260=CARTESIAN_POINT ( 'NONE',  ( -34.50000000000000000, -114.9929510916434339, 12.57451923796416082 ) ) ;
#29266=CARTESIAN_POINT ( 'NONE',  ( -36.31249999999994316, -115.9929510916434481, 13.11852480586264846 ) ) ;
#29267=CARTESIAN_POINT ( 'NONE',  ( -35.50000000000000711, -114.3474311500471430, -1.624782352598427959 ) ) ;
#29279=CARTESIAN_POINT ( 'NONE',  ( -37.05926240293133134, -115.0000000000000000, 4.878524454178448266 ) ) ;
#29282=ADVANCED_FACE ( 'NONE', ( #31030 ), #23872, .F. ) ;
#29288=CARTESIAN_POINT ( 'NONE',  ( -38.30190309005061522, -111.0245472910330022, 6.527725545821552622 ) ) ;
#29306=CARTESIAN_POINT ( 'NONE',  ( -35.98977351030467986, -115.9929510916434481, 14.11852173794918563 ) ) ;
#29310=CARTESIAN_POINT ( 'NONE',  ( -35.62769128460905677, -115.4561184093552413, 7.691024454178449155 ) ) ;
#29312=CARTESIAN_POINT ( 'NONE',  ( -34.50000000000000000, -115.9929510916434481, 12.39849696637031684 ) ) ;
#29321=CARTESIAN_POINT ( 'NONE',  ( -35.81662171581203324, -110.9754527089670546, 8.215225545821551734 ) ) ;
#29323=CARTESIAN_POINT ( 'NONE',  ( -35.50000000000000000, -113.0256022645180707, 0.8765908897032291813 ) ) ;
#29342=CARTESIAN_POINT ( 'NONE',  ( -35.50000000000000711, -113.8159288351371714, 1.978028123174813802 ) ) ;
#29351=CARTESIAN_POINT ( 'NONE',  ( -34.50000000000000000, -114.9929501463477663, 10.50247632894551231 ) ) ;
#29354=CARTESIAN_POINT ( 'NONE',  ( -36.03906250000000000, -114.9929510916434339, 13.11852480586264669 ) ) ;
#29359=CARTESIAN_POINT ( 'NONE',  ( -34.50000000000000000, -114.0743172650041686, 9.508870970061893857 ) ) ;
#29362=( LENGTH_UNIT ( ) NAMED_UNIT ( * ) SI_UNIT ( .MILLI., .METRE. ) );
#29367=CARTESIAN_POINT ( 'NONE',  ( -37.54084996655477369, -114.9929510916434339, 13.11692036158760466 ) ) ;
#29369=CARTESIAN_POINT ( 'NONE',  ( -38.97545270896704039, -113.1123104723225197, 6.847274454178450931 ) ) ;
#29376=CARTESIAN_POINT ( 'NONE',  ( -37.76916472181487450, -111.9754527089670404, 8.534774454178448266 ) ) ;
#29390=CARTESIAN_POINT ( 'NONE',  ( -34.50000000000000000, -111.0140978167138570, 0.7189676474015717078 ) ) ;
#29396=CARTESIAN_POINT ( 'NONE',  ( -35.50000000000000711, -114.1091535596544873, 9.513028657562415447 ) ) ;
#29397=CARTESIAN_POINT ( 'NONE',  ( -34.50000000000000000, -113.9948283797722439, 10.50648163149984171 ) ) ;
#29400=CARTESIAN_POINT ( 'NONE',  ( -37.50818044754229419, -113.9929510916434339, 13.11847460610629845 ) ) ;
#29401=CARTESIAN_POINT ( 'NONE',  ( -37.56526046546249376, -115.9929510916434481, 13.11451721564129258 ) ) ;
#29411=CARTESIAN_POINT ( 'NONE',  ( -35.50000000000000711, -114.9307644833806137, -1.624782352598427959 ) ) ;
#29417=CARTESIAN_POINT ( 'NONE',  ( -35.50000000000000000, -113.0974311500471714, -2.624782352598442614 ) ) ;
#29421=CARTESIAN_POINT ( 'NONE',  ( -37.05926240293133134, -115.0000000000000000, 7.878524454178450043 ) ) ;
#29425=CARTESIAN_POINT ( 'NONE',  ( -34.50000000000000000, -113.0140978167138712, 0.8752176474015934682 ) ) ;
#29431=CARTESIAN_POINT ( 'NONE',  ( -35.50000000000000000, -113.9929510916434623, 10.50625754673586876 ) ) ;
#29435=CARTESIAN_POINT ( 'NONE',  ( -34.50000000000000000, -112.1403507321855528, -1.128496220798856253 ) ) ;
#29436=CARTESIAN_POINT ( 'NONE',  ( -35.93867112612154813, -114.9929510916434339, 14.11732072679899197 ) ) ;
#29441=CARTESIAN_POINT ( 'NONE',  ( -36.00585935943765747, -115.9929510916434481, 13.11852578240983291 ) ) ;
#29442=CARTESIAN_POINT ( 'NONE',  ( -35.50000000000000711, -115.0795240838853886, -1.623175561345890472 ) ) ;
#29453=CARTESIAN_POINT ( 'NONE',  ( -35.99999999999999289, -114.0592624029313242, 7.503524454178450043 ) ) ;
#29464=CARTESIAN_POINT ( 'NONE',  ( -37.05926240293131713, -112.0000000000000142, 9.621475545821551734 ) ) ;
#29487=CARTESIAN_POINT ( 'NONE',  ( -38.45611840935523418, -115.3723087153909432, 8.066024454178448266 ) ) ;
#29488=CARTESIAN_POINT ( 'NONE',  ( -34.50000000000000000, -115.9929510916434481, 11.91443571948720148 ) ) ;
#29497=CARTESIAN_POINT ( 'NONE',  ( -36.94073759706868287, -115.9999999999999858, 5.871475545821550845 ) ) ;
#29513=EDGE_CURVE ( 'NONE', #18380, #18157, #17109, .T. ) ;
#29514=CARTESIAN_POINT ( 'NONE',  ( -37.88768952767750875, -112.0245472910329880, 9.527725545821553510 ) ) ;
#29521=CARTESIAN_POINT ( 'NONE',  ( -35.50000000000000711, -112.8655373925166572, 1.864575885149403423 ) ) ;
#29529=CARTESIAN_POINT ( 'NONE',  ( -34.50000000000000000, -113.8159288351371714, 1.978028123174813802 ) ) ;
#29530=CARTESIAN_POINT ( 'NONE',  ( -34.50300906734827322, -114.9929510916434339, 12.71660600561482468 ) ) ;
#29533=CARTESIAN_POINT ( 'NONE',  ( -37.97447287825094975, -114.9929510916434339, 12.77960891308616809 ) ) ;
#29536=CARTESIAN_POINT ( 'NONE',  ( -34.50000000000000000, -114.2305202833893816, 9.534416457224700991 ) ) ;
#29538=CARTESIAN_POINT ( 'NONE',  ( -38.00000000000000711, -114.9929510916434339, 11.73841344789285657 ) ) ;
#29539=CARTESIAN_POINT ( 'NONE',  ( -35.00000000000000000, -114.0000000000000853, 2.000000000000001776 ) ) ;
#29544=CARTESIAN_POINT ( 'NONE',  ( -37.42187499999997158, -114.9929510916434339, 13.11852480586264669 ) ) ;
#29546=CARTESIAN_POINT ( 'NONE',  ( -35.81662171581204746, -117.0245472910329738, 1.784774454178449155 ) ) ;
#29556=CARTESIAN_POINT ( 'NONE',  ( -35.69809690994938478, -111.0245472910330022, 2.722274454178449155 ) ) ;
#29569=CARTESIAN_POINT ( 'NONE',  ( -34.50000000000000000, -112.8115600290184801, 2.865251044451027074 ) ) ;
#29573=CARTESIAN_POINT ( 'NONE',  ( -35.50000000000000711, -114.9912366357066986, 10.44580456020104720 ) ) ;
#29575=CARTESIAN_POINT ( 'NONE',  ( -34.50000000000000000, -113.9929510916434339, 10.50763272073269405 ) ) ;
#29578=CARTESIAN_POINT ( 'NONE',  ( -38.00000000000000711, -113.9929510916434339, 12.44250253426875119 ) ) ;
#29579=CARTESIAN_POINT ( 'NONE',  ( -35.93473953453761993, -115.9929510916434481, 13.11451721564123396 ) ) ;
#29591=CARTESIAN_POINT ( 'NONE',  ( -35.50000000000000711, -113.0557643173828524, -1.624792769101735868 ) ) ;
#29593=CARTESIAN_POINT ( 'NONE',  ( -35.50100302244946704, -114.9929510916434339, 12.65121853911337269 ) ) ;
#29597=CARTESIAN_POINT ( 'NONE',  ( -35.50000000000000000, -112.8832452823708792, -2.621568770093253953 ) ) ;
#29601=CARTESIAN_POINT ( 'NONE',  ( -35.99999999999999289, -114.0592624029313242, 9.003524454178446490 ) ) ;
#29606=CARTESIAN_POINT ( 'NONE',  ( -34.50000000000000000, -114.3474311500471572, -0.6247823525984269599 ) ) ;
#29612=CARTESIAN_POINT ( 'NONE',  ( -37.37500000000009237, -114.9929510916434339, 13.11852480586264669 ) ) ;
#29615=CARTESIAN_POINT ( 'NONE',  ( -34.50000000000000000, -113.2224311500466030, -1.624782352598427959 ) ) ;
#29620=CARTESIAN_POINT ( 'NONE',  ( -37.46874999999995737, -115.9929510916434481, 13.11852480586264846 ) ) ;
#29642=CARTESIAN_POINT ( 'NONE',  ( -37.88768952767750875, -112.0245472910329880, 6.527725545821550845 ) ) ;
#29645=ORIENTED_EDGE ( 'NONE', *, *, #15666, .F. ) ;
#29657=CARTESIAN_POINT ( 'NONE',  ( -38.45611840935523418, -115.3723087153909432, 6.566024454178448266 ) ) ;
#29658=CARTESIAN_POINT ( 'NONE',  ( -34.50000000000000000, -115.9926080209513657, 10.46845107750242398 ) ) ;
#29668=CARTESIAN_POINT ( 'NONE',  ( -40.02454729103296671, -112.8166217158120332, 9.340225545821551734 ) ) ;
#29689=CARTESIAN_POINT ( 'NONE',  ( -35.50000000000000711, -112.0250551866464548, 1.025914454044489332 ) ) ;
#29696=CARTESIAN_POINT ( 'NONE',  ( -34.50000000000000000, -112.0140978167138712, -0.4685323525984295134 ) ) ;
#29697=CARTESIAN_POINT ( 'NONE',  ( -34.50000000000000000, -114.9929510916434339, 10.59426868253284226 ) ) ;
#29700=CARTESIAN_POINT ( 'NONE',  ( -35.50000000000000000, -113.9929510916435049, 10.50625754673586876 ) ) ;
#29702=CARTESIAN_POINT ( 'NONE',  ( -39.00000000000000000, -113.9929510916434339, 12.39849696637031151 ) ) ;
#29715=CARTESIAN_POINT ( 'NONE',  ( -38.00000000000000711, -114.9929510916434339, 12.53051367006571937 ) ) ;
#29718=CARTESIAN_POINT ( 'NONE',  ( -37.76916472181487450, -111.9754527089670404, 5.534774454178449155 ) ) ;
#29727=CARTESIAN_POINT ( 'NONE',  ( -35.69809690994938478, -111.0245472910330022, 4.222274454178449155 ) ) ;
#29740=CARTESIAN_POINT ( 'NONE',  ( -34.50000000000000000, -111.0687598768285369, 1.355111303971038073 ) ) ;
#29746=CARTESIAN_POINT ( 'NONE',  ( -35.50000000000000711, -114.9927795562974069, 10.48735431211914815 ) ) ;
#29748=CARTESIAN_POINT ( 'NONE',  ( -34.50000000000000000, -113.9929510916434339, 10.59426868253284226 ) ) ;
#29749=CARTESIAN_POINT ( 'NONE',  ( -34.50000000000000000, -116.0140978167138712, 0.8752176474015622709 ) ) ;
#29751=CARTESIAN_POINT ( 'NONE',  ( -34.50000000000000000, -113.9929510916434339, 10.50625754673586876 ) ) ;
#29752=CARTESIAN_POINT ( 'NONE',  ( -37.54084996655477369, -115.9929510916434481, 13.11692036158760466 ) ) ;
#29768=CARTESIAN_POINT ( 'NONE',  ( -35.50000000000000000, -113.0140978167138712, -0.1247823525984260717 ) ) ;
#29772=CARTESIAN_POINT ( 'NONE',  ( -35.50000000000000711, -114.9928438774171582, 10.49113435197128652 ) ) ;
#29777=CARTESIAN_POINT ( 'NONE',  ( -35.50000000000000000, -112.8690837874180062, 2.872105769100646189 ) ) ;
#29780=CARTESIAN_POINT ( 'NONE',  ( -35.97545270896702618, -113.6450488405582604, 5.909774454178450931 ) ) ;
#29786=CARTESIAN_POINT ( 'NONE',  ( -34.50000000000000000, -113.0140978167138712, -0.6247823525979733228 ) ) ;
#29795=CARTESIAN_POINT ( 'NONE',  ( -35.50000000000000000, -113.9697269463297431, 10.50348536859153370 ) ) ;
#29799=CARTESIAN_POINT ( 'NONE',  ( -34.50000000000000000, -112.0221129971568104, -0.7553032835231431319 ) ) ;
#29804=CARTESIAN_POINT ( 'NONE',  ( -37.54084996655477369, -115.9929510916434481, 13.11692036158760466 ) ) ;
#29826=CARTESIAN_POINT ( 'NONE',  ( -35.00000000000000000, -113.9407375970686900, 8.496475545821551734 ) ) ;
#29845=CARTESIAN_POINT ( 'NONE',  ( -34.97545270896703329, -113.2308352781851397, 4.409774454178448266 ) ) ;
#29846=CARTESIAN_POINT ( 'NONE',  ( -37.56132887387857267, -115.9929510916434481, 14.11732072679899197 ) ) ;
#29854=CARTESIAN_POINT ( 'NONE',  ( -37.88768952767750875, -112.0245472910329880, 3.527725545821551290 ) ) ;
#29859=CARTESIAN_POINT ( 'NONE',  ( -34.50000000000000000, -113.1291422947505936, 0.8889500704178361357 ) ) ;
#29872=CARTESIAN_POINT ( 'NONE',  ( -35.50000000000000711, -112.0140978167138712, 0.3752176474015640473 ) ) ;
#29878=CARTESIAN_POINT ( 'NONE',  ( -34.50000000000000000, -116.0140978167138712, -0.5622823525984409487 ) ) ;
#29879=CARTESIAN_POINT ( 'NONE',  ( -38.42182118622945808, -114.9929510916434339, 13.81802396319329773 ) ) ;
#29881=CARTESIAN_POINT ( 'NONE',  ( -35.50000000000000000, -113.9929510916434623, 10.50625754673586876 ) ) ;
#29884=CARTESIAN_POINT ( 'NONE',  ( -39.00000000000000000, -113.9929510916434339, 12.44250253426875119 ) ) ;
#29893=CARTESIAN_POINT ( 'NONE',  ( -37.46874999999996447, -114.9929510916434339, 13.11852480586264669 ) ) ;
#29897=CARTESIAN_POINT ( 'NONE',  ( -36.11231047232249125, -112.0245472910329880, 4.222274454178449155 ) ) ;
#29905=CARTESIAN_POINT ( 'NONE',  ( -39.07941549657749647, -116.1632251905417803, 3.058975545821551734 ) ) ;
#29916=CARTESIAN_POINT ( 'NONE',  ( -34.50000000000000000, -111.2666036476567655, -1.632210088999287212 ) ) ;
#29923=CARTESIAN_POINT ( 'NONE',  ( -35.50000000000000711, -114.9929510916434339, 10.55026311463432087 ) ) ;
#29924=CARTESIAN_POINT ( 'NONE',  ( -35.24442919769867899, -113.9929510916434339, 13.92914543265605509 ) ) ;
#29928=CARTESIAN_POINT ( 'NONE',  ( -37.49414064056232831, -113.9929510916434339, 13.11852578240983291 ) ) ;
#29929=CARTESIAN_POINT ( 'NONE',  ( -38.00000000000000711, -115.9929510916434481, 12.57451923796417681 ) ) ;
#29941=CARTESIAN_POINT ( 'NONE',  ( -35.50000000000000000, -114.1185248058627053, 1.007048908356900085 ) ) ;
#29945=CARTESIAN_POINT ( 'NONE',  ( -35.50000000000000711, -114.9929510916434339, 12.39849696637031506 ) ) ;
#29950=CARTESIAN_POINT ( 'NONE',  ( -35.50000000000000000, -111.2666036476567655, -1.632210088999287212 ) ) ;
#29953=CARTESIAN_POINT ( 'NONE',  ( -37.35495115944176092, -112.9754527089670688, 5.534774454178449155 ) ) ;
#29958=CARTESIAN_POINT ( 'NONE',  ( -34.50000000000000000, -113.0140978167141128, -0.6247823525984907977 ) ) ;
#29965=CARTESIAN_POINT ( 'NONE',  ( -37.58145695302688694, -114.9929510916434339, 13.11211614918362756 ) ) ;
#29971=CARTESIAN_POINT ( 'NONE',  ( -34.50000000000000000, -114.8057644833805568, -1.624782352598427959 ) ) ;
#29974=CARTESIAN_POINT ( 'NONE',  ( -34.50015059926905536, -115.9929510916434481, 12.64306614848962518 ) ) ;
#29978=CARTESIAN_POINT ( 'NONE',  ( -37.99959864031216483, -115.9929510916434481, 12.63896776382213538 ) ) ;
#29999=CARTESIAN_POINT ( 'NONE',  ( -35.00000000000000000, -113.9407375970686900, 5.496475545821551734 ) ) ;
#30020=CARTESIAN_POINT ( 'NONE',  ( -35.93867112612154102, -115.9929510916434481, 14.11732072679899197 ) ) ;
#30029=CARTESIAN_POINT ( 'NONE',  ( -38.45611840935523418, -112.6276912846090568, 9.433975545821551734 ) ) ;
#30054=CARTESIAN_POINT ( 'NONE',  ( -34.50000000000000000, -116.0140978167138712, -0.3747823525984422255 ) ) ;
#30055=CARTESIAN_POINT ( 'NONE',  ( -37.42187499999997158, -114.9929510916434339, 14.11852480586264846 ) ) ;
#30057=CARTESIAN_POINT ( 'NONE',  ( -38.00000000000000711, -114.9929510916434339, 12.44250253426874941 ) ) ;
#30059=CARTESIAN_POINT ( 'NONE',  ( -36.07812499999994316, -114.9929510916434339, 14.11852480586264846 ) ) ;
#30070=CARTESIAN_POINT ( 'NONE',  ( -34.97545270896703329, -113.2308352781851539, 5.909774454178449155 ) ) ;
#30078=CARTESIAN_POINT ( 'NONE',  ( -34.83677480945821259, -116.0794154965774965, 2.683975545821551734 ) ) ;
#30090=CARTESIAN_POINT ( 'NONE',  ( -34.50000000000000000, -111.0168437565048691, 0.9961850632443862708 ) ) ;
#30095=CARTESIAN_POINT ( 'NONE',  ( -35.50000000000000711, -114.9929510916434339, 10.53376102667243508 ) ) ;
#30096=CARTESIAN_POINT ( 'NONE',  ( -34.50000000000000000, -113.9929510916434339, 11.73841344789270202 ) ) ;
#30099=CARTESIAN_POINT ( 'NONE',  ( -34.54793860109200665, -113.9929510916434339, 13.00730889637958221 ) ) ;
#30100=CARTESIAN_POINT ( 'NONE',  ( -37.98325232167028531, -114.9929510916434339, 14.04194344061727406 ) ) ;
#30101=CARTESIAN_POINT ( 'NONE',  ( -35.50000000000000711, -114.1414532730574507, 9.517316564499758158 ) ) ;
#30114=CARTESIAN_POINT ( 'NONE',  ( -35.50000000000000711, -116.0140978167138712, 0.8752176474015622709 ) ) ;
#30117=CARTESIAN_POINT ( 'NONE',  ( -36.25098837183129774, -113.3347980657956242, 4.316024454178448266 ) ) ;
#30119=CARTESIAN_POINT ( 'NONE',  ( -35.50005019975638021, -114.9929510916434339, 12.62670525340498529 ) ) ;
#30122=CARTESIAN_POINT ( 'NONE',  ( -35.50000000000000000, -111.0301281775997353, -0.8858242144478579716 ) ) ;
#30125=CARTESIAN_POINT ( 'NONE',  ( -36.02454729103298092, -114.4734759653044307, 7.597274454178449155 ) ) ;
#30131=CARTESIAN_POINT ( 'NONE',  ( -34.50000000000000000, -113.0140978167140702, 0.8752176474015694874 ) ) ;
#30136=CARTESIAN_POINT ( 'NONE',  ( -35.50000000000000000, -113.9929510916434339, 12.56351784598954424 ) ) ;
#30140=CARTESIAN_POINT ( 'NONE',  ( -34.50000000000000000, -113.0557643173828524, -1.624792769101735868 ) ) ;
#30142=CARTESIAN_POINT ( 'NONE',  ( -38.99879592093640213, -115.9929510916434481, 12.67985367974111277 ) ) ;
#30145=ADVANCED_BREP_SHAPE_REPRESENTATION ( '', ( #22365, #21307 ), #12169 ) ;
#30148=CARTESIAN_POINT ( 'NONE',  ( -37.53269373325071712, -115.9929510916434481, 13.11752178341324360 ) ) ;
#30170=CARTESIAN_POINT ( 'NONE',  ( -35.62769128460905677, -112.5438815906447729, 5.308975545821551734 ) ) ;
#30180=CARTESIAN_POINT ( 'NONE',  ( -35.50000000000000711, -114.0000000000003411, 9.500000000000035527 ) ) ;
#30190=CARTESIAN_POINT ( 'NONE',  ( -35.75562914091914024, -115.9929510916434481, 14.09929883582542409 ) ) ;
#30201=CARTESIAN_POINT ( 'NONE',  ( -38.99999999999999289, -114.0592624029313242, 9.246475545821551734 ) ) ;
#30209=DIRECTION ( 'NONE',  ( 0.000000000000000000, -0.9929510916431035783, 0.1185248058626076212 ) ) ;
#30228=CARTESIAN_POINT ( 'NONE',  ( -34.50000000000000000, -113.0974311500471714, -1.624782352598427959 ) ) ;
#30230=CARTESIAN_POINT ( 'NONE',  ( -38.99924736195578134, -114.9929510916434339, 12.66759465831984777 ) ) ;
#30232=CARTESIAN_POINT ( 'NONE',  ( -35.50000000000000000, -113.9929510916434339, 10.50625754673577994 ) ) ;
#30234=CARTESIAN_POINT ( 'NONE',  ( -35.80421860361284558, -114.9929510916434339, 14.10650203519841916 ) ) ;
#30242=CARTESIAN_POINT ( 'NONE',  ( -38.00000000000000711, -114.9929510916434339, 10.85830208992306822 ) ) ;
#30245=CARTESIAN_POINT ( 'NONE',  ( -35.69809690994938478, -111.0245472910330022, 7.222274454178449155 ) ) ;
#30255=CARTESIAN_POINT ( 'NONE',  ( -38.18337828418795965, -110.9754527089670546, 8.534774454178448266 ) ) ;
#30266=CARTESIAN_POINT ( 'NONE',  ( -34.50000000000000000, -117.0140814545088688, -0.6738694770610542673 ) ) ;
#30270=CARTESIAN_POINT ( 'NONE',  ( -36.03125000000004263, -114.9929510916434339, 13.11852480586264669 ) ) ;
#30276=CARTESIAN_POINT ( 'NONE',  ( -34.80050084267116972, -113.9929510916434339, 13.54034599209289347 ) ) ;
#30279=CARTESIAN_POINT ( 'NONE',  ( -34.50000000000000000, -113.9929510916434339, 10.50625754673588474 ) ) ;
#30282=CARTESIAN_POINT ( 'NONE',  ( -35.50000000000000711, -114.9929510916434339, 10.68227981832981044 ) ) ;
#30296=CARTESIAN_POINT ( 'NONE',  ( -35.50000000000000711, -116.0060826362711595, -0.7553032835231661135 ) ) ;
#30298=CARTESIAN_POINT ( 'NONE',  ( -36.33479806579561000, -114.7490116281687165, 4.691024454178447378 ) ) ;
#30303=CARTESIAN_POINT ( 'NONE',  ( -35.50000000000000000, -116.6134300264884445, -1.853877267570539944 ) ) ;
#30307=CARTESIAN_POINT ( 'NONE',  ( -35.54388159064475872, -112.6276912846090568, 4.316024454178448266 ) ) ;
#30313=CARTESIAN_POINT ( 'NONE',  ( -34.50000000000000000, -112.0140978167138712, 0.7189676474015718188 ) ) ;
#30320=CARTESIAN_POINT ( 'NONE',  ( -35.50000000000000000, -113.9929510916434339, 10.52826033068511435 ) ) ;
#30323=CARTESIAN_POINT ( 'NONE',  ( -34.50000000000000000, -111.0140978167138570, 0.7502176474015694874 ) ) ;
#30325=CARTESIAN_POINT ( 'NONE',  ( -35.50000000000000000, -114.2356323198232673, 8.521029492159460261 ) ) ;
#30334=CARTESIAN_POINT ( 'NONE',  ( -35.50000000000000711, -114.0650276068786582, 9.507762098804159123 ) ) ;
#30353=CARTESIAN_POINT ( 'NONE',  ( -36.25098837183130485, -114.6652019342044184, 2.683975545821551734 ) ) ;
#30372=CARTESIAN_POINT ( 'NONE',  ( -39.00000000000000000, -115.9929510916434481, 12.59652202191340820 ) ) ;
#30384=CARTESIAN_POINT ( 'NONE',  ( -35.62769128460905677, -112.5438815906447729, 8.308975545821549957 ) ) ;
#30391=CARTESIAN_POINT ( 'NONE',  ( -35.00000000000000000, -114.0000000000000853, 2.000000000000001776 ) ) ;
#30411=CARTESIAN_POINT ( 'NONE',  ( -34.50000000000000000, -115.5178116849130276, -1.498529437126731034 ) ) ;
#30412=CARTESIAN_POINT ( 'NONE',  ( -37.49023442168701337, -114.9929510916434339, 14.11852773550420359 ) ) ;
#30413=CARTESIAN_POINT ( 'NONE',  ( -35.50000000000000000, -113.9929510916434623, 10.50436693183592141 ) ) ;
#30416=CARTESIAN_POINT ( 'NONE',  ( -34.68937937320795584, -114.9929510916434339, 13.37409560816408671 ) ) ;
#30425=CARTESIAN_POINT ( 'NONE',  ( -38.00000000000000711, -114.9929510916434339, 12.17846912687782179 ) ) ;
#30427=CARTESIAN_POINT ( 'NONE',  ( -37.05926240293133134, -116.9999999999999858, 6.378524454178448266 ) ) ;
#30429=CARTESIAN_POINT ( 'NONE',  ( -35.50000000000000711, -115.8878449012421754, -1.128496220799388494 ) ) ;
#30438=CARTESIAN_POINT ( 'NONE',  ( -35.00000000000000000, -116.0140978167138712, 0.8752176474015622709 ) ) ;
#30448=CARTESIAN_POINT ( 'NONE',  ( -35.50000000000000000, -112.8690837874180062, 2.872105769100646189 ) ) ;
#30454=CARTESIAN_POINT ( 'NONE',  ( -35.99386409314529800, -114.9929510916434339, 13.11852378322482515 ) ) ;
#30456=CARTESIAN_POINT ( 'NONE',  ( -34.54793860109200665, -113.9929510916434339, 13.00730889637958221 ) ) ;
#30460=CARTESIAN_POINT ( 'NONE',  ( -34.50000000000000000, -113.9929510916435049, 10.50625754673586876 ) ) ;
#30462=CARTESIAN_POINT ( 'NONE',  ( -39.00000000000000711, -114.9929510916434339, 12.39849696637031151 ) ) ;
#30463=CARTESIAN_POINT ( 'NONE',  ( -35.50000000000000711, -114.9912366357066986, 10.44580456020104720 ) ) ;
#30472=CARTESIAN_POINT ( 'NONE',  ( -35.50000000000000000, -113.0140978167138712, 0.8752176474015154195 ) ) ;
#30474=CARTESIAN_POINT ( 'NONE',  ( -36.23083527818512550, -116.0245472910329880, 6.284774454178450043 ) ) ;
#30482=CARTESIAN_POINT ( 'NONE',  ( -35.50000000000000711, -114.0000000000000853, 2.000000000000001776 ) ) ;
#30485=CARTESIAN_POINT ( 'NONE',  ( -35.02454729103298803, -114.8876895276775087, 4.597274454178448266 ) ) ;
#30492=CARTESIAN_POINT ( 'NONE',  ( -34.50000000000000000, -113.3557509229967764, 1.923098431109107054 ) ) ;
#30495=CARTESIAN_POINT ( 'NONE',  ( -35.50000000000000000, -113.9929510916433344, 10.50625754673586876 ) ) ;
#30498=CARTESIAN_POINT ( 'NONE',  ( -34.50000000000000000, -116.0012805033554883, -0.7876962586524312027 ) ) ;
#30499=CARTESIAN_POINT ( 'NONE',  ( -39.00000000000000000, -115.9929510916434481, 12.59652202191340820 ) ) ;
#30522=CARTESIAN_POINT ( 'NONE',  ( -36.25098837183130485, -114.6652019342044184, 4.183975545821551734 ) ) ;
#30531=CARTESIAN_POINT ( 'NONE',  ( -35.50000000000000711, -116.0124910254613297, -0.6902086197697608894 ) ) ;
#30534=CARTESIAN_POINT ( 'NONE',  ( -35.50000000000000711, -114.0185793162512908, 9.502217742515812304 ) ) ;
#30537=CARTESIAN_POINT ( 'NONE',  ( -34.50000000000000000, -114.1302255537607095, 9.515717283514957714 ) ) ;
#30539=CARTESIAN_POINT ( 'NONE',  ( -35.00000000000000000, -114.0592624029316369, 9.003524454178483793 ) ) ;
#30540=CARTESIAN_POINT ( 'NONE',  ( -36.12500000000014211, -115.9929510916434481, 14.11852480586265024 ) ) ;
#30548=CARTESIAN_POINT ( 'NONE',  ( -39.02454729103295961, -113.2308352781851539, 7.840225545821551734 ) ) ;
#30555=UNCERTAINTY_MEASURE_WITH_UNIT (LENGTH_MEASURE( 1.000000000000000082E-05 ), #8317, 'distance_accuracy_value', 'NONE');
#30576=CARTESIAN_POINT ( 'NONE',  ( -36.87500000000098055, -114.9929510916434339, 14.11852480586264846 ) ) ;
#30579=CARTESIAN_POINT ( 'NONE',  ( -36.62499999999902656, -114.9929510916434339, 14.11852480586264846 ) ) ;
#30590=CARTESIAN_POINT ( 'NONE',  ( -34.02454729103298092, -115.3019030900506294, 7.597274454178449155 ) ) ;
#30592=CARTESIAN_POINT ( 'NONE',  ( -35.50000000000000711, -115.5178116849130276, -1.498529437126731034 ) ) ;
#30601=CIRCLE ( 'NONE', #35219, 0.5000000000000004441 ) ;
#30612=ORIENTED_EDGE ( 'NONE', *, *, #9124, .F. ) ;
#30614=CARTESIAN_POINT ( 'NONE',  ( -34.50000000000000000, -114.9307644833806137, -2.624782352598442614 ) ) ;
#30616=CARTESIAN_POINT ( 'NONE',  ( -36.50000000000011369, -114.9929510916434339, 13.11852480586264669 ) ) ;
#30617=CARTESIAN_POINT ( 'NONE',  ( -37.37500000000009237, -113.9929510916434339, 14.11852480586265024 ) ) ;
#30622=CARTESIAN_POINT ( 'NONE',  ( -34.50015059926905536, -113.9929510916434339, 12.64306614848962518 ) ) ;
#30625=CARTESIAN_POINT ( 'NONE',  ( -38.00000000000000711, -115.9929510916434481, 12.17846912687782179 ) ) ;
#30639=CARTESIAN_POINT ( 'NONE',  ( -35.50000000000000000, -115.0140978167138712, -0.6247823525984408377 ) ) ;
#30641=CARTESIAN_POINT ( 'NONE',  ( -37.88768952767750164, -115.9754527089670262, 6.472274454178450043 ) ) ;
#30648=CARTESIAN_POINT ( 'NONE',  ( -35.50000000000000000, -117.0141134414687514, -0.5779076015960331603 ) ) ;
#30659=CARTESIAN_POINT ( 'NONE',  ( -34.50000000000000000, -112.0140978167138712, -0.4997823525984337878 ) ) ;
#30661=ORIENTED_EDGE ( 'NONE', *, *, #12960, .T. ) ;
#30665=CARTESIAN_POINT ( 'NONE',  ( -35.50400759022158326, -113.9929510916434339, 12.68378527132497524 ) ) ;
#30669=CARTESIAN_POINT ( 'NONE',  ( -34.50000000000000000, -112.4803765279500993, 2.803636946313094569 ) ) ;
#30671=CARTESIAN_POINT ( 'NONE',  ( -35.50000000000000000, -114.2450133963102843, 8.522190569412378736 ) ) ;
#30699=CARTESIAN_POINT ( 'NONE',  ( -35.97545270896705460, -114.3549511594417680, 2.590225545821551734 ) ) ;
#30708=CARTESIAN_POINT ( 'NONE',  ( -35.50000000000000711, -114.9819937217110635, 10.35556074009299188 ) ) ;
#30711=CARTESIAN_POINT ( 'NONE',  ( -34.50000000000000000, -114.9929510916434339, 10.52826033068511435 ) ) ;
#30715=CARTESIAN_POINT ( 'NONE',  ( -35.50000000000000000, -114.1556834383649459, 8.511484393387789282 ) ) ;
#30716=CARTESIAN_POINT ( 'NONE',  ( -35.50000000000000711, -112.0269151300720409, -0.7876962586524208776 ) ) ;
#30717=FACE_OUTER_BOUND ( 'NONE', #23511, .T. ) ;
#30725=CARTESIAN_POINT ( 'NONE',  ( -37.99999999999998579, -114.0592624029313242, 3.246475545821551734 ) ) ;
#30748=CARTESIAN_POINT ( 'NONE',  ( -34.50000000000000000, -113.4307644833805142, -0.6247823525984269599 ) ) ;
#30752=CARTESIAN_POINT ( 'NONE',  ( -34.50000000000000000, -115.9929510916434481, 10.51725893871049067 ) ) ;
#30755=CARTESIAN_POINT ( 'NONE',  ( -37.43749999999998579, -114.9929510916434339, 14.11852480586264846 ) ) ;
#30765=CARTESIAN_POINT ( 'NONE',  ( -39.97545270896702618, -112.6980969099493990, 6.847274454178448266 ) ) ;
#30767=CARTESIAN_POINT ( 'NONE',  ( -35.50000000000000711, -112.0140900043366088, -0.5935324770972457697 ) ) ;
#30785=CARTESIAN_POINT ( 'NONE',  ( -35.50000000000000000, -111.0168437565048691, 0.9961850632443862708 ) ) ;
#30787=CARTESIAN_POINT ( 'NONE',  ( -35.50005019975638021, -114.9929510916434339, 12.62670525340498529 ) ) ;
#30789=CARTESIAN_POINT ( 'NONE',  ( -38.95206139890799335, -113.9929510916434339, 13.00730889637963550 ) ) ;
#30794=CARTESIAN_POINT ( 'NONE',  ( -34.50075263804418313, -113.9929510916434339, 12.66759465831979981 ) ) ;
#30798=CARTESIAN_POINT ( 'NONE',  ( -35.50000000000000711, -114.0998638248492085, 9.511920366020609308 ) ) ;
#30811=CARTESIAN_POINT ( 'NONE',  ( -35.50000000000000000, -115.0140978167137860, -0.6411448143358557950 ) ) ;
#30813=CARTESIAN_POINT ( 'NONE',  ( -35.99999999999999289, -114.0592624029313242, 9.003524454178446490 ) ) ;
#30819=CARTESIAN_POINT ( 'NONE',  ( -35.50000000000000711, -112.0141053790792114, 0.9054673897245171243 ) ) ;
#30822=CARTESIAN_POINT ( 'NONE',  ( -36.11231047232249125, -112.0245472910329880, 4.222274454178449155 ) ) ;
#30829=CARTESIAN_POINT ( 'NONE',  ( -34.50000000000000000, -112.0140978167138712, 0.6252176474015680441 ) ) ;
#30837=CARTESIAN_POINT ( 'NONE',  ( -36.50000000000010658, -113.9929510916434339, 13.11852480586264846 ) ) ;
#30842=CARTESIAN_POINT ( 'NONE',  ( -34.50000000000000000, -113.2372261171341563, 2.916049522752222511 ) ) ;
#30843=CARTESIAN_POINT ( 'NONE',  ( -39.00000000000000000, -115.9929510916434481, 12.26648026267477221 ) ) ;
#30869=CARTESIAN_POINT ( 'NONE',  ( -38.02454729103295961, -113.6450488405582462, 6.340225545821551734 ) ) ;
#30878=CARTESIAN_POINT ( 'NONE',  ( -35.50000000000000711, -115.5178116849130276, -1.498529437126731034 ) ) ;
#30880=DIRECTION ( 'NONE',  ( 1.000000000000000000, 0.000000000000000000, 0.000000000000000000 ) ) ;
#30887=CARTESIAN_POINT ( 'NONE',  ( -34.50000000000000000, -114.9902084924877954, 10.43071793783961176 ) ) ;
#30890=CARTESIAN_POINT ( 'NONE',  ( -35.50000000000000000, -115.9927366631908825, 10.47601115720670073 ) ) ;
#30891=CARTESIAN_POINT ( 'NONE',  ( -35.50000000000000711, -112.0250551866464548, 1.025914454044489332 ) ) ;
#30901=CARTESIAN_POINT ( 'NONE',  ( -36.02454729103297382, -113.5265240346956261, 9.902725545821553510 ) ) ;
#30911=CARTESIAN_POINT ( 'NONE',  ( -39.16322519054178741, -111.9205845034225177, 4.933975545821551734 ) ) ;
#30929=CARTESIAN_POINT ( 'NONE',  ( -34.50000000000000000, -114.9307644833806137, -0.6247823525984269599 ) ) ;
#30932=CARTESIAN_POINT ( 'NONE',  ( -34.50000000000000000, -114.2253558743059330, 8.519800927820798009 ) ) ;
#30934=CARTESIAN_POINT ( 'NONE',  ( -34.97545270896703329, -113.2308352781851397, 2.909774454178448710 ) ) ;
#30935=CARTESIAN_POINT ( 'NONE',  ( -37.48437500000004263, -114.9929510916434339, 14.11852480586264846 ) ) ;
#30943=CARTESIAN_POINT ( 'NONE',  ( -33.97545270896702618, -112.8166217158120475, 4.409774454178449155 ) ) ;
#30945=CARTESIAN_POINT ( 'NONE',  ( -35.50000000000000711, -112.0651520602111191, -0.9469505670458575608 ) ) ;
#30959=CARTESIAN_POINT ( 'NONE',  ( -36.11231047232249836, -115.9754527089670262, 5.777725545821550845 ) ) ;
#30964=CARTESIAN_POINT ( 'NONE',  ( -35.50000000000000000, -111.0140978167138570, 0.5627176474015715968 ) ) ;
#30968=CARTESIAN_POINT ( 'NONE',  ( -35.95915003344517658, -114.9929510916434339, 13.11692036158763308 ) ) ;
#30969=CARTESIAN_POINT ( 'NONE',  ( -39.00000000000000000, -113.9929510916434339, 11.73841344789285657 ) ) ;
#30973=CARTESIAN_POINT ( 'NONE',  ( -36.99999999999988631, -113.9929510916434339, 14.11852480586265024 ) ) ;
#30976=CARTESIAN_POINT ( 'NONE',  ( -35.50000000000000711, -114.9929510916434339, 12.39849696637031506 ) ) ;
#30982=CARTESIAN_POINT ( 'NONE',  ( -38.00000000000000711, -115.9929510916434481, 11.91443571948719615 ) ) ;
#30989=CARTESIAN_POINT ( 'NONE',  ( -35.50000000000000000, -114.3474311500471572, -0.6247823525984269599 ) ) ;
#30991=CARTESIAN_POINT ( 'NONE',  ( -38.99999999999999289, -113.9407375970686900, 2.253524454178449155 ) ) ;
#30993=CARTESIAN_POINT ( 'NONE',  ( -36.94073759706868287, -112.0000000000000142, 4.128524454178449155 ) ) ;
#30996=CARTESIAN_POINT ( 'NONE',  ( -35.50000000000000711, -112.0154707866092707, 0.9357013553229778235 ) ) ;
#31006=CARTESIAN_POINT ( 'NONE',  ( -34.50000000000000000, -112.0140978167138712, 0.5627176474015717078 ) ) ;
#31015=CARTESIAN_POINT ( 'NONE',  ( -35.96730626674924025, -113.9929510916434339, 13.11752178341330222 ) ) ;
#31018=CARTESIAN_POINT ( 'NONE',  ( -35.50000000000000000, -113.9929510916434339, 12.57451923796416260 ) ) ;
#31019=CARTESIAN_POINT ( 'NONE',  ( -35.50000000000000000, -115.9929510916434481, 11.21034663311132107 ) ) ;
#31030=FACE_OUTER_BOUND ( 'NONE', #34744, .T. ) ;
#31046=CARTESIAN_POINT ( 'NONE',  ( -37.99999999999998579, -114.0592624029313242, 3.246475545821551734 ) ) ;
#31058=CARTESIAN_POINT ( 'NONE',  ( -36.50000000000011369, -114.9929510916434339, 13.11852480586264669 ) ) ;
#31063=CARTESIAN_POINT ( 'NONE',  ( -34.50000000000000000, -114.9929510916434339, 10.61627146648203812 ) ) ;
#31068=CARTESIAN_POINT ( 'NONE',  ( -35.50000000000000000, -114.3049001878960240, 8.530677542735578101 ) ) ;
#31069=CARTESIAN_POINT ( 'NONE',  ( -35.50000000000000711, -112.3465879560236687, 1.629585756119413364 ) ) ;
#31072=DIRECTION ( 'NONE',  ( -1.000000000000000000, 0.000000000000000000, -0.000000000000000000 ) ) ;
#31081=CARTESIAN_POINT ( 'NONE',  ( -36.52652403469559061, -114.9754527089670262, 7.277725545821552622 ) ) ;
#31090=CARTESIAN_POINT ( 'NONE',  ( -38.18337828418796676, -117.0245472910329738, 2.965225545821551734 ) ) ;
#31106=CARTESIAN_POINT ( 'NONE',  ( -34.50000000000000000, -113.1256619669233885, 1.895633585076891947 ) ) ;
#31109=CARTESIAN_POINT ( 'NONE',  ( -34.50000000000000000, -115.9929510916434481, 10.55026311463432087 ) ) ;
#31113=CARTESIAN_POINT ( 'NONE',  ( -38.98077402996267438, -114.9929510916434339, 12.86289566494346204 ) ) ;
#31124=CARTESIAN_POINT ( 'NONE',  ( -36.94073759706866156, -111.0000000000000284, 8.628524454178448266 ) ) ;
#31126=CARTESIAN_POINT ( 'NONE',  ( -35.50000000000000711, -116.0141056290913610, -0.5935324770972248976 ) ) ;
#31138=CARTESIAN_POINT ( 'NONE',  ( -35.54388159064475872, -115.3723087153909432, 2.683975545821551290 ) ) ;
#31144=CARTESIAN_POINT ( 'NONE',  ( -35.50000000000000000, -111.0780159515033034, -1.143161139953928762 ) ) ;
#31148=CARTESIAN_POINT ( 'NONE',  ( -38.99879592093640213, -113.9929510916434339, 12.67985367974111277 ) ) ;
#31151=CARTESIAN_POINT ( 'NONE',  ( -37.37500000000009237, -113.9929510916434339, 14.11852480586265024 ) ) ;
#31153=CARTESIAN_POINT ( 'NONE',  ( -36.15625000000007816, -114.9929510916434339, 13.11852480586264669 ) ) ;
#31160=CARTESIAN_POINT ( 'NONE',  ( -35.50000000000000711, -114.9922651054798308, 10.46846006712531008 ) ) ;
#31168=CARTESIAN_POINT ( 'NONE',  ( -35.50000000000000000, -115.0140978167138712, 0.8752176474015623819 ) ) ;
#31170=CARTESIAN_POINT ( 'NONE',  ( -37.05926240293131713, -115.9999999999999858, 3.378524454178448710 ) ) ;
#31172=CARTESIAN_POINT ( 'NONE',  ( -35.62769128460905677, -115.4561184093552413, 1.691024454178448710 ) ) ;
#31175=CARTESIAN_POINT ( 'NONE',  ( -35.50000000000000711, -116.0140978167138712, -0.4997823525984418369 ) ) ;
#31183=CARTESIAN_POINT ( 'NONE',  ( -34.50000000000000000, -116.0124910254613297, -0.6902086197697608894 ) ) ;
#31184=CARTESIAN_POINT ( 'NONE',  ( -35.50000000000000711, -112.3465879560236687, 1.629585756119413364 ) ) ;
#31190=CARTESIAN_POINT ( 'NONE',  ( -37.37500000000009237, -113.9929510916434339, 13.11852480586264846 ) ) ;
#31191=CARTESIAN_POINT ( 'NONE',  ( -34.50000000000000000, -113.2637153405686519, 1.912112492696748989 ) ) ;
#31193=CARTESIAN_POINT ( 'NONE',  ( -35.50000000000000000, -113.9929510916434339, 12.26648026267477398 ) ) ;
#31194=CARTESIAN_POINT ( 'NONE',  ( -35.50040135968784938, -115.9929510916434481, 12.63896776382214071 ) ) ;
#31216=SHAPE_REPRESENTATION ( 'spring', ( #21307 ), #12169 ) ;
#31218=CARTESIAN_POINT ( 'NONE',  ( -34.50000000000000000, -116.9884631899972476, -0.9506101647064282290 ) ) ;
#31222=CARTESIAN_POINT ( 'NONE',  ( -37.05926240293131713, -113.0000000000000000, 9.621475545821549957 ) ) ;
#31229=CARTESIAN_POINT ( 'NONE',  ( -35.50000000000000711, -116.0140978167138712, 0.3752176474015736507 ) ) ;
#31233=CARTESIAN_POINT ( 'NONE',  ( -35.98364338251434447, -114.9929510916434339, 13.11827392651456314 ) ) ;
#31238=CARTESIAN_POINT ( 'NONE',  ( -34.50000000000000000, -114.9929510916434339, 11.21034663311131929 ) ) ;
#31245=CARTESIAN_POINT ( 'NONE',  ( -35.50000000000000000, -115.9929510916434481, 10.72628538622835670 ) ) ;
#31246=CARTESIAN_POINT ( 'NONE',  ( -35.50000000000000711, -114.0000000000000853, 2.000000000000001776 ) ) ;
#31256=CARTESIAN_POINT ( 'NONE',  ( -37.97545270896702618, -114.4734759653044023, 6.152725545821551734 ) ) ;
#31266=CARTESIAN_POINT ( 'NONE',  ( -34.92058450342249643, -111.8367748094582197, 6.808975545821551734 ) ) ;
#31280=CARTESIAN_POINT ( 'NONE',  ( -34.50000000000000000, -112.6605569508015350, 1.812590711673265575 ) ) ;
#31284=CARTESIAN_POINT ( 'NONE',  ( -34.50000000000000000, -114.1928420708668028, 8.515919878418792166 ) ) ;
#31291=CARTESIAN_POINT ( 'NONE',  ( -38.69949915733018742, -114.9929510916434339, 13.54034599209165712 ) ) ;
#31298=CARTESIAN_POINT ( 'NONE',  ( -33.97545270896702618, -112.8166217158120475, 8.909774454178450043 ) ) ;
#31300=CARTESIAN_POINT ( 'NONE',  ( -35.50000000000000000, -113.0140978167138712, -0.1247823525984260717 ) ) ;
#31312=CARTESIAN_POINT ( 'NONE',  ( -38.45611840935523418, -112.6276912846090568, 3.433975545821551290 ) ) ;
#31319=CARTESIAN_POINT ( 'NONE',  ( -35.50000000000000000, -117.0140978167138854, -0.3122823525984416149 ) ) ;
#31324=CARTESIAN_POINT ( 'NONE',  ( -38.00000000000000711, -114.9929510916434339, 10.85830208992306822 ) ) ;
#31325=CARTESIAN_POINT ( 'NONE',  ( -34.50000000000000000, -114.0882517521923489, 9.510534276948430232 ) ) ;
#31330=CARTESIAN_POINT ( 'NONE',  ( -38.95206139890799335, -113.9929510916434339, 13.00730889637963550 ) ) ;
#31332=CARTESIAN_POINT ( 'NONE',  ( -36.62499999999902656, -114.9929510916434339, 13.11852480586264669 ) ) ;
#31340=CARTESIAN_POINT ( 'NONE',  ( -35.50000000000000711, -114.9929296450195721, 10.49869535309826674 ) ) ;
#31347=CARTESIAN_POINT ( 'NONE',  ( -35.50000000000000000, -113.4307644833805142, -0.6247823525984269599 ) ) ;
#31351=CARTESIAN_POINT ( 'NONE',  ( -38.99999999999999289, -113.9407375970686900, 2.253524454178449155 ) ) ;
#31354=CARTESIAN_POINT ( 'NONE',  ( -35.50000000000000711, -115.8137639216009234, -1.239329810084483841 ) ) ;
#31362=CARTESIAN_POINT ( 'NONE',  ( -34.50000000000000000, -115.0468226098135744, -1.624774171496087716 ) ) ;
#31372=CARTESIAN_POINT ( 'NONE',  ( -35.98364338251434447, -113.9929510916434339, 13.11827392651456314 ) ) ;
#31374=CARTESIAN_POINT ( 'NONE',  ( -35.50000000000000000, -113.9929510916434339, 12.60752341388803721 ) ) ;
#31375=CARTESIAN_POINT ( 'NONE',  ( -35.50000000000000000, -115.9874658933321001, 10.35517832894335832 ) ) ;
#31394=CARTESIAN_POINT ( 'NONE',  ( -34.50000000000000000, -114.9307644833806137, -2.624782352598442614 ) ) ;
#31398=CARTESIAN_POINT ( 'NONE',  ( -35.99999999999999289, -114.0592624029313242, 1.503524454178448710 ) ) ;
#31404=CARTESIAN_POINT ( 'NONE',  ( -34.50000000000000000, -114.1185248058627053, 1.007048908356900085 ) ) ;
#31409=CARTESIAN_POINT ( 'NONE',  ( -35.50000000000000711, -114.9929510916434339, 12.17846912687782712 ) ) ;
#31415=CARTESIAN_POINT ( 'NONE',  ( -37.43749999999998579, -114.9929510916434339, 14.11852480586264846 ) ) ;
#31421=CARTESIAN_POINT ( 'NONE',  ( -35.50000000000000000, -115.9920935318519923, 10.44577481630138749 ) ) ;
#31422=CARTESIAN_POINT ( 'NONE',  ( -35.50000000000000711, -112.0140978167138712, -0.1247823525984259746 ) ) ;
#31434=CARTESIAN_POINT ( 'NONE',  ( -38.02454729103295961, -113.6450488405582462, 6.340225545821551734 ) ) ;
#31443=CARTESIAN_POINT ( 'NONE',  ( -39.99999999999999289, -114.0592624029313242, 7.746475545821553510 ) ) ;
#31464=CARTESIAN_POINT ( 'NONE',  ( -34.50000000000000000, -115.0304602784513293, -0.6247823525985405357 ) ) ;
#31467=CARTESIAN_POINT ( 'NONE',  ( -34.57658136524561598, -115.9929510916434481, 13.10177712753338675 ) ) ;
#31471=CARTESIAN_POINT ( 'NONE',  ( -34.50000000000000000, -114.1835524127412924, 8.514811007161055656 ) ) ;
#31482=CARTESIAN_POINT ( 'NONE',  ( -39.99999999999999289, -114.0592624029313242, 6.246475545821551734 ) ) ;
#31486=CARTESIAN_POINT ( 'NONE',  ( -35.50000000000000000, -113.0140978167134449, 0.8752176474011410523 ) ) ;
#31499=CARTESIAN_POINT ( 'NONE',  ( -38.97545270896704039, -114.8876895276775087, 7.652725545821550845 ) ) ;
#31504=CARTESIAN_POINT ( 'NONE',  ( -35.50000000000000000, -114.5974311500472567, -2.624782352598442614 ) ) ;
#31511=CARTESIAN_POINT ( 'NONE',  ( -38.00000000000000711, -114.9929510916434339, 12.53051367006571937 ) ) ;
#31513=CARTESIAN_POINT ( 'NONE',  ( -34.50000000000000000, -114.1152303497977414, 9.513755561829650986 ) ) ;
#31516=CARTESIAN_POINT ( 'NONE',  ( -38.92341863475394348, -113.9929510916434339, 13.10177712753322155 ) ) ;
#31518=CARTESIAN_POINT ( 'NONE',  ( -35.50000102263782509, -114.9929510916434339, 12.62466071271731316 ) ) ;
#31524=CARTESIAN_POINT ( 'NONE',  ( -35.50000000000000711, -114.9929510916434339, 10.59426868253284226 ) ) ;
#31531=CARTESIAN_POINT ( 'NONE',  ( -34.50000000000000000, -113.4742757288593964, 0.9301473394660054739 ) ) ;
#31538=CARTESIAN_POINT ( 'NONE',  ( -36.23083527818512550, -116.0245472910329880, 6.284774454178450043 ) ) ;
#31540=CARTESIAN_POINT ( 'NONE',  ( -35.50000000000000711, -112.0140978167138712, -0.3747823525984256832 ) ) ;
#31549=CARTESIAN_POINT ( 'NONE',  ( -34.50000000000000000, -115.1446187476384040, -1.616767172155725740 ) ) ;
#31550=CARTESIAN_POINT ( 'NONE',  ( -35.50000000000000711, -112.8356783780338759, 1.859636627348750348 ) ) ;
#31557=CARTESIAN_POINT ( 'NONE',  ( -37.99974912065192001, -113.9929510916434339, 12.63488142334838749 ) ) ;
#31559=CARTESIAN_POINT ( 'NONE',  ( -35.50000000000000000, -113.9929510916434339, 11.73841344789270202 ) ) ;
#31560=CARTESIAN_POINT ( 'NONE',  ( -35.50000102263781798, -115.9929510916434481, 12.62466071271731494 ) ) ;
#31570=CARTESIAN_POINT ( 'NONE',  ( -35.50000000000000711, -112.1859307030124739, 1.448610958621386224 ) ) ;
#31572=CARTESIAN_POINT ( 'NONE',  ( -35.50000000000000711, -114.0882517521923489, 9.510534276948430232 ) ) ;
#31577=CARTESIAN_POINT ( 'NONE',  ( -34.50000000000000000, -112.8832452823708792, -2.621568770093253953 ) ) ;
#31581=CARTESIAN_POINT ( 'NONE',  ( -36.64504884055821776, -112.9754527089670688, 8.215225545821551734 ) ) ;
#31585=CARTESIAN_POINT ( 'NONE',  ( -35.50000000000000000, -113.1807644833805426, -0.6247823525984269599 ) ) ;
#31588=CARTESIAN_POINT ( 'NONE',  ( -35.50000000000000711, -114.9929510916434339, 10.94631322572069365 ) ) ;
#31590=CARTESIAN_POINT ( 'NONE',  ( -37.18750000000006395, -114.9929510916434339, 14.11852480586264846 ) ) ;
#31597=CARTESIAN_POINT ( 'NONE',  ( -35.50400759022158326, -115.9929510916434481, 12.68378527132497524 ) ) ;
#31598=CARTESIAN_POINT ( 'NONE',  ( -35.50000000000000711, -115.1770117227680998, -1.611965039240062181 ) ) ;
#31608=CARTESIAN_POINT ( 'NONE',  ( -37.66520193420439711, -114.7490116281687023, 9.058975545821549957 ) ) ;
#31616=CARTESIAN_POINT ( 'NONE',  ( -37.05926240293131713, -111.0000000000000284, 9.621475545821549957 ) ) ;
#31629=VERTEX_POINT ( 'NONE', #33985 ) ;
#31633=CARTESIAN_POINT ( 'NONE',  ( -34.50481333282507279, -115.9929510916434481, 12.74107470552716315 ) ) ;
#31635=CARTESIAN_POINT ( 'NONE',  ( -38.99999999999999289, -113.9407375970686900, 2.253524454178449155 ) ) ;
#31636=CARTESIAN_POINT ( 'NONE',  ( -34.50000000000000000, -115.9929510916434481, 11.38636890470581164 ) ) ;
#31648=CARTESIAN_POINT ( 'NONE',  ( -34.83677480945821259, -116.0794154965774965, 2.683975545821551734 ) ) ;
#31651=CARTESIAN_POINT ( 'NONE',  ( -35.50000000000000711, -116.0140978167138712, 0.6252176474015648244 ) ) ;
#31661=CARTESIAN_POINT ( 'NONE',  ( -35.00000000000000000, -113.9407375970686900, 5.496475545821551734 ) ) ;
#31666=CARTESIAN_POINT ( 'NONE',  ( -35.50000000000000000, -111.1162063037085801, -1.269118781493287607 ) ) ;
#31672=CARTESIAN_POINT ( 'NONE',  ( -38.00000000000000711, -114.9929510916434339, 12.60752341388803721 ) ) ;
#31675=CARTESIAN_POINT ( 'NONE',  ( -34.50000000000000000, -114.9929510916434339, 12.59652202191340642 ) ) ;
#31677=CARTESIAN_POINT ( 'NONE',  ( -37.53269373325071712, -114.9929510916434339, 13.11752178341324360 ) ) ;
#31679=CARTESIAN_POINT ( 'NONE',  ( -35.87745010033553683, -113.9929510916434339, 14.11371147303761475 ) ) ;
#31681=CARTESIAN_POINT ( 'NONE',  ( -37.50818044754229419, -114.9929510916434339, 13.11847460610629668 ) ) ;
#31689=CARTESIAN_POINT ( 'NONE',  ( -35.50000000000000711, -114.9929510916434339, 10.53376102667243508 ) ) ;
#31696=CARTESIAN_POINT ( 'NONE',  ( -34.50000000000000000, -113.0140978167136581, 0.8752176474015604946 ) ) ;
#31698=CARTESIAN_POINT ( 'NONE',  ( -37.88768952767750164, -115.9754527089670262, 7.972274454178450043 ) ) ;
#31704=CARTESIAN_POINT ( 'NONE',  ( -36.11231047232249125, -112.0245472910329880, 5.722274454178448266 ) ) ;
#31707=CARTESIAN_POINT ( 'NONE',  ( -35.50000000000000711, -112.0140978167138712, -0.4685323525984295134 ) ) ;
#31714=CARTESIAN_POINT ( 'NONE',  ( -34.50000000000000000, -116.0140978167138712, 0.3752176474015736507 ) ) ;
#31715=CARTESIAN_POINT ( 'NONE',  ( -35.50000000000000711, -112.0140978167138712, 0.7189676474015718188 ) ) ;
#31721=CARTESIAN_POINT ( 'NONE',  ( -34.50000000000000000, -113.9929510916434339, 10.52826033068511435 ) ) ;
#31727=CARTESIAN_POINT ( 'NONE',  ( -37.24999999999992184, -113.9929510916434339, 13.11852480586264846 ) ) ;
#31728=CARTESIAN_POINT ( 'NONE',  ( -35.50000000000000000, -115.9929510916434481, 12.50851088611648265 ) ) ;
#31740=CARTESIAN_POINT ( 'NONE',  ( -35.50000000000000711, -112.0140978167138712, 0.5627176474015717078 ) ) ;
#31743=CARTESIAN_POINT ( 'NONE',  ( -35.50000000000000711, -114.0000000000003411, 9.500000000000035527 ) ) ;
#31748=CARTESIAN_POINT ( 'NONE',  ( -35.50000000000000000, -113.8814751941374652, 2.992951091643117678 ) ) ;
#31752=CARTESIAN_POINT ( 'NONE',  ( -35.99999999999999289, -114.0592624029313242, 4.503524454178447378 ) ) ;
#31757=CARTESIAN_POINT ( 'NONE',  ( -35.50000000000000000, -115.0140978167138712, -0.5622823525984408377 ) ) ;
#31763=CARTESIAN_POINT ( 'NONE',  ( -36.31249999999995026, -114.9929510916434339, 13.11852480586264669 ) ) ;
#31766=CARTESIAN_POINT ( 'NONE',  ( -34.50000000000000000, -114.9929510916434339, 12.53051367006571581 ) ) ;
#31772=CARTESIAN_POINT ( 'NONE',  ( -35.50000000000000000, -115.9929510916434481, 12.50851088611648265 ) ) ;
#31774=CARTESIAN_POINT ( 'NONE',  ( -35.50000000000000711, -115.6286452741999113, -1.424448457485488095 ) ) ;
#31784=CARTESIAN_POINT ( 'NONE',  ( -37.47347596530441649, -114.9754527089670262, 6.472274454178449155 ) ) ;
#31794=CARTESIAN_POINT ( 'NONE',  ( -34.83677480945821259, -116.0794154965774965, 7.183975545821551734 ) ) ;
#31813=CARTESIAN_POINT ( 'NONE',  ( -34.50000000000000000, -115.9929510916434481, 11.91443571948720148 ) ) ;
#31815=CARTESIAN_POINT ( 'NONE',  ( -38.99999999999999289, -113.9407375970686900, 3.753524454178449155 ) ) ;
#31816=CARTESIAN_POINT ( 'NONE',  ( -34.50000000000000000, -115.9929510916434481, 10.51725893871049067 ) ) ;
#31826=CARTESIAN_POINT ( 'NONE',  ( -38.30190309005061522, -111.0245472910330022, 5.027725545821551734 ) ) ;
#31828=CARTESIAN_POINT ( 'NONE',  ( -35.50000000000000000, -113.0140978167142833, 0.8752176474019800478 ) ) ;
#31845=CARTESIAN_POINT ( 'NONE',  ( -35.50000000000000000, -115.6584342456100671, -2.522673865603758614 ) ) ;
#31853=CARTESIAN_POINT ( 'NONE',  ( -34.50000000000000000, -112.7472371723319355, 1.839427296857320648 ) ) ;
#31854=CARTESIAN_POINT ( 'NONE',  ( -34.51202277066418844, -114.9929510916434339, 12.81430620224972294 ) ) ;
#31856=CARTESIAN_POINT ( 'NONE',  ( -35.99181955245763476, -114.9929510916434339, 13.11847460610632687 ) ) ;
#31859=CARTESIAN_POINT ( 'NONE',  ( -34.50000000000000000, -114.9912366357066986, 10.44580456020104720 ) ) ;
#31861=CARTESIAN_POINT ( 'NONE',  ( -37.98402046630260287, -114.9929510916434339, 12.74811950270164118 ) ) ;
#31867=CARTESIAN_POINT ( 'NONE',  ( -35.50000000000000711, -114.9929501463477663, 10.50247632894551231 ) ) ;
#31869=CARTESIAN_POINT ( 'NONE',  ( -35.02454729103298803, -114.8876895276775087, 1.597274454178448710 ) ) ;
#31876=CARTESIAN_POINT ( 'NONE',  ( -34.50000000000000000, -113.0140978167138712, -0.6247823525979733228 ) ) ;
#31878=CARTESIAN_POINT ( 'NONE',  ( -37.76916472181487450, -111.9754527089670404, 8.534774454178448266 ) ) ;
#31880=CARTESIAN_POINT ( 'NONE',  ( -39.16322519054179452, -116.0794154965774823, 5.066024454178449155 ) ) ;
#31882=CARTESIAN_POINT ( 'NONE',  ( -35.50000000000000711, -112.0140978167138712, -0.5622823525984296245 ) ) ;
#31886=( NAMED_UNIT ( * ) SI_UNIT ( $, .STERADIAN. ) SOLID_ANGLE_UNIT ( ) );
#31890=CARTESIAN_POINT ( 'NONE',  ( -34.50000000000000000, -114.9724313160460696, -1.624792769101446765 ) ) ;
#31898=CARTESIAN_POINT ( 'NONE',  ( -34.50000000000000000, -113.9929510916435618, 10.50625754673588474 ) ) ;
#31901=CARTESIAN_POINT ( 'NONE',  ( -38.00000000000000711, -113.9929510916434339, 12.39849696637031151 ) ) ;
#31904=CARTESIAN_POINT ( 'NONE',  ( -38.00000000000000711, -115.9929510916434481, 12.50851088611646311 ) ) ;
#31914=CARTESIAN_POINT ( 'NONE',  ( -35.50000000000000711, -112.8511839106603247, -1.611965039240275122 ) ) ;
#31917=CARTESIAN_POINT ( 'NONE',  ( -35.50000000000000711, -114.0185793162512908, 9.502217742515812304 ) ) ;
#31923=CARTESIAN_POINT ( 'NONE',  ( -34.50000000000000000, -115.3399256288223569, -2.599147725881697291 ) ) ;
#31927=CARTESIAN_POINT ( 'NONE',  ( -36.33479806579560289, -113.2509883718313262, 8.308975545821549957 ) ) ;
#31933=CARTESIAN_POINT ( 'NONE',  ( -34.50000000000000000, -113.1061333991432321, 0.8862035858144284850 ) ) ;
#31942=CARTESIAN_POINT ( 'NONE',  ( -37.99359134332094357, -114.9929510916434339, 12.69998175888958158 ) ) ;
#31945=CARTESIAN_POINT ( 'NONE',  ( -36.99999999999989342, -114.9929510916434339, 14.11852480586264846 ) ) ;
#31947=PRODUCT ( 'spring', 'spring', '', ( #9127 ) ) ;
#31951=CARTESIAN_POINT ( 'NONE',  ( -35.50160444427493189, -115.9929510916434481, 12.65937477241749853 ) ) ;
#31963=CARTESIAN_POINT ( 'NONE',  ( -37.99999999999998579, -113.9407375970686758, 2.253524454178448710 ) ) ;
#31975=CARTESIAN_POINT ( 'NONE',  ( -39.16322519054178741, -111.9205845034225177, 7.933975545821553510 ) ) ;
#31998=CARTESIAN_POINT ( 'NONE',  ( -35.97545865737298953, -115.9929510916434481, 14.11837420659365527 ) ) ;
#32000=CARTESIAN_POINT ( 'NONE',  ( -36.11231047232249836, -112.0245472910329880, 4.222274454178449155 ) ) ;
#32001=CARTESIAN_POINT ( 'NONE',  ( -34.50000000000000000, -115.9929510916434481, 11.21034663311132107 ) ) ;
#32011=CARTESIAN_POINT ( 'NONE',  ( -35.02454729103298803, -113.1123104723225197, 5.402725545821551734 ) ) ;
#32014=CARTESIAN_POINT ( 'NONE',  ( -35.50000000000000000, -113.0140978167137860, 0.8752176474016654106 ) ) ;
#32034=CARTESIAN_POINT ( 'NONE',  ( -35.50000000000000711, -112.0140978167138712, -0.1247823525984259746 ) ) ;
#32041=CARTESIAN_POINT ( 'NONE',  ( -34.50000000000000000, -112.6605569508015350, 1.812590711673265575 ) ) ;
#32043=CARTESIAN_POINT ( 'NONE',  ( -34.50000000000000000, -114.9492820284331742, 10.20776876943783940 ) ) ;
#32046=CARTESIAN_POINT ( 'NONE',  ( -35.97955704204053262, -114.9929510916434339, 13.11812344617474579 ) ) ;
#32048=CARTESIAN_POINT ( 'NONE',  ( -34.50000000000000000, -114.1152303497977414, 9.513755561829650986 ) ) ;
#32050=CARTESIAN_POINT ( 'NONE',  ( -38.00000000000000711, -114.9929510916434339, 12.26648026267477043 ) ) ;
#32051=DIRECTION ( 'NONE',  ( -1.000000000000000000, 0.000000000000000000, 0.000000000000000000 ) ) ;
#32056=CARTESIAN_POINT ( 'NONE',  ( -37.99839555572501837, -114.9929510916434339, 12.65937477241748965 ) ) ;
#32058=CARTESIAN_POINT ( 'NONE',  ( -39.02454729103295961, -114.7691647218148745, 5.159774454178448266 ) ) ;
#32065=CARTESIAN_POINT ( 'NONE',  ( -34.50000000000000000, -113.0140978167136581, -0.6247823525984268489 ) ) ;
#32068=CARTESIAN_POINT ( 'NONE',  ( -35.54388159064475872, -112.6276912846090568, 8.816024454178448266 ) ) ;
#32082=CARTESIAN_POINT ( 'NONE',  ( -34.50000000000000000, -114.8474311500471572, -2.624782352598442614 ) ) ;
#32088=CARTESIAN_POINT ( 'NONE',  ( -38.00000000000000711, -113.9929510916434339, 12.39849696637031151 ) ) ;
#32091=CARTESIAN_POINT ( 'NONE',  ( -34.50000000000000000, -113.9465028010160381, 10.50071319044726081 ) ) ;
#32093=CARTESIAN_POINT ( 'NONE',  ( -37.46874999999995737, -115.9929510916434481, 13.11852480586264846 ) ) ;
#32104=CARTESIAN_POINT ( 'NONE',  ( -35.50000000000000711, -112.6919296022648638, -1.573728109100751116 ) ) ;
#32107=CARTESIAN_POINT ( 'NONE',  ( -35.50000000000000711, -114.5636144531578680, 9.676196722963288366 ) ) ;
#32111=CARTESIAN_POINT ( 'NONE',  ( -35.50000000000000000, -111.0140978167138570, 0.5627176474015715968 ) ) ;
#32115=CARTESIAN_POINT ( 'NONE',  ( -36.02454729103298092, -114.4734759653044307, 6.097274454178449155 ) ) ;
#32122=CARTESIAN_POINT ( 'NONE',  ( -34.50000000000000000, -115.0140978167134165, -0.6247823525984399495 ) ) ;
#32125=CARTESIAN_POINT ( 'NONE',  ( -38.00000000000000711, -114.9929510916434339, 11.73841344789285657 ) ) ;
#32127=CARTESIAN_POINT ( 'NONE',  ( -34.50000000000000000, -112.3465879560236687, 1.629585756119413364 ) ) ;
#32129=CARTESIAN_POINT ( 'NONE',  ( -34.50000000000000000, -114.9929510916434339, 12.44250253426871033 ) ) ;
#32134=CARTESIAN_POINT ( 'NONE',  ( -35.50000000000000000, -115.9929510916434481, 12.39849696637031684 ) ) ;
#32135=CARTESIAN_POINT ( 'NONE',  ( -35.50000000000000711, -112.9813730236132585, -1.624774171495860786 ) ) ;
#32143=EDGE_CURVE ( 'NONE', #18651, #17346, #30601, .T. ) ;
#32148=CARTESIAN_POINT ( 'NONE',  ( -36.94073759706866156, -113.0000000000000000, 7.128524454178450043 ) ) ;
#32156=CARTESIAN_POINT ( 'NONE',  ( -35.54388159064475872, -115.3723087153909432, 8.683975545821551734 ) ) ;
#32179=CARTESIAN_POINT ( 'NONE',  ( -38.37230871539094323, -112.5438815906447729, 8.441024454178448266 ) ) ;
#32181=CARTESIAN_POINT ( 'NONE',  ( -34.50000000000000000, -115.9929492010520846, 10.50058572605509966 ) ) ;
#32192=CARTESIAN_POINT ( 'NONE',  ( -38.45611840935523418, -112.6276912846090568, 4.933975545821551734 ) ) ;
#32211=CARTESIAN_POINT ( 'NONE',  ( -35.50000000000000711, -112.6043641208289188, 1.789429170677330649 ) ) ;
#32221=CARTESIAN_POINT ( 'NONE',  ( -34.50000000000000000, -114.9929510916434339, 12.56351784598954424 ) ) ;
#32223=CARTESIAN_POINT ( 'NONE',  ( -37.24999999999992895, -114.9929510916434339, 13.11852480586264669 ) ) ;
#32227=CARTESIAN_POINT ( 'NONE',  ( -39.00000000000000000, -113.9929510916434339, 10.50625754673587053 ) ) ;
#32229=CARTESIAN_POINT ( 'NONE',  ( -38.00000000000000711, -114.9929510916434339, 12.56351784598954779 ) ) ;
#32234=CARTESIAN_POINT ( 'NONE',  ( -37.49414064056234253, -114.9929510916434339, 13.11852578240983291 ) ) ;
#32237=CARTESIAN_POINT ( 'NONE',  ( -36.11231047232249125, -112.0245472910329880, 5.722274454178448266 ) ) ;
#32245=CARTESIAN_POINT ( 'NONE',  ( -38.18337828418795965, -110.9754527089670546, 2.534774454178448710 ) ) ;
#32260=CARTESIAN_POINT ( 'NONE',  ( -34.50000000000000000, -112.4803765279500993, 2.803636946313094569 ) ) ;
#32266=CARTESIAN_POINT ( 'NONE',  ( -34.50000000000000000, -113.8814751941377352, 10.49295109164313722 ) ) ;
#32269=CARTESIAN_POINT ( 'NONE',  ( -38.00000068757622529, -113.9929510916434339, 12.61439929482944855 ) ) ;
#32270=CARTESIAN_POINT ( 'NONE',  ( -37.62959469683911351, -115.9929510916434481, 13.10254527216511633 ) ) ;
#32282=CARTESIAN_POINT ( 'NONE',  ( -35.50000000000000711, -112.0140978167138712, 0.7189676474015718188 ) ) ;
#32284=CARTESIAN_POINT ( 'NONE',  ( -35.50000000000000711, -114.9860996047076895, 10.38555023491505835 ) ) ;
#32288=CARTESIAN_POINT ( 'NONE',  ( -35.50000000000000000, -112.3697613878167658, -2.522673865603075605 ) ) ;
#32291=CARTESIAN_POINT ( 'NONE',  ( -38.02454729103296671, -114.3549511594417396, 6.659774454178448266 ) ) ;
#32295=CARTESIAN_POINT ( 'NONE',  ( -34.50000000000000000, -113.0140978167138712, -0.3747823525984258497 ) ) ;
#32302=CARTESIAN_POINT ( 'NONE',  ( -38.00000000000000711, -114.9929510916434339, 12.59652202191340820 ) ) ;
#32305=CARTESIAN_POINT ( 'NONE',  ( -34.50000000000000000, -112.0140978167138712, -0.3747823525984256832 ) ) ;
#32310=CARTESIAN_POINT ( 'NONE',  ( -37.42187499999996447, -115.9929510916434481, 13.11852480586264846 ) ) ;
#32330=CARTESIAN_POINT ( 'NONE',  ( -38.97545270896704039, -114.8876895276775087, 6.152725545821551734 ) ) ;
#32352=CARTESIAN_POINT ( 'NONE',  ( -39.02454729103295961, -114.7691647218148745, 5.159774454178449155 ) ) ;
#32354=CARTESIAN_POINT ( 'NONE',  ( -35.24442919769867899, -115.9929510916434481, 13.92914543265605509 ) ) ;
#32364=CARTESIAN_POINT ( 'NONE',  ( -38.99999999999999289, -114.0592624029313242, 6.246475545821550845 ) ) ;
#32385=CARTESIAN_POINT ( 'NONE',  ( -35.50000000000000711, -112.1859307030124739, 1.448610958621386224 ) ) ;
#32395=CARTESIAN_POINT ( 'NONE',  ( -34.50000000000000000, -112.0140978167138712, 0.8127176474015721519 ) ) ;
#32396=CARTESIAN_POINT ( 'NONE',  ( -34.50000000000000000, -114.2305202833893816, 9.534416457224700991 ) ) ;
#32399=CARTESIAN_POINT ( 'NONE',  ( -35.69272627125609176, -114.9929510916434339, 13.01835785830562209 ) ) ;
#32402=CARTESIAN_POINT ( 'NONE',  ( -34.50000000000000000, -114.9929510916434339, 10.53376102667243508 ) ) ;
#32410=CARTESIAN_POINT ( 'NONE',  ( -38.00000000000000711, -114.9929510916434339, 12.57451923796417503 ) ) ;
#32412=CARTESIAN_POINT ( 'NONE',  ( -38.30190309005061522, -116.9754527089670546, 1.972274454178448932 ) ) ;
#32419=CARTESIAN_POINT ( 'NONE',  ( -34.02454729103298092, -115.3019030900506294, 3.097274454178448710 ) ) ;
#32432=CARTESIAN_POINT ( 'NONE',  ( -34.50000000000000000, -111.0140978167138570, -0.4997823525984338988 ) ) ;
#32437=CARTESIAN_POINT ( 'NONE',  ( -35.50000000000000711, -114.0882517521923489, 9.510534276948430232 ) ) ;
#32438=CARTESIAN_POINT ( 'NONE',  ( -34.50000000000000000, -113.9929510916434339, 10.56126450660895699 ) ) ;
#32441=CARTESIAN_POINT ( 'NONE',  ( -37.99974912065192001, -113.9929510916434339, 12.63488142334838749 ) ) ;
#32442=CARTESIAN_POINT ( 'NONE',  ( -37.99899697755054717, -115.9929510916434481, 12.65121853911336913 ) ) ;
#32453=CARTESIAN_POINT ( 'NONE',  ( -35.50000000000000000, -113.0140978167138712, 0.7189676474015717078 ) ) ;
#32455=CARTESIAN_POINT ( 'NONE',  ( -35.50000000000000711, -114.9922651054798308, 10.46846006712531008 ) ) ;
#32461=CARTESIAN_POINT ( 'NONE',  ( -35.50000000000000000, -111.0687598768285369, 1.355111303971038073 ) ) ;
#32464=CARTESIAN_POINT ( 'NONE',  ( -38.02454729103296671, -114.3549511594417396, 8.159774454178448266 ) ) ;
#32468=CARTESIAN_POINT ( 'NONE',  ( -34.50000000000000000, -113.6807644833805995, -0.6247823525984269599 ) ) ;
#32471=CARTESIAN_POINT ( 'NONE',  ( -38.00000000000000711, -114.9929510916434339, 10.85830208992306822 ) ) ;
#32474=CARTESIAN_POINT ( 'NONE',  ( -34.50000000000000000, -112.0460568841087223, -0.8839717462762063382 ) ) ;
#32479=CARTESIAN_POINT ( 'NONE',  ( -35.50000000000000711, -114.1152303497977414, 9.513755561829650986 ) ) ;
#32490=DIRECTION ( 'NONE',  ( -1.000000000000000000, 0.000000000000000000, 0.000000000000000000 ) ) ;
#32502=CARTESIAN_POINT ( 'NONE',  ( -37.76916472181486739, -116.0245472910329880, 8.965225545821551734 ) ) ;
#32522=CARTESIAN_POINT ( 'NONE',  ( -37.05926240293131713, -115.9999999999999858, 4.878524454178449155 ) ) ;
#32523=CARTESIAN_POINT ( 'NONE',  ( -36.50000000000010658, -115.9929510916434481, 14.11852480586265024 ) ) ;
#32531=CARTESIAN_POINT ( 'NONE',  ( -36.23083527818512550, -111.9754527089670404, 3.715225545821550845 ) ) ;
#32549=CARTESIAN_POINT ( 'NONE',  ( -35.02454729103298092, -113.1123104723225055, 8.402725545821551734 ) ) ;
#32557=CARTESIAN_POINT ( 'NONE',  ( -35.50000000000000711, -112.8511839106603247, -1.611965039240275122 ) ) ;
#32563=CARTESIAN_POINT ( 'NONE',  ( -34.50000000000000000, -116.0141056290913610, -0.5935324770972248976 ) ) ;
#32564=CARTESIAN_POINT ( 'NONE',  ( -37.69578139638701941, -114.9929510916434339, 14.10650203519847778 ) ) ;
#32567=CARTESIAN_POINT ( 'NONE',  ( -35.50000000000000000, -113.9929510916432207, 10.50625754673563250 ) ) ;
#32569=CARTESIAN_POINT ( 'NONE',  ( -34.50000000000000000, -114.9860996047076895, 10.38555023491505835 ) ) ;
#32574=PRESENTATION_STYLE_ASSIGNMENT (( #16172 ) ) ;
#32580=CARTESIAN_POINT ( 'NONE',  ( -35.99181955245763476, -114.9929510916434339, 13.11847460610632687 ) ) ;
#32582=CARTESIAN_POINT ( 'NONE',  ( -36.23083527818512550, -116.0245472910329880, 4.784774454178448266 ) ) ;
#32594=CARTESIAN_POINT ( 'NONE',  ( -35.69809690994938478, -111.0245472910330022, 5.722274454178450043 ) ) ;
#32608=CARTESIAN_POINT ( 'NONE',  ( -34.50000000000000000, -111.0140978167138570, -0.5622823525984297355 ) ) ;
#32614=CARTESIAN_POINT ( 'NONE',  ( -35.50000000000000711, -114.9929510916434339, 10.52000928670414126 ) ) ;
#32615=CARTESIAN_POINT ( 'NONE',  ( -34.50000000000000000, -113.9929510916434339, 12.53051367006571581 ) ) ;
#32618=CARTESIAN_POINT ( 'NONE',  ( -37.52044295795950291, -113.9929510916434339, 13.11812344617477422 ) ) ;
#32620=CARTESIAN_POINT ( 'NONE',  ( -36.03906250000000000, -115.9929510916434481, 13.11852480586264846 ) ) ;
#32637=CARTESIAN_POINT ( 'NONE',  ( -35.50000000000000711, -116.0140896356112989, -0.6575071456984549201 ) ) ;
#32642=CARTESIAN_POINT ( 'NONE',  ( -35.50000000000000711, -114.9929510916434339, 12.17846912687782712 ) ) ;
#32646=CARTESIAN_POINT ( 'NONE',  ( -35.50000000000000000, -112.5389594332240222, 2.818899826424027477 ) ) ;
#32649=CARTESIAN_POINT ( 'NONE',  ( -37.35495115944176092, -112.9754527089670688, 7.034774454178450043 ) ) ;
#32656=CARTESIAN_POINT ( 'NONE',  ( -34.50000000000000000, -113.0140978167138712, 0.3752176474015639918 ) ) ;
#32665=CARTESIAN_POINT ( 'NONE',  ( -35.50000000000000000, -113.9000545103886850, 10.49516883415891577 ) ) ;
#32669=CARTESIAN_POINT ( 'NONE',  ( -34.50000000000000000, -112.6919296022648638, -1.573728109100751116 ) ) ;
#32671=CARTESIAN_POINT ( 'NONE',  ( -36.12500000000014211, -115.9929510916434481, 14.11852480586265024 ) ) ;
#32676=CARTESIAN_POINT ( 'NONE',  ( -35.50000000000000711, -114.1021862393805577, 9.512197583835053649 ) ) ;
#32696=CARTESIAN_POINT ( 'NONE',  ( -38.99999999999999289, -114.0592624029313242, 4.746475545821550845 ) ) ;
#32713=CARTESIAN_POINT ( 'NONE',  ( -37.98325232167028531, -115.9929510916434481, 14.04194344061727584 ) ) ;
#32721=CARTESIAN_POINT ( 'NONE',  ( -38.99999999999999289, -114.0592624029313242, 4.746475545821550845 ) ) ;
#32744=CARTESIAN_POINT ( 'NONE',  ( -34.50000000000000000, -116.0140978167138712, -0.4685323525984310677 ) ) ;
#32746=CARTESIAN_POINT ( 'NONE',  ( -37.46093750000000711, -114.9929510916434339, 14.11852480586264846 ) ) ;
#32749=CARTESIAN_POINT ( 'NONE',  ( -35.50000000000000000, -113.9929510916434339, 10.50625754673586876 ) ) ;
#32751=CARTESIAN_POINT ( 'NONE',  ( -34.50000000000000000, -114.9929510916434339, 10.94631322572069365 ) ) ;
#32765=CARTESIAN_POINT ( 'NONE',  ( -34.00000000000000000, -114.0592624029313242, 1.503524454178448710 ) ) ;
#32773=CARTESIAN_POINT ( 'NONE',  ( -38.18337828418795965, -110.9754527089670546, 7.034774454178450043 ) ) ;
#32786=CARTESIAN_POINT ( 'NONE',  ( -34.50000000000000000, -111.0140978167138570, 0.8127176474015720409 ) ) ;
#32792=CARTESIAN_POINT ( 'NONE',  ( -35.50000000000000711, -114.0998638248492085, 9.511920366020609308 ) ) ;
#32794=CARTESIAN_POINT ( 'NONE',  ( -36.15625000000007816, -113.9929510916434339, 14.11852480586265024 ) ) ;
#32799=CARTESIAN_POINT ( 'NONE',  ( -34.51922597003733273, -113.9929510916434339, 12.86289566494349224 ) ) ;
#32801=CARTESIAN_POINT ( 'NONE',  ( -35.50000000000000711, -114.9929510916434339, 10.55026311463432087 ) ) ;
#32814=CARTESIAN_POINT ( 'NONE',  ( -35.50000000000000000, -113.9344536409997630, 0.9850770315317123327 ) ) ;
#32816=CARTESIAN_POINT ( 'NONE',  ( -37.74901162816869515, -114.6652019342044042, 3.566024454178448710 ) ) ;
#32819=CARTESIAN_POINT ( 'NONE',  ( -35.49999931242378892, -114.9929510916434339, 12.61439929482945566 ) ) ;
#32823=CARTESIAN_POINT ( 'NONE',  ( -35.50000000000000000, -112.4803765279500993, 2.803636946313094569 ) ) ;
#32826=CARTESIAN_POINT ( 'NONE',  ( -37.88768952767750164, -115.9754527089670262, 3.472274454178448266 ) ) ;
#32831=CARTESIAN_POINT ( 'NONE',  ( -34.50000000000000000, -115.0140978167138428, -0.6247823525986679893 ) ) ;
#32836=CARTESIAN_POINT ( 'NONE',  ( -35.50000000000000000, -113.9929510916434339, 10.51725893871049067 ) ) ;
#32844=CARTESIAN_POINT ( 'NONE',  ( -34.50000000000000000, -115.3362660311619692, -1.573728109101206085 ) ) ;
#32845=CARTESIAN_POINT ( 'NONE',  ( -35.50000000000000000, -114.2899554544714960, 8.528375582263644006 ) ) ;
#32850=CARTESIAN_POINT ( 'NONE',  ( -37.75185693410092824, -115.9929510916434481, 13.05539834812634759 ) ) ;
#32869=CARTESIAN_POINT ( 'NONE',  ( -37.88768952767750875, -112.0245472910329880, 9.527725545821557063 ) ) ;
#32881=CARTESIAN_POINT ( 'NONE',  ( -35.50000000000000711, -114.9929510916434339, 10.51175824272318415 ) ) ;
#32891=CARTESIAN_POINT ( 'NONE',  ( -36.03125000000003553, -115.9929510916434481, 14.11852480586265024 ) ) ;
#32900=CARTESIAN_POINT ( 'NONE',  ( -38.37230871539094323, -115.4561184093552413, 7.558975545821551734 ) ) ;
#32927=CARTESIAN_POINT ( 'NONE',  ( -34.50000000000000000, -112.3995503592287690, -1.424448457485529618 ) ) ;
#32928=CARTESIAN_POINT ( 'NONE',  ( -36.62499999999902656, -114.9929510916434339, 14.11852480586264846 ) ) ;
#32929=CARTESIAN_POINT ( 'NONE',  ( -35.50000000000000000, -113.9929510916435618, 10.50625754673588474 ) ) ;
#32931=CARTESIAN_POINT ( 'NONE',  ( -34.50120407906360498, -114.9929510916434339, 12.67985367974112343 ) ) ;
#32943=CARTESIAN_POINT ( 'NONE',  ( -39.97545270896702618, -112.6980969099493990, 3.847274454178448710 ) ) ;
#32950=CARTESIAN_POINT ( 'NONE',  ( -34.83677480945821259, -116.0794154965774965, 4.183975545821551734 ) ) ;
#32965=CARTESIAN_POINT ( 'NONE',  ( -35.50000000000000000, -112.7319952733504635, 2.855726801009121463 ) ) ;
#32972=CARTESIAN_POINT ( 'NONE',  ( -35.50000000000000711, -114.0185793162512908, 9.502217742515812304 ) ) ;
#32973=CARTESIAN_POINT ( 'NONE',  ( -34.50000000000000000, -113.9929510916434339, 12.60752341388803721 ) ) ;
#32976=CARTESIAN_POINT ( 'NONE',  ( -34.50000000000000000, -113.9929510916438460, 10.50625754673626133 ) ) ;
#32977=CARTESIAN_POINT ( 'NONE',  ( -39.00000000000000711, -114.9929510916434339, 12.56351784598954779 ) ) ;
#32978=CARTESIAN_POINT ( 'NONE',  ( -35.50000000000000711, -114.1021862393805577, 9.512197583835053649 ) ) ;
#32991=CARTESIAN_POINT ( 'NONE',  ( -35.50000000000000000, -113.0140978167138712, 0.5627176474015715968 ) ) ;
#32993=CARTESIAN_POINT ( 'NONE',  ( -38.02454729103296671, -114.3549511594417396, 2.159774454178448710 ) ) ;
#32999=CARTESIAN_POINT ( 'NONE',  ( -35.50000000000000711, -113.1256619669233885, 1.895633585076891947 ) ) ;
#33003=CARTESIAN_POINT ( 'NONE',  ( -34.97545270896703329, -113.2308352781851539, 4.409774454178448266 ) ) ;
#33008=CARTESIAN_POINT ( 'NONE',  ( -34.50000000000000000, -115.0140978167139707, -0.6247823525984387283 ) ) ;
#33016=CARTESIAN_POINT ( 'NONE',  ( -35.50000000000000000, -113.9929510916434339, 10.53376102667243508 ) ) ;
#33020=CARTESIAN_POINT ( 'NONE',  ( -34.50000000000000000, -111.0140978167138570, 0.3752176474015639918 ) ) ;
#33021=CARTESIAN_POINT ( 'NONE',  ( -37.88878409051687157, -115.9929510916434481, 14.07058620477052280 ) ) ;
#33027=CARTESIAN_POINT ( 'NONE',  ( -37.56526046546249376, -115.9929510916434481, 13.11451721564129258 ) ) ;
#33048=CARTESIAN_POINT ( 'NONE',  ( -36.23083527818512550, -111.9754527089670404, 9.715225545821551734 ) ) ;
#33067=CARTESIAN_POINT ( 'NONE',  ( -35.98977351030467986, -115.9929510916434481, 14.11852173794918563 ) ) ;
#33079=CARTESIAN_POINT ( 'NONE',  ( -35.54388159064475872, -115.3723087153909432, 8.683975545821551734 ) ) ;
#33105=CARTESIAN_POINT ( 'NONE',  ( -34.50000000000000000, -114.9307644833806137, -1.624782352598427959 ) ) ;
#33106=CARTESIAN_POINT ( 'NONE',  ( -36.06250000000002132, -114.9929510916434339, 14.11852480586264846 ) ) ;
#33107=CARTESIAN_POINT ( 'NONE',  ( -38.00000000000000711, -114.9929510916434339, 10.85830208992306822 ) ) ;
#33109=CARTESIAN_POINT ( 'NONE',  ( -36.03906250000000000, -114.9929510916434339, 14.11852480586264846 ) ) ;
#33122=CARTESIAN_POINT ( 'NONE',  ( -39.97545270896702618, -112.6980969099493990, 5.347274454178449155 ) ) ;
#33140=CARTESIAN_POINT ( 'NONE',  ( -35.50000000000000000, -113.0071371610607684, 2.888584676720006961 ) ) ;
#33145=CARTESIAN_POINT ( 'NONE',  ( -35.50000000000000711, -114.9929510916434339, 12.57451923796416082 ) ) ;
#33148=CARTESIAN_POINT ( 'NONE',  ( -34.50481333282507279, -113.9929510916434339, 12.74107470552716315 ) ) ;
#33149=AXIS2_PLACEMENT_3D ( 'NONE', #28198, #11991, #31072 ) ;
#33152=CARTESIAN_POINT ( 'NONE',  ( -34.50000000000000000, -113.9929510916434339, 10.51175824272318415 ) ) ;
#33154=CARTESIAN_POINT ( 'NONE',  ( -35.50000000000000711, -114.1861579685891712, 9.524983039397698192 ) ) ;
#33168=CARTESIAN_POINT ( 'NONE',  ( -35.50000000000000000, -113.0140978167140702, 0.8752176474015694874 ) ) ;
#33170=CARTESIAN_POINT ( 'NONE',  ( -38.45611840935523418, -115.3723087153909432, 3.566024454178448710 ) ) ;
#33177=CARTESIAN_POINT ( 'NONE',  ( -35.50000000000000711, -112.1859307030124739, 1.448610958621386224 ) ) ;
#33181=CARTESIAN_POINT ( 'NONE',  ( -36.11231047232249125, -112.0245472910329880, 8.722274454178448266 ) ) ;
#33186=CARTESIAN_POINT ( 'NONE',  ( -34.50000000000000000, -115.0140978167138712, -0.1247823525984438492 ) ) ;
#33191=CARTESIAN_POINT ( 'NONE',  ( -35.50000000000000000, -113.9929510916434623, 10.50436693183592141 ) ) ;
#33194=CARTESIAN_POINT ( 'NONE',  ( -34.50000000000000000, -115.8137639216009234, -1.239329810084483841 ) ) ;
#33197=CARTESIAN_POINT ( 'NONE',  ( -37.49023442168701337, -115.9929510916434481, 14.11852773550420359 ) ) ;
#33224=CARTESIAN_POINT ( 'NONE',  ( -36.52652403469559061, -114.9754527089670262, 2.777725545821551734 ) ) ;
#33235=CARTESIAN_POINT ( 'NONE',  ( -35.50000000000000711, -114.1489256397697289, 9.518467544735724317 ) ) ;
#33238=CARTESIAN_POINT ( 'NONE',  ( -34.50000000000000000, -114.0000000000003411, 9.500000000000035527 ) ) ;
#33244=CARTESIAN_POINT ( 'NONE',  ( -36.00976557831293690, -115.9929510916434481, 14.11852773550420359 ) ) ;
#33255=CARTESIAN_POINT ( 'NONE',  ( -35.00000000000000000, -113.9407375970686900, 9.996475545821549957 ) ) ;
#33281=CARTESIAN_POINT ( 'NONE',  ( -34.50000000000000000, -112.0140978167138712, -0.3122823525984337878 ) ) ;
#33282=CARTESIAN_POINT ( 'NONE',  ( -37.24999999999992895, -114.9929510916434339, 14.11852480586264846 ) ) ;
#33284=CARTESIAN_POINT ( 'NONE',  ( -35.50000000000000000, -113.9929510916434339, 10.51725893871049067 ) ) ;
#33287=CARTESIAN_POINT ( 'NONE',  ( -36.31249999999995026, -114.9929510916434339, 14.11852480586264846 ) ) ;
#33296=CARTESIAN_POINT ( 'NONE',  ( -37.05926240293133134, -116.9999999999999858, 3.378524454178448710 ) ) ;
#33298=CARTESIAN_POINT ( 'NONE',  ( -35.50000000000000711, -113.0557643173828524, -1.624792769101735868 ) ) ;
#33315=CARTESIAN_POINT ( 'NONE',  ( -35.50000000000000000, -112.6572589393539516, 2.844055607295835397 ) ) ;
#33319=CARTESIAN_POINT ( 'NONE',  ( -35.50000000000000711, -114.9929510916434339, 12.59652202191340642 ) ) ;
#33321=CARTESIAN_POINT ( 'NONE',  ( -34.50000000000000000, -113.9929510916434339, 11.21034663311132107 ) ) ;
#33327=CARTESIAN_POINT ( 'NONE',  ( -34.50000000000000000, -113.9929510916434339, 12.59652202191340464 ) ) ;
#33328=CARTESIAN_POINT ( 'NONE',  ( -38.69949915733018742, -114.9929510916434339, 13.54034599209165712 ) ) ;
#33329=CARTESIAN_POINT ( 'NONE',  ( -35.50000000000000711, -114.9929510916434339, 11.21034663311131929 ) ) ;
#33339=CARTESIAN_POINT ( 'NONE',  ( -35.50000000000000000, -115.0140978167138712, -0.6247823525985405357 ) ) ;
#33341=CARTESIAN_POINT ( 'NONE',  ( -37.76916472181487450, -111.9754527089670404, 5.534774454178449155 ) ) ;
#33347=CARTESIAN_POINT ( 'NONE',  ( -35.50000000000000711, -112.0140978167138712, 0.7502176474015694874 ) ) ;
#33350=CARTESIAN_POINT ( 'NONE',  ( -38.45611840935523418, -115.3723087153909432, 8.066024454178448266 ) ) ;
#33356=CARTESIAN_POINT ( 'NONE',  ( -34.50000000000000000, -112.0140978167138712, 0.7502176474015694874 ) ) ;
#33362=CARTESIAN_POINT ( 'NONE',  ( -35.50005019975638021, -113.9929510916434339, 12.62670525340498351 ) ) ;
#33366=CARTESIAN_POINT ( 'NONE',  ( -34.50000000000000000, -116.0140978167138712, -0.1247823525984439463 ) ) ;
#33367=CARTESIAN_POINT ( 'NONE',  ( -39.00000000000000000, -115.9929510916434481, 10.50625754673587053 ) ) ;
#33389=CARTESIAN_POINT ( 'NONE',  ( -37.66520193420439711, -114.7490116281687023, 3.058975545821551734 ) ) ;
#33398=CARTESIAN_POINT ( 'NONE',  ( -35.50000000000000711, -114.3474311500471430, -1.624782352598427959 ) ) ;
#33401=CARTESIAN_POINT ( 'NONE',  ( -35.50000000000000711, -114.2598117360253696, 9.542047897280109936 ) ) ;
#33405=CARTESIAN_POINT ( 'NONE',  ( -34.50000000000000000, -114.9925223117477202, 10.47601618151863079 ) ) ;
#33409=CARTESIAN_POINT ( 'NONE',  ( -35.50000000000000000, -114.5266723804073195, 8.577838247824468354 ) ) ;
#33410=CARTESIAN_POINT ( 'NONE',  ( -35.50000000000000711, -112.0221129971568104, -0.7553032835231431319 ) ) ;
#33418=CARTESIAN_POINT ( 'NONE',  ( -34.97545270896703329, -114.7691647218148745, 8.590225545821551734 ) ) ;
#33447=CARTESIAN_POINT ( 'NONE',  ( -34.50000000000000000, -115.0140978167138712, -0.1247823525984438492 ) ) ;
#33450=CARTESIAN_POINT ( 'NONE',  ( -34.50000000000000000, -114.2356323198232673, 8.521029492159460261 ) ) ;
#33453=CARTESIAN_POINT ( 'NONE',  ( -37.34375000000001421, -114.9929510916434339, 14.11852480586264846 ) ) ;
#33462=CARTESIAN_POINT ( 'NONE',  ( -38.30190309005061522, -116.9754527089670546, 3.472274454178448710 ) ) ;
#33465=CARTESIAN_POINT ( 'NONE',  ( -35.50000000000000711, -112.0140978167138712, -0.4997823525984337878 ) ) ;
#33476=ORIENTED_EDGE ( 'NONE', *, *, #10831, .F. ) ;
#33485=CARTESIAN_POINT ( 'NONE',  ( -35.50000000000000000, -111.0360125565790383, 1.176611260687384419 ) ) ;
#33487=CARTESIAN_POINT ( 'NONE',  ( -35.50040135968785648, -114.9929510916434339, 12.63896776382214071 ) ) ;
#33489=CARTESIAN_POINT ( 'NONE',  ( -37.69578139638701941, -113.9929510916434339, 14.10650203519847778 ) ) ;
#33494=CARTESIAN_POINT ( 'NONE',  ( -34.50481333282507279, -113.9929510916434339, 12.74107470552716315 ) ) ;
#33495=CARTESIAN_POINT ( 'NONE',  ( -38.95206139890800046, -114.9929510916434339, 13.00730889637963728 ) ) ;
#33496=CARTESIAN_POINT ( 'NONE',  ( -35.50000000000000711, -114.2598117360253696, 9.542047897280109936 ) ) ;
#33509=CARTESIAN_POINT ( 'NONE',  ( -35.50000000000000000, -115.0140978167138712, -0.6247823525984418369 ) ) ;
#33512=CARTESIAN_POINT ( 'NONE',  ( -36.23083527818512550, -116.0245472910329880, 4.784774454178448266 ) ) ;
#33518=CARTESIAN_POINT ( 'NONE',  ( -35.50000000000000711, -112.4434344552011282, 1.705278471174987986 ) ) ;
#33529=CARTESIAN_POINT ( 'NONE',  ( -34.50000000000000000, -115.0140978167139707, -0.6091573525984161908 ) ) ;
#33535=CARTESIAN_POINT ( 'NONE',  ( -35.50000000000000000, -113.9929510916434339, 10.50625754673587409 ) ) ;
#33538=CARTESIAN_POINT ( 'NONE',  ( -34.50000000000000000, -111.0687598768285369, 1.355111303971038073 ) ) ;
#33539=CARTESIAN_POINT ( 'NONE',  ( -35.50000000000000000, -114.7000328234681206, 8.631511418192262752 ) ) ;
#33563=CARTESIAN_POINT ( 'NONE',  ( -35.99999999999999289, -113.9407375970686758, 5.496475545821551734 ) ) ;
#33571=CARTESIAN_POINT ( 'NONE',  ( -35.50000000000000711, -116.0140978167138712, -0.3747823525984422255 ) ) ;
#33579=CARTESIAN_POINT ( 'NONE',  ( -35.50000000000000000, -114.3793648455349654, 8.543708532059524074 ) ) ;
#33580=CARTESIAN_POINT ( 'NONE',  ( -35.50000000000000711, -112.8356783780338759, 1.859636627348750348 ) ) ;
#33591=CARTESIAN_POINT ( 'NONE',  ( -35.97545270896705460, -114.3549511594417680, 2.590225545821551734 ) ) ;
#33601=CARTESIAN_POINT ( 'NONE',  ( -39.99999999999999289, -113.9407375970686758, 8.253524454178448266 ) ) ;
#33617=CARTESIAN_POINT ( 'NONE',  ( -34.50000000000000000, -114.0000000000000853, 2.000000000000001776 ) ) ;
#33619=CARTESIAN_POINT ( 'NONE',  ( -34.50000000000000000, -116.0140978167138712, 0.3752176474015736507 ) ) ;
#33620=CARTESIAN_POINT ( 'NONE',  ( -39.00000000000000711, -114.9929510916434339, 10.50625754673587231 ) ) ;
#33623=CARTESIAN_POINT ( 'NONE',  ( -38.99518666717493431, -114.9929510916434339, 12.74107470552714716 ) ) ;
#33634=CARTESIAN_POINT ( 'NONE',  ( -35.81662171581204746, -117.0245472910329738, 6.284774454178449155 ) ) ;
#33636=CARTESIAN_POINT ( 'NONE',  ( -35.50000000000000711, -114.9307644833806137, -1.624782352598427959 ) ) ;
#33649=CARTESIAN_POINT ( 'NONE',  ( -35.00000000000000000, -113.9407375970686900, 3.996475545821551290 ) ) ;
#33655=CARTESIAN_POINT ( 'NONE',  ( -35.50000000000000000, -111.0140978167138570, 0.7502176474015694874 ) ) ;
#33658=CARTESIAN_POINT ( 'NONE',  ( -37.46874999999996447, -114.9929510916434339, 13.11852480586264669 ) ) ;
#33660=CARTESIAN_POINT ( 'NONE',  ( -38.99984940073100148, -113.9929510916434339, 12.64306614848957544 ) ) ;
#33664=CARTESIAN_POINT ( 'NONE',  ( -36.03125000000003553, -113.9929510916434339, 14.11852480586265024 ) ) ;
#33668=CARTESIAN_POINT ( 'NONE',  ( -35.50640865667918433, -114.9929510916434339, 12.69998175888958514 ) ) ;
#33675=CARTESIAN_POINT ( 'NONE',  ( -35.50000000000000711, -114.5636144531578680, 9.676196722963288366 ) ) ;
#33684=CARTESIAN_POINT ( 'NONE',  ( -35.50000000000000000, -115.0140978167138712, -0.4997823525984417259 ) ) ;
#33686=CARTESIAN_POINT ( 'NONE',  ( -38.45611840935523418, -115.3723087153909432, 2.066024454178448710 ) ) ;
#33689=CARTESIAN_POINT ( 'NONE',  ( -34.97545270896703329, -113.2308352781851539, 7.409774454178451819 ) ) ;
#33694=CARTESIAN_POINT ( 'NONE',  ( -35.50000000000000000, -114.9307644833806137, -2.624782352598442614 ) ) ;
#33697=CARTESIAN_POINT ( 'NONE',  ( -37.76916472181487450, -111.9754527089670404, 4.034774454178449155 ) ) ;
#33703=CARTESIAN_POINT ( 'NONE',  ( -34.50000000000000000, -112.0140978167138712, -0.5622823525984296245 ) ) ;
#33712=CARTESIAN_POINT ( 'NONE',  ( -37.48437500000004263, -113.9929510916434339, 13.11852480586264846 ) ) ;
#33717=CARTESIAN_POINT ( 'NONE',  ( -34.50000000000000000, -116.0140978167138712, -0.3747823525984422255 ) ) ;
#33718=CARTESIAN_POINT ( 'NONE',  ( -35.50000000000000000, -114.8124184834118324, 8.677834500183694288 ) ) ;
#33748=CARTESIAN_POINT ( 'NONE',  ( -36.25098837183130485, -114.6652019342044184, 7.183975545821551734 ) ) ;
#33756=CARTESIAN_POINT ( 'NONE',  ( -35.50000000000000711, -113.3474311500483935, -1.624782352598427959 ) ) ;
#33762=CARTESIAN_POINT ( 'NONE',  ( -36.07812499999994316, -114.9929510916434339, 13.11852480586264669 ) ) ;
#33768=CARTESIAN_POINT ( 'NONE',  ( -34.50000000000000000, -114.8211182053456838, 9.932864235516914775 ) ) ;
#33773=CARTESIAN_POINT ( 'NONE',  ( -35.50000000000000000, -114.3496480102005251, 8.538090462223289379 ) ) ;
#33774=CARTESIAN_POINT ( 'NONE',  ( -35.50000000000000711, -112.0140978167138712, 0.3752176474015640473 ) ) ;
#33786=CARTESIAN_POINT ( 'NONE',  ( -37.66520193420439711, -114.7490116281687023, 7.558975545821551734 ) ) ;
#33796=CARTESIAN_POINT ( 'NONE',  ( -34.92058450342249643, -111.8367748094582197, 3.808975545821551734 ) ) ;
#33812=CARTESIAN_POINT ( 'NONE',  ( -34.50000000000000000, -113.3557509229967764, 1.923098431109107054 ) ) ;
#33815=CARTESIAN_POINT ( 'NONE',  ( -34.50000000000000000, -115.9929510916434481, 10.53376102667243508 ) ) ;
#33818=CARTESIAN_POINT ( 'NONE',  ( -34.50000000000000000, -114.2675000158779710, 8.525177020294046670 ) ) ;
#33827=CARTESIAN_POINT ( 'NONE',  ( -39.97545270896702618, -115.3019030900506152, 7.652725545821552622 ) ) ;
#33829=CARTESIAN_POINT ( 'NONE',  ( -35.50000000000000711, -112.0140978167138712, 0.0002176474015661141945 ) ) ;
#33841=CARTESIAN_POINT ( 'NONE',  ( -36.94073759706868287, -115.9999999999999858, 7.371475545821551734 ) ) ;
#33846=CARTESIAN_POINT ( 'NONE',  ( -35.50000000000000000, -116.9501796819249222, -1.143161139954000260 ) ) ;
#33850=CARTESIAN_POINT ( 'NONE',  ( -38.00000000000000711, -114.9929510916434339, 11.21034663311206181 ) ) ;
#33851=CARTESIAN_POINT ( 'NONE',  ( -39.00000000000000000, -113.9929510916434339, 12.60752341388803721 ) ) ;
#33856=CARTESIAN_POINT ( 'NONE',  ( -37.98325232167028531, -113.9929510916434339, 14.04194344061727584 ) ) ;
#33859=CARTESIAN_POINT ( 'NONE',  ( -35.97955704204053262, -114.9929510916434339, 13.11812344617474579 ) ) ;
#33866=CARTESIAN_POINT ( 'NONE',  ( -35.50000000000000711, -114.9929510916434339, 12.59102132592610523 ) ) ;
#33869=CARTESIAN_POINT ( 'NONE',  ( -38.37230871539094323, -112.5438815906447729, 3.941024454178448710 ) ) ;
#33873=CARTESIAN_POINT ( 'NONE',  ( -35.50000000000000000, -115.0140978167138712, 0.6252176474015650465 ) ) ;
#33875=CARTESIAN_POINT ( 'NONE',  ( -35.02454729103298803, -114.8876895276775087, 3.097274454178448710 ) ) ;
#33877=CARTESIAN_POINT ( 'NONE',  ( -35.02454729103298803, -114.8876895276775087, 3.097274454178448710 ) ) ;
#33880=CARTESIAN_POINT ( 'NONE',  ( -35.50000000000000711, -115.9630435732166518, -0.9469505670456015434 ) ) ;
#33888=CARTESIAN_POINT ( 'NONE',  ( -34.50000000000000000, -115.6286452741999113, -1.424448457485488095 ) ) ;
#33889=CARTESIAN_POINT ( 'NONE',  ( -35.50000000000000711, -113.1256619669233885, 1.895633585076891947 ) ) ;
#33897=CARTESIAN_POINT ( 'NONE',  ( -37.53269373325071712, -113.9929510916434339, 13.11752178341324360 ) ) ;
#33901=CARTESIAN_POINT ( 'NONE',  ( -35.50160444427493189, -113.9929510916434339, 12.65937477241749853 ) ) ;
#33903=CARTESIAN_POINT ( 'NONE',  ( -35.50000000000000000, -115.9929510916434481, 10.52000928670414126 ) ) ;
#33929=CARTESIAN_POINT ( 'NONE',  ( -37.05926240293133134, -115.0000000000000000, 1.878524454178448710 ) ) ;
#33940=CARTESIAN_POINT ( 'NONE',  ( -35.50000000000000711, -114.9929510916434339, 10.85830208992344303 ) ) ;
#33946=CARTESIAN_POINT ( 'NONE',  ( -34.50000000000000000, -114.9928438774171582, 10.49113435197128652 ) ) ;
#33951=CARTESIAN_POINT ( 'NONE',  ( -35.50000000000000000, -115.9929510916434481, 10.55026311463432087 ) ) ;
#33963=CARTESIAN_POINT ( 'NONE',  ( -35.99999999999999289, -113.9407375970686758, 5.496475545821551734 ) ) ;
#33975=CARTESIAN_POINT ( 'NONE',  ( -33.97545270896702618, -112.8166217158120475, 5.909774454178450931 ) ) ;
#33985=CARTESIAN_POINT ( 'NONE',  ( -35.50000000000000711, -114.0000000000003411, 9.500000000000035527 ) ) ;
#33992=CARTESIAN_POINT ( 'NONE',  ( -34.50000000000000000, -112.7765286249690035, 1.847058736912741583 ) ) ;
#33995=CARTESIAN_POINT ( 'NONE',  ( -39.00000000000000711, -114.9929510916434339, 12.17846912687782179 ) ) ;
#34000=CARTESIAN_POINT ( 'NONE',  ( -38.99999693208653895, -114.9929510916434339, 12.62875129555797749 ) ) ;
#34009=CARTESIAN_POINT ( 'NONE',  ( -34.92058450342249643, -111.8367748094582197, 6.808975545821551734 ) ) ;
#34011=CARTESIAN_POINT ( 'NONE',  ( -35.50000000000000000, -113.0140978167138712, 0.3752176474015639918 ) ) ;
#34022=CARTESIAN_POINT ( 'NONE',  ( -37.05926240293131713, -112.0000000000000142, 3.621475545821551290 ) ) ;
#34029=CARTESIAN_POINT ( 'NONE',  ( -35.50000000000000000, -117.0108842342086888, -0.7556348869410856040 ) ) ;
#34032=CARTESIAN_POINT ( 'NONE',  ( -37.99974912065192711, -114.9929510916434339, 12.63488142334838571 ) ) ;
#34033=CARTESIAN_POINT ( 'NONE',  ( -34.50000000000000000, -114.0743172650041686, 9.508870970061893857 ) ) ;
#34036=CARTESIAN_POINT ( 'NONE',  ( -38.69949915733018742, -113.9929510916434339, 13.54034599209165890 ) ) ;
#34038=CARTESIAN_POINT ( 'NONE',  ( -36.03125000000004263, -114.9929510916434339, 13.11852480586264669 ) ) ;
#34044=CARTESIAN_POINT ( 'NONE',  ( -35.50000000000000711, -114.8211182053456838, 9.932864235516914775 ) ) ;
#34047=CARTESIAN_POINT ( 'NONE',  ( -34.97545270896703329, -113.2308352781851539, 2.909774454178448710 ) ) ;
#34053=CARTESIAN_POINT ( 'NONE',  ( -35.50000000000000000, -113.0140978167137717, -0.6411448143358797758 ) ) ;
#34057=CARTESIAN_POINT ( 'NONE',  ( -34.97545270896703329, -113.2308352781851539, 2.909774454178448710 ) ) ;
#34060=CARTESIAN_POINT ( 'NONE',  ( -35.50000000000000711, -115.2732872103912030, -1.592823285204062911 ) ) ;
#34065=( NAMED_UNIT ( * ) PLANE_ANGLE_UNIT ( ) SI_UNIT ( $, .RADIAN. ) );
#34069=CARTESIAN_POINT ( 'NONE',  ( -34.50000000000000000, -116.0140978167138712, -0.3122823525984417259 ) ) ;
#34076=CARTESIAN_POINT ( 'NONE',  ( -35.74814306589956203, -113.9929510916434339, 13.05539834812772781 ) ) ;
#34079=CARTESIAN_POINT ( 'NONE',  ( -35.98364338251434447, -113.9929510916434339, 13.11827392651456314 ) ) ;
#34080=CARTESIAN_POINT ( 'NONE',  ( -35.50000000000000000, -115.9929510916434481, 12.44250253426871033 ) ) ;
#34102=CARTESIAN_POINT ( 'NONE',  ( -34.50000000000000000, -117.0108842342086888, -0.7556348869410856040 ) ) ;
#34106=CARTESIAN_POINT ( 'NONE',  ( -36.52652403469556930, -113.0245472910329880, 2.722274454178449155 ) ) ;
#34113=CARTESIAN_POINT ( 'NONE',  ( -35.50000000000000000, -115.0140978167138712, -0.6247823525984418369 ) ) ;
#34117=CARTESIAN_POINT ( 'NONE',  ( -35.50000000000000711, -114.9929510916434339, 10.53376102667243508 ) ) ;
#34123=CARTESIAN_POINT ( 'NONE',  ( -35.90191880024783444, -114.9929510916434339, 14.11551573851448893 ) ) ;
#34127=CARTESIAN_POINT ( 'NONE',  ( -35.50000000000000000, -115.9929510916434481, 10.56126450660895699 ) ) ;
#34128=CARTESIAN_POINT ( 'NONE',  ( -35.50000000000000711, -112.0140978167138712, -0.3122823525984337878 ) ) ;
#34141=CARTESIAN_POINT ( 'NONE',  ( -38.02454729103295961, -113.6450488405582462, 4.840225545821551734 ) ) ;
#34151=CARTESIAN_POINT ( 'NONE',  ( -39.16322519054178741, -111.9205845034225177, 6.433975545821551734 ) ) ;
#34168=CARTESIAN_POINT ( 'NONE',  ( -34.50000000000000000, -115.0140978167137860, -0.6247823525984403936 ) ) ;
#34172=CARTESIAN_POINT ( 'NONE',  ( -34.50000000000000000, -114.2067765580549832, 8.517583185305328541 ) ) ;
#34177=CARTESIAN_POINT ( 'NONE',  ( -38.99699093265173389, -114.9929510916434339, 12.71660600561481402 ) ) ;
#34185=CARTESIAN_POINT ( 'NONE',  ( -35.69809690994941320, -116.9754527089670546, 5.777725545821551734 ) ) ;
#34188=CARTESIAN_POINT ( 'NONE',  ( -35.50000000000000711, -116.0140978167138712, -0.1247823525984439463 ) ) ;
#34197=CARTESIAN_POINT ( 'NONE',  ( -37.88768952767750875, -112.0245472910329880, 6.527725545821550845 ) ) ;
#34203=CARTESIAN_POINT ( 'NONE',  ( -35.50000000000000000, -113.0765974847181781, -2.624803185604914102 ) ) ;
#34207=CARTESIAN_POINT ( 'NONE',  ( -37.80727372874345349, -114.9929510916434339, 13.01835785830664527 ) ) ;
#34211=CARTESIAN_POINT ( 'NONE',  ( -37.98325232167028531, -113.9929510916434339, 14.04194344061727584 ) ) ;
#34214=CARTESIAN_POINT ( 'NONE',  ( -38.99999693208653895, -113.9929510916434339, 12.62875129555797749 ) ) ;
#34216=CARTESIAN_POINT ( 'NONE',  ( -37.43749999999998579, -114.9929510916434339, 13.11852480586264669 ) ) ;
#34223=CARTESIAN_POINT ( 'NONE',  ( -35.50000000000000711, -114.9929510916434339, 12.44250253426871033 ) ) ;
#34231=CARTESIAN_POINT ( 'NONE',  ( -34.50000000000000000, -113.0140978167137717, 0.8752176474015607166 ) ) ;
#34235=CARTESIAN_POINT ( 'NONE',  ( -38.45611840935523418, -115.3723087153909432, 5.066024454178449155 ) ) ;
#34238=CARTESIAN_POINT ( 'NONE',  ( -35.50000000000000711, -112.0141059978162019, -0.6575071456984691309 ) ) ;
#34246=CARTESIAN_POINT ( 'NONE',  ( -34.50000000000000000, -114.5974311500472425, -1.624782352598427959 ) ) ;
#34247=CARTESIAN_POINT ( 'NONE',  ( -35.50000000000000711, -112.9876085932806262, 1.879154677457530065 ) ) ;
#34255=CARTESIAN_POINT ( 'NONE',  ( -36.07812499999994316, -113.9929510916434339, 13.11852480586264846 ) ) ;
#34257=CARTESIAN_POINT ( 'NONE',  ( -36.12500000000014211, -113.9929510916434339, 13.11852480586264846 ) ) ;
#34258=CARTESIAN_POINT ( 'NONE',  ( -35.50000000000000000, -115.9382890315277308, 10.02636389016632812 ) ) ;
#34261=APPLICATION_CONTEXT ( 'automotive_design' ) ;
#34270=CARTESIAN_POINT ( 'NONE',  ( -35.50000000000000711, -112.0460568841087223, -0.8839717462762063382 ) ) ;
#34273=CARTESIAN_POINT ( 'NONE',  ( -35.50000000000000711, -114.1021862393805577, 9.512197583835053649 ) ) ;
#34280=CARTESIAN_POINT ( 'NONE',  ( -34.50000000000000000, -113.2224311500466030, -2.624782352598442614 ) ) ;
#34284=CARTESIAN_POINT ( 'NONE',  ( -36.25098837183129774, -113.3347980657956242, 4.316024454178448266 ) ) ;
#34291=CARTESIAN_POINT ( 'NONE',  ( -35.50000000000000000, -113.2224311500466030, -0.6247823525984269599 ) ) ;
#34297=CARTESIAN_POINT ( 'NONE',  ( -36.12500000000014211, -114.9929510916434339, 13.11852480586264669 ) ) ;
#34303=CARTESIAN_POINT ( 'NONE',  ( -34.50000000000000000, -114.9929510916434339, 12.59652202191340642 ) ) ;
#34309=CARTESIAN_POINT ( 'NONE',  ( -35.50000000000000000, -115.9929510916434481, 12.59652202191340464 ) ) ;
#34310=CARTESIAN_POINT ( 'NONE',  ( -35.50000000000000711, -115.2732872103912030, -1.592823285204062911 ) ) ;
#34320=CARTESIAN_POINT ( 'NONE',  ( -35.99999999999999289, -113.9407375970686758, 8.496475545821549957 ) ) ;
#34329=CARTESIAN_POINT ( 'NONE',  ( -39.97545270896702618, -115.3019030900506152, 7.652725545821552622 ) ) ;
#34351=CARTESIAN_POINT ( 'NONE',  ( -37.18750000000004974, -115.9929510916434481, 14.11852480586265024 ) ) ;
#34356=CARTESIAN_POINT ( 'NONE',  ( -37.56132887387857267, -114.9929510916434339, 14.11732072679899197 ) ) ;
#34368=CARTESIAN_POINT ( 'NONE',  ( -33.97545270896703329, -115.1833782841879810, 2.590225545821551734 ) ) ;
#34371=CARTESIAN_POINT ( 'NONE',  ( -35.50000000000000000, -113.0140978167136581, 0.8752176474015604946 ) ) ;
#34373=VERTEX_POINT ( 'NONE', #15745 ) ;
#34384=CARTESIAN_POINT ( 'NONE',  ( -35.00000000000000000, -113.9407375970686900, 6.996475545821551734 ) ) ;
#34391=CARTESIAN_POINT ( 'NONE',  ( -35.50000000000000000, -117.0140978167138854, -0.1247823525984438492 ) ) ;
#34400=CARTESIAN_POINT ( 'NONE',  ( -34.50000000000000000, -114.9929510916434339, 11.21034663311131929 ) ) ;
#34402=CARTESIAN_POINT ( 'NONE',  ( -37.48437500000004263, -114.9929510916434339, 13.11852480586264669 ) ) ;
#34404=CARTESIAN_POINT ( 'NONE',  ( -34.80050084267116972, -113.9929510916434339, 13.54034599209289347 ) ) ;
#34407=CARTESIAN_POINT ( 'NONE',  ( -37.48437500000004263, -114.9929510916434339, 13.11852480586264669 ) ) ;
#34413=CARTESIAN_POINT ( 'NONE',  ( -35.50000000000000711, -114.9929510916434339, 10.68227981832981044 ) ) ;
#34421=CARTESIAN_POINT ( 'NONE',  ( -34.50000000000000000, -113.0140978167138712, 0.8752176474013583229 ) ) ;
#34426=CARTESIAN_POINT ( 'NONE',  ( -38.45611840935523418, -115.3723087153909432, 2.066024454178448710 ) ) ;
#34430=CARTESIAN_POINT ( 'NONE',  ( -35.50000000000000711, -115.0468226098135744, -1.624774171496087716 ) ) ;
#34438=CARTESIAN_POINT ( 'NONE',  ( -34.50000000000000000, -116.0140978167138712, 0.8752176474015622709 ) ) ;
#34439=CARTESIAN_POINT ( 'NONE',  ( -35.50000000000000711, -112.0577668799241309, 1.173706424699810569 ) ) ;
#34448=CARTESIAN_POINT ( 'NONE',  ( -37.52044295795950291, -113.9929510916434339, 13.11812344617477422 ) ) ;
#34450=CARTESIAN_POINT ( 'NONE',  ( -35.83891589277641287, -113.9929510916434339, 13.09299768411358400 ) ) ;
#34451=CARTESIAN_POINT ( 'NONE',  ( -35.69272627125608466, -115.9929510916434481, 13.01835785830562209 ) ) ;
#34460=CARTESIAN_POINT ( 'NONE',  ( -35.50000000000000711, -114.6807644833805000, -1.624782352598427959 ) ) ;
#34469=CARTESIAN_POINT ( 'NONE',  ( -34.50000000000000000, -117.0140978167138854, 0.6252176474015650465 ) ) ;
#34470=CARTESIAN_POINT ( 'NONE',  ( -35.00000000000000000, -114.0000000000000853, 2.000000000000001776 ) ) ;
#34473=CARTESIAN_POINT ( 'NONE',  ( -37.74901162816869515, -114.6652019342044042, 3.566024454178448710 ) ) ;
#34477=CARTESIAN_POINT ( 'NONE',  ( -35.50000000000000000, -114.6807644833805000, -0.6247823525984269599 ) ) ;
#34481=CARTESIAN_POINT ( 'NONE',  ( -37.18750000000006395, -114.9929510916434339, 13.11852480586264669 ) ) ;
#34484=CARTESIAN_POINT ( 'NONE',  ( -37.48437500000004263, -114.9929510916434339, 14.11852480586264846 ) ) ;
#34490=CARTESIAN_POINT ( 'NONE',  ( -35.50640865667917723, -115.9929510916434481, 12.69998175888958691 ) ) ;
#34491=CARTESIAN_POINT ( 'NONE',  ( -35.50000000000000711, -113.4307644833805000, -1.624782352598427959 ) ) ;
#34500=CARTESIAN_POINT ( 'NONE',  ( -35.97545270896702618, -113.6450488405582604, 7.409774454178449155 ) ) ;
#34509=CARTESIAN_POINT ( 'NONE',  ( -34.02454729103297382, -112.6980969099494132, 5.402725545821552622 ) ) ;
#34529=CARTESIAN_POINT ( 'NONE',  ( -34.50000000000000000, -115.9929510916434481, 11.38636890470581164 ) ) ;
#34533=CARTESIAN_POINT ( 'NONE',  ( -34.50000000000000000, -115.9929510916434481, 10.56126450660895699 ) ) ;
#34543=CARTESIAN_POINT ( 'NONE',  ( -33.97545270896703329, -115.1833782841879810, 7.090225545821551734 ) ) ;
#34546=CARTESIAN_POINT ( 'NONE',  ( -35.50000000000000711, -116.0140978167138712, 0.0002176474015577116276 ) ) ;
#34558=CARTESIAN_POINT ( 'NONE',  ( -35.00000000000000000, -113.9407375970686900, 8.496475545821551734 ) ) ;
#34565=CARTESIAN_POINT ( 'NONE',  ( -35.50000000000000000, -111.2666036476567655, -1.632210088999287212 ) ) ;
#34572=CARTESIAN_POINT ( 'NONE',  ( -34.50000000000000000, -114.9929510916434339, 10.52826033068511435 ) ) ;
#34574=CARTESIAN_POINT ( 'NONE',  ( -36.03125000000004263, -114.9929510916434339, 13.11852480586264669 ) ) ;
#34576=CARTESIAN_POINT ( 'NONE',  ( -34.50000000000000000, -114.0000000000003411, 9.500000000000035527 ) ) ;
#34579=CARTESIAN_POINT ( 'NONE',  ( -37.53269373325071712, -114.9929510916434339, 13.11752178341324360 ) ) ;
#34585=CARTESIAN_POINT ( 'NONE',  ( -35.50000000000000711, -114.9929510916434339, 10.72628538622835670 ) ) ;
#34587=CARTESIAN_POINT ( 'NONE',  ( -36.23083527818512550, -116.0245472910329880, 3.284774454178449155 ) ) ;
#34593=CARTESIAN_POINT ( 'NONE',  ( -34.50000000000000000, -113.0140978167143260, -0.6247823525984285142 ) ) ;
#34595=CARTESIAN_POINT ( 'NONE',  ( -36.23083527818512550, -116.0245472910329880, 7.784774454178451819 ) ) ;
#34601=CARTESIAN_POINT ( 'NONE',  ( -39.97545270896702618, -112.6980969099493990, 3.847274454178448710 ) ) ;
#34603=CARTESIAN_POINT ( 'NONE',  ( -35.50000000000000711, -115.1446187476384040, -1.616767172155725740 ) ) ;
#34607=SURFACE_SIDE_STYLE ('',( #23068 ) ) ;
#34612=CARTESIAN_POINT ( 'NONE',  ( -34.50000000000000000, -114.3474311500471430, -1.624782352598427959 ) ) ;
#34617=CARTESIAN_POINT ( 'NONE',  ( -34.50000000000000000, -113.9929510916434197, 10.50625754673586876 ) ) ;
#34620=CARTESIAN_POINT ( 'NONE',  ( -35.51597953369717686, -113.9929510916434339, 12.74811950270164473 ) ) ;
#34622=CARTESIAN_POINT ( 'NONE',  ( -38.00000000000000711, -115.9929510916434481, 12.56351784598954779 ) ) ;
#34633=CARTESIAN_POINT ( 'NONE',  ( -35.50000000000000711, -112.0140978167138712, -0.3122823525984337878 ) ) ;
#34638=FACE_OUTER_BOUND ( 'NONE', #25167, .T. ) ;
#34642=CARTESIAN_POINT ( 'NONE',  ( -34.50000000000000000, -113.0974311500471714, -2.624782352598442614 ) ) ;
#34647=CARTESIAN_POINT ( 'NONE',  ( -37.35495115944176092, -112.9754527089670688, 2.534774454178448710 ) ) ;
#34653=CARTESIAN_POINT ( 'NONE',  ( -34.50000000000000000, -113.7503824761461004, 0.9631051547057219997 ) ) ;
#34657=CARTESIAN_POINT ( 'NONE',  ( -35.50000000000000000, -113.8814751941377352, 10.49295109164313722 ) ) ;
#34660=CARTESIAN_POINT ( 'NONE',  ( -36.00976557831293690, -114.9929510916434339, 14.11852773550420359 ) ) ;
#34668=CARTESIAN_POINT ( 'NONE',  ( -35.50040135968784938, -115.9929510916434481, 12.63896776382214071 ) ) ;
#34679=CARTESIAN_POINT ( 'NONE',  ( -37.74901162816869515, -114.6652019342044042, 6.566024454178448266 ) ) ;
#34688=CARTESIAN_POINT ( 'NONE',  ( -37.05926240293131713, -111.0000000000000284, 8.121475545821549957 ) ) ;
#34705=FACE_OUTER_BOUND ( 'NONE', #13275, .T. ) ;
#34708=CARTESIAN_POINT ( 'NONE',  ( -34.50000000000000000, -115.9929510916434481, 12.26648026267477398 ) ) ;
#34710=CARTESIAN_POINT ( 'NONE',  ( -37.88768952767750164, -115.9754527089670262, 3.472274454178448266 ) ) ;
#34711=CARTESIAN_POINT ( 'NONE',  ( -34.50000000000000000, -115.9895221797699065, 10.38535157366622563 ) ) ;
#34722=CARTESIAN_POINT ( 'NONE',  ( -33.97545270896703329, -115.1833782841879810, 8.590225545821549957 ) ) ;
#34724=CARTESIAN_POINT ( 'NONE',  ( -35.50000000000000000, -113.0140978167138712, 0.7189676474015717078 ) ) ;
#34735=CARTESIAN_POINT ( 'NONE',  ( -39.02454729103295961, -113.2308352781851397, 9.340225545821551734 ) ) ;
#34740=CARTESIAN_POINT ( 'NONE',  ( -35.50000000000000711, -112.8356783780338759, 1.859636627348750348 ) ) ;
#34744=EDGE_LOOP ( 'NONE', ( #9164, #17925, #21347, #26006, #14646 ) ) ;
#34748=CARTESIAN_POINT ( 'NONE',  ( -34.50000000000000000, -114.9656200615856818, 10.26631071845107179 ) ) ;
#34751=CARTESIAN_POINT ( 'NONE',  ( -35.50640865667918433, -114.9929510916434339, 12.69998175888958514 ) ) ;
#34753=CARTESIAN_POINT ( 'NONE',  ( -34.50000000000000000, -114.0928965812550757, 9.511088712577292270 ) ) ;
#34755=CARTESIAN_POINT ( 'NONE',  ( -38.00000000000000711, -114.9929510916434339, 12.17846912687782179 ) ) ;
#34761=CARTESIAN_POINT ( 'NONE',  ( -37.62959469683911351, -114.9929510916434339, 13.10254527216511633 ) ) ;
#34764=CARTESIAN_POINT ( 'NONE',  ( -35.54388159064475872, -112.6276912846090568, 4.316024454178448266 ) ) ;
#34770=CARTESIAN_POINT ( 'NONE',  ( -34.50000000000000000, -113.0140978167138712, 0.7502176474015694874 ) ) ;
#34771=CARTESIAN_POINT ( 'NONE',  ( -34.97545270896703329, -113.2308352781851539, 8.909774454178450043 ) ) ;
#34772=ORIENTED_EDGE ( 'NONE', *, *, #2185, .T. ) ;
#34773=CARTESIAN_POINT ( 'NONE',  ( -39.97545270896702618, -112.6980969099493990, 2.347274454178448710 ) ) ;
#34785=CARTESIAN_POINT ( 'NONE',  ( -34.50000000000000000, -112.3697613878167658, -2.522673865603075605 ) ) ;
#34792=CARTESIAN_POINT ( 'NONE',  ( -34.50000000000000000, -113.9883062625807071, 10.50570311110699961 ) ) ;
#34797=CARTESIAN_POINT ( 'NONE',  ( -37.48437500000004263, -113.9929510916434339, 13.11852480586264846 ) ) ;
#34799=CARTESIAN_POINT ( 'NONE',  ( -37.50613590685470911, -115.9929510916434481, 13.11852378322482515 ) ) ;
#34812=CARTESIAN_POINT ( 'NONE',  ( -35.50000000000000711, -112.0651520602111191, -0.9469505670458575608 ) ) ;
#34820=CARTESIAN_POINT ( 'NONE',  ( -35.50000000000000000, -111.0140978167138570, -0.5622823525984297355 ) ) ;
#34824=CARTESIAN_POINT ( 'NONE',  ( -36.25098837183129774, -113.3347980657956242, 8.816024454178446490 ) ) ;
#34830=CARTESIAN_POINT ( 'NONE',  ( -35.50000000000000000, -115.0304602784513293, -0.6247823525985405357 ) ) ;
#34836=CARTESIAN_POINT ( 'NONE',  ( -37.56526046546250086, -114.9929510916434339, 13.11451721564129258 ) ) ;
#34840=CARTESIAN_POINT ( 'NONE',  ( -34.50000000000000000, -114.6807644833805000, -1.624782352598427959 ) ) ;
#34841=CARTESIAN_POINT ( 'NONE',  ( -37.42187499999997158, -114.9929510916434339, 14.11852480586264846 ) ) ;
#34847=CARTESIAN_POINT ( 'NONE',  ( -36.87500000000098765, -115.9929510916434481, 13.11852480586264846 ) ) ;
#34848=CARTESIAN_POINT ( 'NONE',  ( -35.50000000000000711, -112.7549084230351752, -1.592823285203595285 ) ) ;
#34861=CARTESIAN_POINT ( 'NONE',  ( -38.02454729103296671, -114.3549511594417396, 6.659774454178448266 ) ) ;
#34871=CARTESIAN_POINT ( 'NONE',  ( -37.88768952767750875, -112.0245472910329880, 3.527725545821551290 ) ) ;
#34884=ORIENTED_EDGE ( 'NONE', *, *, #8111, .T. ) ;
#34896=CARTESIAN_POINT ( 'NONE',  ( -34.50000000000000000, -115.9929510916434481, 12.57451923796416260 ) ) ;
#34898=CARTESIAN_POINT ( 'NONE',  ( -37.76916472181487450, -111.9754527089670404, 8.534774454178448266 ) ) ;
#34899=CARTESIAN_POINT ( 'NONE',  ( -34.50000000000000000, -115.9929510916434481, 10.51175824272318415 ) ) ;
#34909=CARTESIAN_POINT ( 'NONE',  ( -36.11231047232249125, -115.9754527089670262, 5.777725545821551734 ) ) ;
#34924=( BOUNDED_CURVE ( )  B_SPLINE_CURVE ( 2, ( #9323, #6971, #28411, #854, #11836, #22817, #9142, #20280, #31635, #1227, #23180, #17945, #1585, #12564, #23537, #30934, #12742, #26973, #18486, #2481, #23718, #34710, #35078, #21523, #31815, #20812, #10569, #2314, #26430, #32000, #10401, #29845, #7336, #7854, #21357, #7676, #32522, #29129, #2136, #32352, #9847, #5186, #13283, #16125, #18660, #26786, #18311, #13113, #27141, #10034, #13451, #24259, #20997, #35247, #29657, #24431, #15419, #4999, #15955, #18844, #24094, #7151, #4480, #18125, #1761, #21187, #29310, #4658, #15588, #26610, #29487, #1945, #12920, #23905, #32179, #34898, #10221, #7506, #4826, #15767, #30539 ),
 .UNSPECIFIED., .F., .T. ) 
 B_SPLINE_CURVE_WITH_KNOTS ( ( 3, 2, 2, 2, 2, 2, 2, 2, 2, 2, 2, 2, 2, 2, 2, 2, 2, 2, 2, 2, 2, 2, 2, 2, 2, 2, 2, 2, 2, 2, 2, 2, 2, 2, 2, 2, 2, 2, 2, 2, 3 ),
 ( 0.000000000000000000, 0.02500000000000000139, 0.05000000000000000278, 0.07499999999999999722, 0.1000000000000000056, 0.1250000000000000000, 0.1499999999999999944, 0.1749999999999999889, 0.2000000000000000111, 0.2250000000000000056, 0.2500000000000000000, 0.2750000000000000222, 0.2999999999999999889, 0.3250000000000000111, 0.3499999999999999778, 0.3750000000000000000, 0.4000000000000000222, 0.4249999999999999889, 0.4500000000000000111, 0.4749999999999999778, 0.5000000000000000000, 0.5250000000000000222, 0.5500000000000000444, 0.5749999999999999556, 0.5999999999999999778, 0.6250000000000000000, 0.6500000000000000222, 0.6750000000000000444, 0.6999999999999999556, 0.7249999999999999778, 0.7500000000000000000, 0.7750000000000000222, 0.8000000000000000444, 0.8249999999999999556, 0.8499999999999999778, 0.8750000000000000000, 0.9000000000000000222, 0.9250000000000000444, 0.9499999999999999556, 0.9749999999999999778, 1.000000000000000000 ),
 .UNSPECIFIED. ) 
 CURVE ( )  GEOMETRIC_REPRESENTATION_ITEM ( )  RATIONAL_B_SPLINE_CURVE ( ( 1.000000000000000000, 0.9238795325112867385, 1.000000000000000000, 0.9238795325112867385, 1.000000000000000000, 0.9238795325112867385, 1.000000000000000000, 0.9238795325112867385, 1.000000000000000000, 0.9238795325112867385, 1.000000000000000000, 0.9238795325112867385, 1.000000000000000000, 0.9238795325112867385, 1.000000000000000000, 0.9238795325112867385, 1.000000000000000000, 0.9238795325112867385, 1.000000000000000000, 0.9238795325112867385, 1.000000000000000000, 0.9238795325112867385, 1.000000000000000000, 0.9238795325112867385, 1.000000000000000000, 0.9238795325112867385, 1.000000000000000000, 0.9238795325112867385, 1.000000000000000000, 0.9238795325112867385, 1.000000000000000000, 0.9238795325112867385, 1.000000000000000000, 0.9238795325112867385, 1.000000000000000000, 0.9238795325112867385, 1.000000000000000000, 0.9238795325112867385, 1.000000000000000000, 0.9238795325112867385, 1.000000000000000000, 0.9238795325112867385, 1.000000000000000000, 0.9238795325112867385, 1.000000000000000000, 0.9238795325112867385, 1.000000000000000000, 0.9238795325112867385, 1.000000000000000000, 0.9238795325112867385, 1.000000000000000000, 0.9238795325112867385, 1.000000000000000000, 0.9238795325112867385, 1.000000000000000000, 0.9238795325112867385, 1.000000000000000000, 0.9238795325112867385, 1.000000000000000000, 0.9238795325112867385, 1.000000000000000000, 0.9238795325112867385, 1.000000000000000000, 0.9238795325112867385, 1.000000000000000000, 0.9238795325112867385, 1.000000000000000000, 0.9238795325112867385, 1.000000000000000000, 0.9238795325112867385, 1.000000000000000000, 0.9238795325112867385, 1.000000000000000000, 0.9238795325112867385, 1.000000000000000000, 0.9238795325112867385, 1.000000000000000000, 0.9238795325112867385, 1.000000000000000000, 0.9238795325112867385, 1.000000000000000000 ) ) 
 REPRESENTATION_ITEM ( '' )  );
#34925=CARTESIAN_POINT ( 'NONE',  ( -38.37230871539094323, -115.4561184093552413, 9.058975545821551734 ) ) ;
#34931=CARTESIAN_POINT ( 'NONE',  ( -35.50000000000000711, -112.4434344552011282, 1.705278471174987986 ) ) ;
#34938=CARTESIAN_POINT ( 'NONE',  ( -34.50000000000000000, -112.3465879560236687, 1.629585756119413364 ) ) ;
#34940=CARTESIAN_POINT ( 'NONE',  ( -34.50000000000000000, -114.9929510916434339, 12.26648026267477221 ) ) ;
#34944=CARTESIAN_POINT ( 'NONE',  ( -37.54084996655477369, -114.9929510916434339, 13.11692036158760466 ) ) ;
#34946=CARTESIAN_POINT ( 'NONE',  ( -34.50000000000000000, -114.9902084924877954, 10.43071793783961176 ) ) ;
#34949=CARTESIAN_POINT ( 'NONE',  ( -38.00000068757622529, -114.9929510916434339, 12.61439929482944855 ) ) ;
#34955=CARTESIAN_POINT ( 'NONE',  ( -37.51635661748575501, -114.9929510916434339, 13.11827392651459157 ) ) ;
#34957=CARTESIAN_POINT ( 'NONE',  ( -37.88768952767750164, -115.9754527089670262, 7.972274454178450043 ) ) ;
#34965=CARTESIAN_POINT ( 'NONE',  ( -34.92058450342251064, -116.1632251905417945, 1.691024454178448932 ) ) ;
#34970=CARTESIAN_POINT ( 'NONE',  ( -35.50000000000000711, -116.0140978167138712, 0.0002176474015577116276 ) ) ;
#34978=CARTESIAN_POINT ( 'NONE',  ( -34.50000000000000000, -113.4307644833805142, -2.624782352598442614 ) ) ;
#34985=CARTESIAN_POINT ( 'NONE',  ( -34.50000000000000000, -113.9929510916435049, 10.50625754673586876 ) ) ;
#34988=CARTESIAN_POINT ( 'NONE',  ( -34.50000000000000000, -113.9883062625807071, 10.50570311110699961 ) ) ;
#34990=CARTESIAN_POINT ( 'NONE',  ( -35.98364338251434447, -115.9929510916434481, 13.11827392651456314 ) ) ;
#35002=CARTESIAN_POINT ( 'NONE',  ( -35.50000000000000711, -112.0140978167138712, 0.2502176474015765373 ) ) ;
#35004=CARTESIAN_POINT ( 'NONE',  ( -35.50000000000000711, -114.9819937217110635, 10.35556074009299188 ) ) ;
#35009=CARTESIAN_POINT ( 'NONE',  ( -35.50000000000000000, -113.2224311500466030, -2.624782352598442614 ) ) ;
#35013=CARTESIAN_POINT ( 'NONE',  ( -36.33479806579561000, -114.7490116281687165, 7.691024454178450043 ) ) ;
#35022=CARTESIAN_POINT ( 'NONE',  ( -34.50000000000000000, -113.0140978167156902, -0.6247823525984268489 ) ) ;
#35027=CARTESIAN_POINT ( 'NONE',  ( -38.00000000000000711, -114.9929510916434339, 12.56351784598954779 ) ) ;
#35030=CARTESIAN_POINT ( 'NONE',  ( -34.50000000000000000, -112.0157046079661995, -0.6902086197697556713 ) ) ;
#35036=CARTESIAN_POINT ( 'NONE',  ( -35.50000000000000000, -115.9929510916434481, 12.26648026267477398 ) ) ;
#35037=CARTESIAN_POINT ( 'NONE',  ( -35.50000000000000711, -116.0124910254613297, -0.6902086197697608894 ) ) ;
#35059=CARTESIAN_POINT ( 'NONE',  ( -35.54388159064475872, -115.3723087153909432, 4.183975545821551734 ) ) ;
#35078=CARTESIAN_POINT ( 'NONE',  ( -38.45611840935523418, -115.3723087153909432, 3.566024454178448710 ) ) ;
#35079=CARTESIAN_POINT ( 'NONE',  ( -34.50000000000000000, -115.9929510916434481, 11.73841344789270202 ) ) ;
#35089=CARTESIAN_POINT ( 'NONE',  ( -38.97545270896704039, -114.8876895276775087, 3.152725545821551290 ) ) ;
#35104=CARTESIAN_POINT ( 'NONE',  ( -36.94073759706868287, -115.9999999999999858, 8.871475545821551734 ) ) ;
#35109=CARTESIAN_POINT ( 'NONE',  ( -35.50000000000000711, -112.7765286249690035, 1.847058736912741583 ) ) ;
#35116=CARTESIAN_POINT ( 'NONE',  ( -34.50000000000000000, -112.0209493036498287, 0.9959249592223760050 ) ) ;
#35117=CARTESIAN_POINT ( 'NONE',  ( -34.50000000000000000, -114.9928438774171582, 10.49113435197128652 ) ) ;
#35119=CARTESIAN_POINT ( 'NONE',  ( -35.87040530316090070, -114.9929510916434339, 13.10254527216545917 ) ) ;
#35122=CARTESIAN_POINT ( 'NONE',  ( -34.50000000000000000, -114.9929510916434339, 10.51175824272318415 ) ) ;
#35132=CARTESIAN_POINT ( 'NONE',  ( -36.03906250000000000, -114.9929510916434339, 13.11852480586264669 ) ) ;
#35134=CARTESIAN_POINT ( 'NONE',  ( -35.62769128460905677, -115.4561184093552413, 4.691024454178448266 ) ) ;
#35141=CARTESIAN_POINT ( 'NONE',  ( -38.30190309005061522, -116.9754527089670546, 4.972274454178449155 ) ) ;
#35154=CARTESIAN_POINT ( 'NONE',  ( -34.50000000000000000, -111.0301281775997353, -0.8858242144478579716 ) ) ;
#35158=CARTESIAN_POINT ( 'NONE',  ( -35.50000000000000711, -114.1021862393805577, 9.512197583835053649 ) ) ;
#35159=CARTESIAN_POINT ( 'NONE',  ( -34.50000000000000000, -113.9929510916433912, 10.50625754673588474 ) ) ;
#35162=CARTESIAN_POINT ( 'NONE',  ( -37.42187499999996447, -113.9929510916434339, 13.11852480586264846 ) ) ;
#35163=CARTESIAN_POINT ( 'NONE',  ( -37.99599240977853754, -115.9929510916434481, 12.68378527132499656 ) ) ;
#35177=CARTESIAN_POINT ( 'NONE',  ( -35.50000000000000000, -113.0140978167134449, 0.8752176474011410523 ) ) ;
#35180=CARTESIAN_POINT ( 'NONE',  ( -35.50000000000000711, -114.9929510916434339, 10.85830208992344303 ) ) ;
#35184=CARTESIAN_POINT ( 'NONE',  ( -35.50000000000000000, -111.0140978167138570, 0.6252176474015680441 ) ) ;
#35188=CARTESIAN_POINT ( 'NONE',  ( -37.97545270896701908, -113.5265240346955977, 6.847274454178448266 ) ) ;
#35192=CARTESIAN_POINT ( 'NONE',  ( -34.50000000000000000, -113.3474311500483935, -0.6247823525984269599 ) ) ;
#35197=CARTESIAN_POINT ( 'NONE',  ( -38.00000000000000711, -114.9929510916434339, 12.57451923796417503 ) ) ;
#35200=CARTESIAN_POINT ( 'NONE',  ( -34.50000000000000000, -112.3995503592287690, -1.424448457485529618 ) ) ;
#35207=CARTESIAN_POINT ( 'NONE',  ( -37.99359134332094357, -115.9929510916434481, 12.69998175888958514 ) ) ;
#35219=AXIS2_PLACEMENT_3D ( 'NONE', #26187, #4067, #30880 ) ;
#35229=CARTESIAN_POINT ( 'NONE',  ( -36.94073759706868287, -115.9999999999999858, 4.371475545821550845 ) ) ;
#35247=CARTESIAN_POINT ( 'NONE',  ( -37.88768952767750164, -115.9754527089670262, 6.472274454178449155 ) ) ;
#35249=CARTESIAN_POINT ( 'NONE',  ( -34.50000000000000000, -115.9929510916434481, 10.61627146648203990 ) ) ;
#35260=CARTESIAN_POINT ( 'NONE',  ( -37.05926240293131713, -111.0000000000000284, 9.621475545821549957 ) ) ;
#35282=CARTESIAN_POINT ( 'NONE',  ( -35.50000000000000711, -112.5103839485166333, -1.498529437127682495 ) ) ;
#35289=CARTESIAN_POINT ( 'NONE',  ( -34.50000000000000000, -114.6807644833805000, -1.624782352598427959 ) ) ;
#35291=CARTESIAN_POINT ( 'NONE',  ( -37.54906985245724371, -114.9929510916434339, 14.11777216781844579 ) ) ;
#35295=CARTESIAN_POINT ( 'NONE',  ( -38.00000000000000711, -114.9929510916434339, 10.50625754673587231 ) ) ;
#35298=CARTESIAN_POINT ( 'NONE',  ( -34.50000000000000000, -114.9927795562974069, 10.48735431211914815 ) ) ;
#35300=CARTESIAN_POINT ( 'NONE',  ( -38.00000000000000711, -114.9929510916434339, 12.60752341388803721 ) ) ;
#35306=CARTESIAN_POINT ( 'NONE',  ( -37.89983305244309975, -114.9929510916434339, 12.92579853460519246 ) ) ;
#35308=CARTESIAN_POINT ( 'NONE',  ( -37.05926240293131713, -115.9999999999999858, 6.378524454178448266 ) ) ;
#35316=CARTESIAN_POINT ( 'NONE',  ( -36.94073759706866156, -111.0000000000000284, 4.128524454178449155 ) ) ;
#35319=CARTESIAN_POINT ( 'NONE',  ( -35.50000000000000711, -116.0140978167138712, -0.3122823525984417259 ) ) ;
#35328=CARTESIAN_POINT ( 'NONE',  ( -34.50000000000000000, -111.0140978167138570, 0.3752176474015639918 ) ) ;
#35332=CARTESIAN_POINT ( 'NONE',  ( -35.50000000000000711, -114.9656200615856818, 10.26631071845107179 ) ) ;
#35333=CARTESIAN_POINT ( 'NONE',  ( -34.50000000000000000, -113.9929510916434339, 10.50625754673588474 ) ) ;
#35336=CARTESIAN_POINT ( 'NONE',  ( -34.50000000000000000, -113.9000545103886850, 10.49516883415891577 ) ) ;
#35337=CARTESIAN_POINT ( 'NONE',  ( -37.46093750000000711, -115.9929510916434481, 13.11852480586264846 ) ) ;
#35348=CARTESIAN_POINT ( 'NONE',  ( -35.50000000000000711, -116.0140978167138712, 0.6252176474015648244 ) ) ;
#35350=CARTESIAN_POINT ( 'NONE',  ( -35.50000000000000711, -114.9929510916434339, 10.94631322572069365 ) ) ;
#35354=CARTESIAN_POINT ( 'NONE',  ( -35.50000000000000000, -111.0140978167138570, -0.4997823525984338988 ) ) ;
#35357=CARTESIAN_POINT ( 'NONE',  ( -35.00000000000000000, -114.0592624029313242, 3.003524454178448710 ) ) ;
#35362=CARTESIAN_POINT ( 'NONE',  ( -34.50000000000000000, -113.0140978167138712, 0.8752176474015154195 ) ) ;
#35370=CARTESIAN_POINT ( 'NONE',  ( -38.00000000000000711, -114.9929510916434339, 12.50851088611646311 ) ) ;
#35373=CARTESIAN_POINT ( 'NONE',  ( -34.50000000000000000, -112.0140978167138712, -0.4997823525984337878 ) ) ;
#35378=CARTESIAN_POINT ( 'NONE',  ( -37.99994980024369085, -115.9929510916434481, 12.62670525340494621 ) ) ;
#35400=CARTESIAN_POINT ( 'NONE',  ( -38.45611840935523418, -112.6276912846090568, 4.933975545821551734 ) ) ;
#35420=CARTESIAN_POINT ( 'NONE',  ( -37.62254989966453422, -115.9929510916434481, 14.11371147303758278 ) ) ;
#35429=CARTESIAN_POINT ( 'NONE',  ( -36.94073759706868287, -115.9999999999999858, 4.371475545821550845 ) ) ;
#35460=CARTESIAN_POINT ( 'NONE',  ( -34.50000000000000000, -113.8474311500459777, -1.624782352598427959 ) ) ;
#35461=CARTESIAN_POINT ( 'NONE',  ( -38.98797722933582577, -114.9929510916434339, 12.81430620224974959 ) ) ;
#35464=CARTESIAN_POINT ( 'NONE',  ( -35.50000000000000000, -113.9000545103886850, 10.49516883415891577 ) ) ;
#35466=CARTESIAN_POINT ( 'NONE',  ( -37.46093750000000711, -114.9929510916434339, 14.11852480586264846 ) ) ;
#35474=VERTEX_POINT ( 'NONE', #16725 ) ;
#35476=CARTESIAN_POINT ( 'NONE',  ( -35.99386409314529800, -114.9929510916434339, 13.11852378322482515 ) ) ;
#35478=CARTESIAN_POINT ( 'NONE',  ( -37.88768952767750164, -115.9754527089670262, 4.972274454178448266 ) ) ;
#35489=CARTESIAN_POINT ( 'NONE',  ( -33.97545270896703329, -115.1833782841879810, 2.590225545821551734 ) ) ;
#35502=CARTESIAN_POINT ( 'NONE',  ( -34.50000000000000000, -113.3474311500483935, -2.624782352598442614 ) ) ;
#35510=CARTESIAN_POINT ( 'NONE',  ( -36.01562499999997158, -113.9929510916434339, 14.11852480586265024 ) ) ;
#35513=CARTESIAN_POINT ( 'NONE',  ( -38.00000000000000711, -113.9929510916434339, 12.50851088611646311 ) ) ;
#35514=CARTESIAN_POINT ( 'NONE',  ( -35.50000000000000711, -114.3464919575557843, 9.568884482464163455 ) ) ;
#35530=CARTESIAN_POINT ( 'NONE',  ( -35.50000000000000711, -116.0124910254613297, -0.6902086197697608894 ) ) ;
#35533=CARTESIAN_POINT ( 'NONE',  ( -36.25098837183129774, -113.3347980657956242, 5.816024454178450043 ) ) ;
#35535=CARTESIAN_POINT ( 'NONE',  ( -35.50000000000000711, -114.9929510916434339, 12.57451923796416082 ) ) ;
#35539=CARTESIAN_POINT ( 'NONE',  ( -35.50000000000000000, -113.0765974847181781, -2.624803185604914102 ) ) ;
#35543=CARTESIAN_POINT ( 'NONE',  ( -36.23083527818512550, -116.0245472910329880, 3.284774454178449155 ) ) ;
#35549=CARTESIAN_POINT ( 'NONE',  ( -34.50000000000000000, -115.0140978167138712, -0.6247823525985405357 ) ) ;
#35557=CARTESIAN_POINT ( 'NONE',  ( -35.50000000000000000, -113.9929510916434339, 12.60752341388803721 ) ) ;
#35561=CARTESIAN_POINT ( 'NONE',  ( -34.50000000000000000, -112.0140978167138712, 0.5627176474015717078 ) ) ;
#35562=CARTESIAN_POINT ( 'NONE',  ( -35.51674767832922441, -115.9929510916434481, 14.04194344061634325 ) ) ;
#35566=CARTESIAN_POINT ( 'NONE',  ( -37.80727372874345349, -115.9929510916434481, 13.01835785830664705 ) ) ;
#35588=CARTESIAN_POINT ( 'NONE',  ( -38.97545270896704039, -114.8876895276775087, 9.152725545821555286 ) ) ;
#35602=CARTESIAN_POINT ( 'NONE',  ( -38.98797722933581866, -115.9929510916434481, 12.81430620224974959 ) ) ;
#35611=CARTESIAN_POINT ( 'NONE',  ( -37.35495115944176803, -115.0245472910329880, 4.465225545821550845 ) ) ;
ENDSEC;
END-ISO-10303-21;
